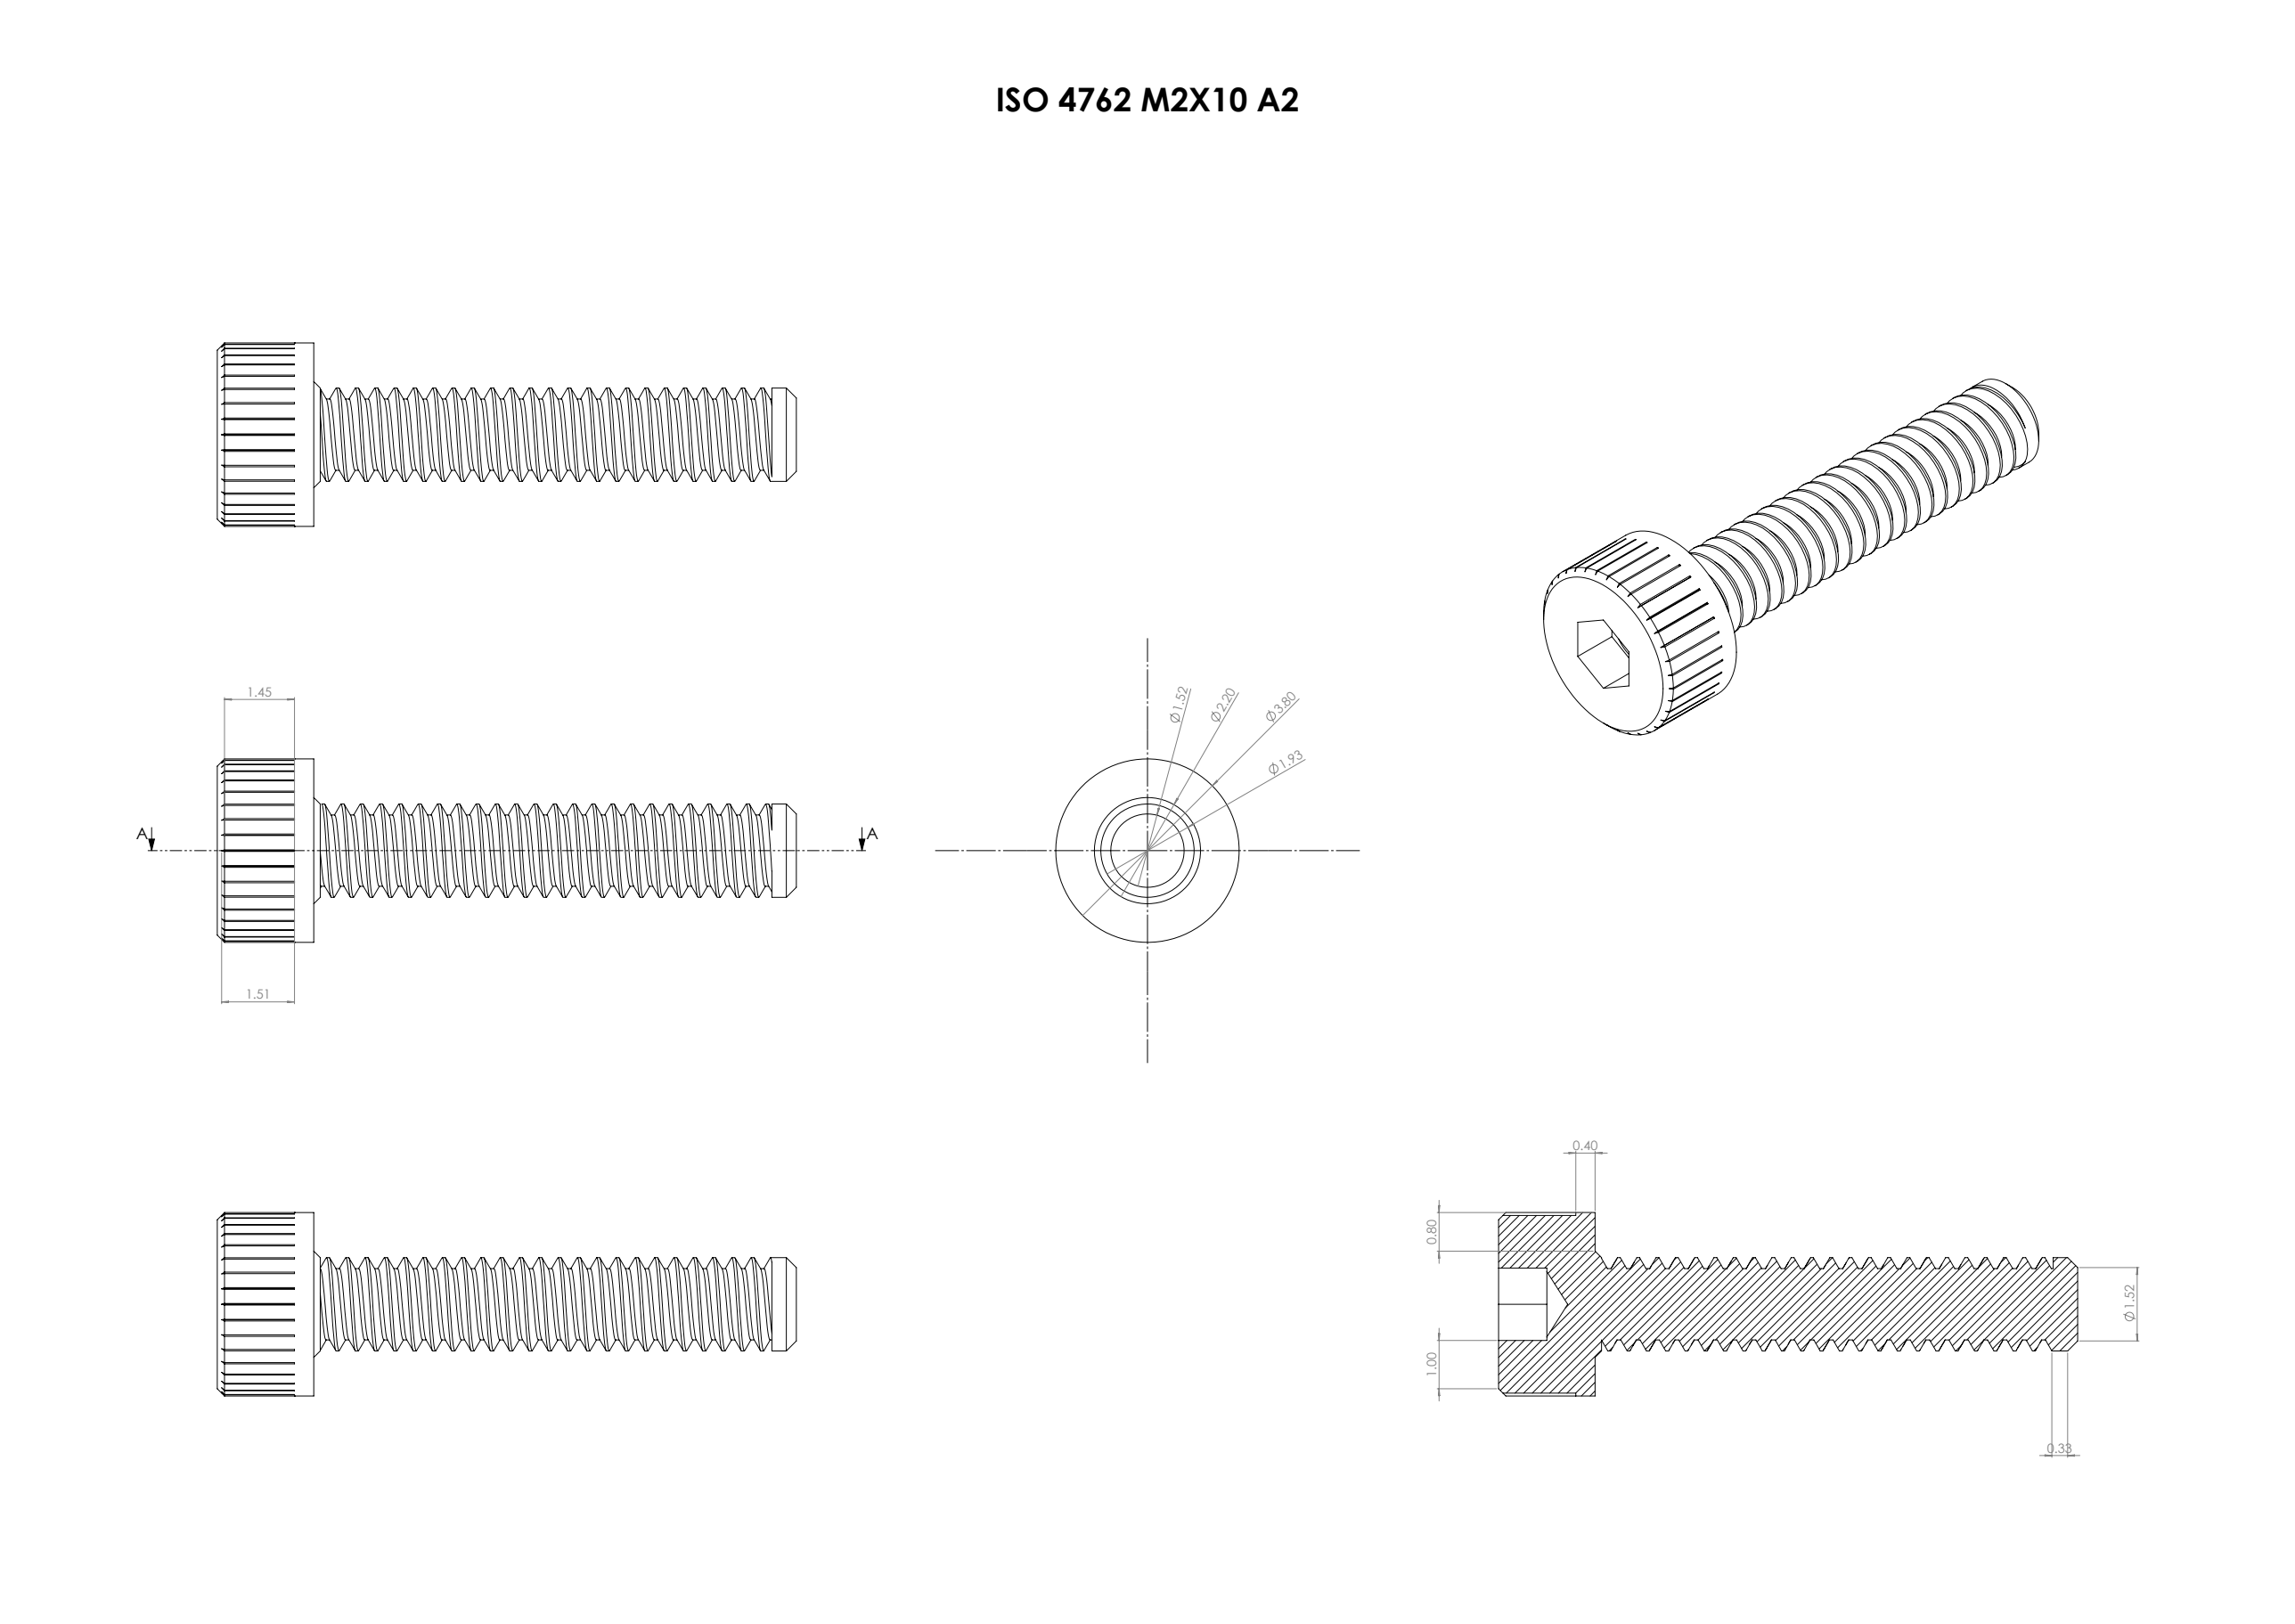
ISO-10303-21;
HEADER;
/* Generated by software containing ST-Developer
 * from STEP Tools, Inc. (www.steptools.com) 
 */

FILE_DESCRIPTION(
/* description */ (''),
/* implementation_level */ '2;1');

FILE_NAME(
/* name */ '16_ISO_4762_M2x10_A2.step',
/* time_stamp */ '2026-10-19T23:00:43-07:00',
/* author */ (''),
/* organization */ (''),
/* preprocessor_version */ 'ST-DEVELOPER v20.2',
/* originating_system */ 'Autodesk Translation Framework v15.15.0.0',
/* authorisation */ '');

FILE_SCHEMA (('AUTOMOTIVE_DESIGN { 1 0 10303 214 3 1 1 }'));
ENDSEC;

DATA;
#10=MECHANICAL_DESIGN_GEOMETRIC_PRESENTATION_REPRESENTATION('',(#1012),#55002);
#323=(
BOUNDED_CURVE()
B_SPLINE_CURVE(2,(#47824,#47825,#47826),.UNSPECIFIED.,.F.,.F.)
B_SPLINE_CURVE_WITH_KNOTS((3,3),(0.,0.00841282944278042),.UNSPECIFIED.)
CURVE()
GEOMETRIC_REPRESENTATION_ITEM()
RATIONAL_B_SPLINE_CURVE((1.,1.00035365746955,1.00043184882983))
REPRESENTATION_ITEM('')
);
#324=(
BOUNDED_CURVE()
B_SPLINE_CURVE(2,(#47830,#47831,#47832),.UNSPECIFIED.,.F.,.F.)
B_SPLINE_CURVE_WITH_KNOTS((3,3),(0.0131888113576721,0.0216016408002996),
 .UNSPECIFIED.)
CURVE()
GEOMETRIC_REPRESENTATION_ITEM()
RATIONAL_B_SPLINE_CURVE((1.00043184882948,1.00035365746926,1.))
REPRESENTATION_ITEM('')
);
#325=(
BOUNDED_CURVE()
B_SPLINE_CURVE(2,(#47845,#47846,#47847),.UNSPECIFIED.,.F.,.F.)
B_SPLINE_CURVE_WITH_KNOTS((3,3),(0.,0.0084128294426201),.UNSPECIFIED.)
CURVE()
GEOMETRIC_REPRESENTATION_ITEM()
RATIONAL_B_SPLINE_CURVE((1.,1.00035365746986,1.00043184883023))
REPRESENTATION_ITEM('')
);
#326=(
BOUNDED_CURVE()
B_SPLINE_CURVE(2,(#47851,#47852,#47853),.UNSPECIFIED.,.F.,.F.)
B_SPLINE_CURVE_WITH_KNOTS((3,3),(0.0131888113575809,0.0216016408002996),
 .UNSPECIFIED.)
CURVE()
GEOMETRIC_REPRESENTATION_ITEM()
RATIONAL_B_SPLINE_CURVE((1.00043184883059,1.00035365747017,1.))
REPRESENTATION_ITEM('')
);
#327=(
BOUNDED_CURVE()
B_SPLINE_CURVE(2,(#47866,#47867,#47868),.UNSPECIFIED.,.F.,.F.)
B_SPLINE_CURVE_WITH_KNOTS((3,3),(0.,0.00841282944278058),.UNSPECIFIED.)
CURVE()
GEOMETRIC_REPRESENTATION_ITEM()
RATIONAL_B_SPLINE_CURVE((1.,1.00035365746906,1.00043184882924))
REPRESENTATION_ITEM('')
);
#328=(
BOUNDED_CURVE()
B_SPLINE_CURVE(2,(#47872,#47873,#47874),.UNSPECIFIED.,.F.,.F.)
B_SPLINE_CURVE_WITH_KNOTS((3,3),(0.0131888113576548,0.0216016408002996),
 .UNSPECIFIED.)
CURVE()
GEOMETRIC_REPRESENTATION_ITEM()
RATIONAL_B_SPLINE_CURVE((1.00043184882846,1.00035365746842,1.))
REPRESENTATION_ITEM('')
);
#329=(
BOUNDED_CURVE()
B_SPLINE_CURVE(2,(#47887,#47888,#47889),.UNSPECIFIED.,.F.,.F.)
B_SPLINE_CURVE_WITH_KNOTS((3,3),(0.,0.00841282944280584),.UNSPECIFIED.)
CURVE()
GEOMETRIC_REPRESENTATION_ITEM()
RATIONAL_B_SPLINE_CURVE((1.,1.00035365746775,1.00043184882763))
REPRESENTATION_ITEM('')
);
#330=(
BOUNDED_CURVE()
B_SPLINE_CURVE(2,(#47893,#47894,#47895),.UNSPECIFIED.,.F.,.F.)
B_SPLINE_CURVE_WITH_KNOTS((3,3),(0.0131888113576015,0.0216016408002996),
 .UNSPECIFIED.)
CURVE()
GEOMETRIC_REPRESENTATION_ITEM()
RATIONAL_B_SPLINE_CURVE((1.00043184882681,1.00035365746707,1.))
REPRESENTATION_ITEM('')
);
#331=(
BOUNDED_CURVE()
B_SPLINE_CURVE(2,(#47908,#47909,#47910),.UNSPECIFIED.,.F.,.F.)
B_SPLINE_CURVE_WITH_KNOTS((3,3),(0.,0.00841282944278488),.UNSPECIFIED.)
CURVE()
GEOMETRIC_REPRESENTATION_ITEM()
RATIONAL_B_SPLINE_CURVE((1.,1.0003536574676,1.00043184882745))
REPRESENTATION_ITEM('')
);
#332=(
BOUNDED_CURVE()
B_SPLINE_CURVE(2,(#47914,#47915,#47916),.UNSPECIFIED.,.F.,.F.)
B_SPLINE_CURVE_WITH_KNOTS((3,3),(0.0131888113575949,0.0216016408002996),
 .UNSPECIFIED.)
CURVE()
GEOMETRIC_REPRESENTATION_ITEM()
RATIONAL_B_SPLINE_CURVE((1.000431848828,1.00035365746804,1.))
REPRESENTATION_ITEM('')
);
#333=(
BOUNDED_CURVE()
B_SPLINE_CURVE(2,(#47929,#47930,#47931),.UNSPECIFIED.,.F.,.F.)
B_SPLINE_CURVE_WITH_KNOTS((3,3),(0.,0.00841282944265237),.UNSPECIFIED.)
CURVE()
GEOMETRIC_REPRESENTATION_ITEM()
RATIONAL_B_SPLINE_CURVE((1.,1.00035365746874,1.00043184882885))
REPRESENTATION_ITEM('')
);
#334=(
BOUNDED_CURVE()
B_SPLINE_CURVE(2,(#47935,#47936,#47937),.UNSPECIFIED.,.F.,.F.)
B_SPLINE_CURVE_WITH_KNOTS((3,3),(0.0131888113575151,0.0216016408002996),
 .UNSPECIFIED.)
CURVE()
GEOMETRIC_REPRESENTATION_ITEM()
RATIONAL_B_SPLINE_CURVE((1.00043184882745,1.0003536574676,1.))
REPRESENTATION_ITEM('')
);
#335=(
BOUNDED_CURVE()
B_SPLINE_CURVE(2,(#47950,#47951,#47952),.UNSPECIFIED.,.F.,.F.)
B_SPLINE_CURVE_WITH_KNOTS((3,3),(0.,0.00841282944265245),.UNSPECIFIED.)
CURVE()
GEOMETRIC_REPRESENTATION_ITEM()
RATIONAL_B_SPLINE_CURVE((1.,1.00035365746621,1.00043184882576))
REPRESENTATION_ITEM('')
);
#336=(
BOUNDED_CURVE()
B_SPLINE_CURVE(2,(#47956,#47957,#47958),.UNSPECIFIED.,.F.,.F.)
B_SPLINE_CURVE_WITH_KNOTS((3,3),(0.013188811357676,0.0216016408002996),
 .UNSPECIFIED.)
CURVE()
GEOMETRIC_REPRESENTATION_ITEM()
RATIONAL_B_SPLINE_CURVE((1.00043184882966,1.0003536574694,1.))
REPRESENTATION_ITEM('')
);
#337=(
BOUNDED_CURVE()
B_SPLINE_CURVE(2,(#47971,#47972,#47973),.UNSPECIFIED.,.F.,.F.)
B_SPLINE_CURVE_WITH_KNOTS((3,3),(0.,0.00841282944263587),.UNSPECIFIED.)
CURVE()
GEOMETRIC_REPRESENTATION_ITEM()
RATIONAL_B_SPLINE_CURVE((1.,1.00035365746699,1.00043184882672))
REPRESENTATION_ITEM('')
);
#338=(
BOUNDED_CURVE()
B_SPLINE_CURVE(2,(#47977,#47978,#47979),.UNSPECIFIED.,.F.,.F.)
B_SPLINE_CURVE_WITH_KNOTS((3,3),(0.0131888113575321,0.0216016408002996),
 .UNSPECIFIED.)
CURVE()
GEOMETRIC_REPRESENTATION_ITEM()
RATIONAL_B_SPLINE_CURVE((1.00043184883015,1.00035365746981,1.))
REPRESENTATION_ITEM('')
);
#339=(
BOUNDED_CURVE()
B_SPLINE_CURVE(2,(#47992,#47993,#47994),.UNSPECIFIED.,.F.,.F.)
B_SPLINE_CURVE_WITH_KNOTS((3,3),(0.,0.00841282944268715),.UNSPECIFIED.)
CURVE()
GEOMETRIC_REPRESENTATION_ITEM()
RATIONAL_B_SPLINE_CURVE((1.,1.00035365746714,1.0004318488269))
REPRESENTATION_ITEM('')
);
#340=(
BOUNDED_CURVE()
B_SPLINE_CURVE(2,(#47998,#47999,#48000),.UNSPECIFIED.,.F.,.F.)
B_SPLINE_CURVE_WITH_KNOTS((3,3),(0.0131888113576173,0.0216016408002996),
 .UNSPECIFIED.)
CURVE()
GEOMETRIC_REPRESENTATION_ITEM()
RATIONAL_B_SPLINE_CURVE((1.00043184882651,1.00035365746683,1.))
REPRESENTATION_ITEM('')
);
#341=(
BOUNDED_CURVE()
B_SPLINE_CURVE(2,(#48013,#48014,#48015),.UNSPECIFIED.,.F.,.F.)
B_SPLINE_CURVE_WITH_KNOTS((3,3),(0.,0.00841282944268232),.UNSPECIFIED.)
CURVE()
GEOMETRIC_REPRESENTATION_ITEM()
RATIONAL_B_SPLINE_CURVE((1.,1.00035365746714,1.0004318488269))
REPRESENTATION_ITEM('')
);
#342=(
BOUNDED_CURVE()
B_SPLINE_CURVE(2,(#48019,#48020,#48021),.UNSPECIFIED.,.F.,.F.)
B_SPLINE_CURVE_WITH_KNOTS((3,3),(0.0131888113576523,0.0216016408002997),
 .UNSPECIFIED.)
CURVE()
GEOMETRIC_REPRESENTATION_ITEM()
RATIONAL_B_SPLINE_CURVE((1.00043184882641,1.00035365746674,1.))
REPRESENTATION_ITEM('')
);
#343=(
BOUNDED_CURVE()
B_SPLINE_CURVE(2,(#48034,#48035,#48036),.UNSPECIFIED.,.F.,.F.)
B_SPLINE_CURVE_WITH_KNOTS((3,3),(0.,0.00841282944262782),.UNSPECIFIED.)
CURVE()
GEOMETRIC_REPRESENTATION_ITEM()
RATIONAL_B_SPLINE_CURVE((1.,1.00035365747069,1.00043184883123))
REPRESENTATION_ITEM('')
);
#344=(
BOUNDED_CURVE()
B_SPLINE_CURVE(2,(#48040,#48041,#48042),.UNSPECIFIED.,.F.,.F.)
B_SPLINE_CURVE_WITH_KNOTS((3,3),(0.0131888113575803,0.0216016408002996),
 .UNSPECIFIED.)
CURVE()
GEOMETRIC_REPRESENTATION_ITEM()
RATIONAL_B_SPLINE_CURVE((1.00043184883154,1.00035365747094,1.))
REPRESENTATION_ITEM('')
);
#345=(
BOUNDED_CURVE()
B_SPLINE_CURVE(2,(#48055,#48056,#48057),.UNSPECIFIED.,.F.,.F.)
B_SPLINE_CURVE_WITH_KNOTS((3,3),(0.,0.00841282944278058),.UNSPECIFIED.)
CURVE()
GEOMETRIC_REPRESENTATION_ITEM()
RATIONAL_B_SPLINE_CURVE((1.,1.00035365746906,1.00043184882924))
REPRESENTATION_ITEM('')
);
#346=(
BOUNDED_CURVE()
B_SPLINE_CURVE(2,(#48061,#48062,#48063),.UNSPECIFIED.,.F.,.F.)
B_SPLINE_CURVE_WITH_KNOTS((3,3),(0.0131888113576548,0.0216016408002996),
 .UNSPECIFIED.)
CURVE()
GEOMETRIC_REPRESENTATION_ITEM()
RATIONAL_B_SPLINE_CURVE((1.00043184882846,1.00035365746842,1.))
REPRESENTATION_ITEM('')
);
#347=(
BOUNDED_CURVE()
B_SPLINE_CURVE(2,(#48076,#48077,#48078),.UNSPECIFIED.,.F.,.F.)
B_SPLINE_CURVE_WITH_KNOTS((3,3),(0.,0.00841282944280138),.UNSPECIFIED.)
CURVE()
GEOMETRIC_REPRESENTATION_ITEM()
RATIONAL_B_SPLINE_CURVE((1.,1.00035365746471,1.00043184882392))
REPRESENTATION_ITEM('')
);
#348=(
BOUNDED_CURVE()
B_SPLINE_CURVE(2,(#48082,#48083,#48084),.UNSPECIFIED.,.F.,.F.)
B_SPLINE_CURVE_WITH_KNOTS((3,3),(0.0131888113575931,0.0216016408002996),
 .UNSPECIFIED.)
CURVE()
GEOMETRIC_REPRESENTATION_ITEM()
RATIONAL_B_SPLINE_CURVE((1.00043184882494,1.00035365746554,1.))
REPRESENTATION_ITEM('')
);
#349=(
BOUNDED_CURVE()
B_SPLINE_CURVE(2,(#48097,#48098,#48099),.UNSPECIFIED.,.F.,.F.)
B_SPLINE_CURVE_WITH_KNOTS((3,3),(0.,0.00841282944261464),.UNSPECIFIED.)
CURVE()
GEOMETRIC_REPRESENTATION_ITEM()
RATIONAL_B_SPLINE_CURVE((1.,1.00035365746679,1.00043184882648))
REPRESENTATION_ITEM('')
);
#350=(
BOUNDED_CURVE()
B_SPLINE_CURVE(2,(#48103,#48104,#48105),.UNSPECIFIED.,.F.,.F.)
B_SPLINE_CURVE_WITH_KNOTS((3,3),(0.0131888113575887,0.0216016408002996),
 .UNSPECIFIED.)
CURVE()
GEOMETRIC_REPRESENTATION_ITEM()
RATIONAL_B_SPLINE_CURVE((1.00043184882758,1.0003536574677,1.))
REPRESENTATION_ITEM('')
);
#351=(
BOUNDED_CURVE()
B_SPLINE_CURVE(2,(#48118,#48119,#48120),.UNSPECIFIED.,.F.,.F.)
B_SPLINE_CURVE_WITH_KNOTS((3,3),(0.,0.00841282944265251),.UNSPECIFIED.)
CURVE()
GEOMETRIC_REPRESENTATION_ITEM()
RATIONAL_B_SPLINE_CURVE((1.,1.00035365746762,1.00043184882748))
REPRESENTATION_ITEM('')
);
#352=(
BOUNDED_CURVE()
B_SPLINE_CURVE(2,(#48124,#48125,#48126),.UNSPECIFIED.,.F.,.F.)
B_SPLINE_CURVE_WITH_KNOTS((3,3),(0.0131888113576473,0.0216016408002996),
 .UNSPECIFIED.)
CURVE()
GEOMETRIC_REPRESENTATION_ITEM()
RATIONAL_B_SPLINE_CURVE((1.00043184883165,1.00035365747103,1.))
REPRESENTATION_ITEM('')
);
#353=(
BOUNDED_CURVE()
B_SPLINE_CURVE(2,(#48139,#48140,#48141),.UNSPECIFIED.,.F.,.F.)
B_SPLINE_CURVE_WITH_KNOTS((3,3),(0.,0.00841282944262983),.UNSPECIFIED.)
CURVE()
GEOMETRIC_REPRESENTATION_ITEM()
RATIONAL_B_SPLINE_CURVE((1.,1.00035365747139,1.00043184883209))
REPRESENTATION_ITEM('')
);
#354=(
BOUNDED_CURVE()
B_SPLINE_CURVE(2,(#48145,#48146,#48147),.UNSPECIFIED.,.F.,.F.)
B_SPLINE_CURVE_WITH_KNOTS((3,3),(0.0131888113576388,0.0216016408002996),
 .UNSPECIFIED.)
CURVE()
GEOMETRIC_REPRESENTATION_ITEM()
RATIONAL_B_SPLINE_CURVE((1.00043184882737,1.00035365746753,1.))
REPRESENTATION_ITEM('')
);
#355=(
BOUNDED_CURVE()
B_SPLINE_CURVE(2,(#48160,#48161,#48162),.UNSPECIFIED.,.F.,.F.)
B_SPLINE_CURVE_WITH_KNOTS((3,3),(0.,0.00841282944261306),.UNSPECIFIED.)
CURVE()
GEOMETRIC_REPRESENTATION_ITEM()
RATIONAL_B_SPLINE_CURVE((1.,1.00035365747318,1.00043184883428))
REPRESENTATION_ITEM('')
);
#356=(
BOUNDED_CURVE()
B_SPLINE_CURVE(2,(#48166,#48167,#48168),.UNSPECIFIED.,.F.,.F.)
B_SPLINE_CURVE_WITH_KNOTS((3,3),(0.0131888113575341,0.0216016408002996),
 .UNSPECIFIED.)
CURVE()
GEOMETRIC_REPRESENTATION_ITEM()
RATIONAL_B_SPLINE_CURVE((1.00043184882813,1.00035365746816,1.))
REPRESENTATION_ITEM('')
);
#357=(
BOUNDED_CURVE()
B_SPLINE_CURVE(2,(#48183,#48184,#48185),.UNSPECIFIED.,.F.,.F.)
B_SPLINE_CURVE_WITH_KNOTS((3,3),(0.,0.00841282944268199),.UNSPECIFIED.)
CURVE()
GEOMETRIC_REPRESENTATION_ITEM()
RATIONAL_B_SPLINE_CURVE((1.,1.00035365746877,1.00043184882888))
REPRESENTATION_ITEM('')
);
#358=(
BOUNDED_CURVE()
B_SPLINE_CURVE(2,(#48189,#48190,#48191),.UNSPECIFIED.,.F.,.F.)
B_SPLINE_CURVE_WITH_KNOTS((3,3),(0.0131888113576103,0.0216016408002996),
 .UNSPECIFIED.)
CURVE()
GEOMETRIC_REPRESENTATION_ITEM()
RATIONAL_B_SPLINE_CURVE((1.00043184882915,1.00035365746898,1.))
REPRESENTATION_ITEM('')
);
#359=(
BOUNDED_CURVE()
B_SPLINE_CURVE(2,(#48204,#48205,#48206),.UNSPECIFIED.,.F.,.F.)
B_SPLINE_CURVE_WITH_KNOTS((3,3),(0.,0.00841282944276111),.UNSPECIFIED.)
CURVE()
GEOMETRIC_REPRESENTATION_ITEM()
RATIONAL_B_SPLINE_CURVE((1.,1.00035365746789,1.00043184882782))
REPRESENTATION_ITEM('')
);
#360=(
BOUNDED_CURVE()
B_SPLINE_CURVE(2,(#48210,#48211,#48212),.UNSPECIFIED.,.F.,.F.)
B_SPLINE_CURVE_WITH_KNOTS((3,3),(0.013188811357663,0.0216016408002997),
 .UNSPECIFIED.)
CURVE()
GEOMETRIC_REPRESENTATION_ITEM()
RATIONAL_B_SPLINE_CURVE((1.00043184882852,1.00035365746847,1.))
REPRESENTATION_ITEM('')
);
#361=(
BOUNDED_CURVE()
B_SPLINE_CURVE(2,(#48225,#48226,#48227),.UNSPECIFIED.,.F.,.F.)
B_SPLINE_CURVE_WITH_KNOTS((3,3),(0.,0.00841282944263208),.UNSPECIFIED.)
CURVE()
GEOMETRIC_REPRESENTATION_ITEM()
RATIONAL_B_SPLINE_CURVE((1.,1.00035365746816,1.00043184882815))
REPRESENTATION_ITEM('')
);
#362=(
BOUNDED_CURVE()
B_SPLINE_CURVE(2,(#48231,#48232,#48233),.UNSPECIFIED.,.F.,.F.)
B_SPLINE_CURVE_WITH_KNOTS((3,3),(0.013188811357748,0.0216016408002996),
 .UNSPECIFIED.)
CURVE()
GEOMETRIC_REPRESENTATION_ITEM()
RATIONAL_B_SPLINE_CURVE((1.00043184883132,1.00035365747076,1.))
REPRESENTATION_ITEM('')
);
#363=(
BOUNDED_CURVE()
B_SPLINE_CURVE(2,(#48246,#48247,#48248),.UNSPECIFIED.,.F.,.F.)
B_SPLINE_CURVE_WITH_KNOTS((3,3),(0.,0.00841282944264326),.UNSPECIFIED.)
CURVE()
GEOMETRIC_REPRESENTATION_ITEM()
RATIONAL_B_SPLINE_CURVE((1.,1.00035365746759,1.00043184882744))
REPRESENTATION_ITEM('')
);
#364=(
BOUNDED_CURVE()
B_SPLINE_CURVE(2,(#48252,#48253,#48254),.UNSPECIFIED.,.F.,.F.)
B_SPLINE_CURVE_WITH_KNOTS((3,3),(0.0131888113575487,0.0216016408002996),
 .UNSPECIFIED.)
CURVE()
GEOMETRIC_REPRESENTATION_ITEM()
RATIONAL_B_SPLINE_CURVE((1.0004318488259,1.00035365746632,1.))
REPRESENTATION_ITEM('')
);
#365=(
BOUNDED_CURVE()
B_SPLINE_CURVE(2,(#48267,#48268,#48269),.UNSPECIFIED.,.F.,.F.)
B_SPLINE_CURVE_WITH_KNOTS((3,3),(0.,0.00841282944280138),.UNSPECIFIED.)
CURVE()
GEOMETRIC_REPRESENTATION_ITEM()
RATIONAL_B_SPLINE_CURVE((1.,1.00035365746471,1.00043184882392))
REPRESENTATION_ITEM('')
);
#366=(
BOUNDED_CURVE()
B_SPLINE_CURVE(2,(#48273,#48274,#48275),.UNSPECIFIED.,.F.,.F.)
B_SPLINE_CURVE_WITH_KNOTS((3,3),(0.0131888113575931,0.0216016408002996),
 .UNSPECIFIED.)
CURVE()
GEOMETRIC_REPRESENTATION_ITEM()
RATIONAL_B_SPLINE_CURVE((1.00043184882494,1.00035365746554,1.))
REPRESENTATION_ITEM('')
);
#367=(
BOUNDED_CURVE()
B_SPLINE_CURVE(2,(#48288,#48289,#48290),.UNSPECIFIED.,.F.,.F.)
B_SPLINE_CURVE_WITH_KNOTS((3,3),(0.,0.00841282944270105),.UNSPECIFIED.)
CURVE()
GEOMETRIC_REPRESENTATION_ITEM()
RATIONAL_B_SPLINE_CURVE((1.,1.000353657467,1.00043184882673))
REPRESENTATION_ITEM('')
);
#368=(
BOUNDED_CURVE()
B_SPLINE_CURVE(2,(#48294,#48295,#48296),.UNSPECIFIED.,.F.,.F.)
B_SPLINE_CURVE_WITH_KNOTS((3,3),(0.0131888113574971,0.0216016408002996),
 .UNSPECIFIED.)
CURVE()
GEOMETRIC_REPRESENTATION_ITEM()
RATIONAL_B_SPLINE_CURVE((1.00043184882773,1.00035365746783,1.))
REPRESENTATION_ITEM('')
);
#369=(
BOUNDED_CURVE()
B_SPLINE_CURVE(2,(#48309,#48310,#48311),.UNSPECIFIED.,.F.,.F.)
B_SPLINE_CURVE_WITH_KNOTS((3,3),(0.,0.00841282944264652),.UNSPECIFIED.)
CURVE()
GEOMETRIC_REPRESENTATION_ITEM()
RATIONAL_B_SPLINE_CURVE((1.,1.00035365746972,1.00043184883004))
REPRESENTATION_ITEM('')
);
#370=(
BOUNDED_CURVE()
B_SPLINE_CURVE(2,(#48315,#48316,#48317),.UNSPECIFIED.,.F.,.F.)
B_SPLINE_CURVE_WITH_KNOTS((3,3),(0.0131888113576371,0.0216016408002996),
 .UNSPECIFIED.)
CURVE()
GEOMETRIC_REPRESENTATION_ITEM()
RATIONAL_B_SPLINE_CURVE((1.00043184882659,1.00035365746689,1.))
REPRESENTATION_ITEM('')
);
#371=(
BOUNDED_CURVE()
B_SPLINE_CURVE(2,(#48330,#48331,#48332),.UNSPECIFIED.,.F.,.F.)
B_SPLINE_CURVE_WITH_KNOTS((3,3),(0.,0.00841282944262983),.UNSPECIFIED.)
CURVE()
GEOMETRIC_REPRESENTATION_ITEM()
RATIONAL_B_SPLINE_CURVE((1.,1.00035365747139,1.00043184883209))
REPRESENTATION_ITEM('')
);
#372=(
BOUNDED_CURVE()
B_SPLINE_CURVE(2,(#48336,#48337,#48338),.UNSPECIFIED.,.F.,.F.)
B_SPLINE_CURVE_WITH_KNOTS((3,3),(0.0131888113576388,0.0216016408002996),
 .UNSPECIFIED.)
CURVE()
GEOMETRIC_REPRESENTATION_ITEM()
RATIONAL_B_SPLINE_CURVE((1.00043184882737,1.00035365746753,1.))
REPRESENTATION_ITEM('')
);
#373=(
BOUNDED_CURVE()
B_SPLINE_CURVE(2,(#48351,#48352,#48353),.UNSPECIFIED.,.F.,.F.)
B_SPLINE_CURVE_WITH_KNOTS((3,3),(0.,0.00841282944264003),.UNSPECIFIED.)
CURVE()
GEOMETRIC_REPRESENTATION_ITEM()
RATIONAL_B_SPLINE_CURVE((1.,1.0003536574673,1.00043184882709))
REPRESENTATION_ITEM('')
);
#374=(
BOUNDED_CURVE()
B_SPLINE_CURVE(2,(#48357,#48358,#48359),.UNSPECIFIED.,.F.,.F.)
B_SPLINE_CURVE_WITH_KNOTS((3,3),(0.0131888113576155,0.0216016408002996),
 .UNSPECIFIED.)
CURVE()
GEOMETRIC_REPRESENTATION_ITEM()
RATIONAL_B_SPLINE_CURVE((1.00043184882608,1.00035365746647,1.))
REPRESENTATION_ITEM('')
);
#375=(
BOUNDED_CURVE()
B_SPLINE_CURVE(2,(#48372,#48373,#48374),.UNSPECIFIED.,.F.,.F.)
B_SPLINE_CURVE_WITH_KNOTS((3,3),(0.,0.00841282944269557),.UNSPECIFIED.)
CURVE()
GEOMETRIC_REPRESENTATION_ITEM()
RATIONAL_B_SPLINE_CURVE((1.,1.00035365746722,1.000431848827))
REPRESENTATION_ITEM('')
);
#376=(
BOUNDED_CURVE()
B_SPLINE_CURVE(2,(#48378,#48379,#48380),.UNSPECIFIED.,.F.,.F.)
B_SPLINE_CURVE_WITH_KNOTS((3,3),(0.0131888113576143,0.0216016408002996),
 .UNSPECIFIED.)
CURVE()
GEOMETRIC_REPRESENTATION_ITEM()
RATIONAL_B_SPLINE_CURVE((1.00043184882947,1.00035365746925,1.))
REPRESENTATION_ITEM('')
);
#377=(
BOUNDED_CURVE()
B_SPLINE_CURVE(2,(#48393,#48394,#48395),.UNSPECIFIED.,.F.,.F.)
B_SPLINE_CURVE_WITH_KNOTS((3,3),(0.,0.00841282944278065),.UNSPECIFIED.)
CURVE()
GEOMETRIC_REPRESENTATION_ITEM()
RATIONAL_B_SPLINE_CURVE((1.,1.00035365746947,1.00043184882974))
REPRESENTATION_ITEM('')
);
#378=(
BOUNDED_CURVE()
B_SPLINE_CURVE(2,(#48399,#48400,#48401),.UNSPECIFIED.,.F.,.F.)
B_SPLINE_CURVE_WITH_KNOTS((3,3),(0.0131888113576697,0.0216016408002996),
 .UNSPECIFIED.)
CURVE()
GEOMETRIC_REPRESENTATION_ITEM()
RATIONAL_B_SPLINE_CURVE((1.00043184882899,1.00035365746886,1.))
REPRESENTATION_ITEM('')
);
#379=(
BOUNDED_CURVE()
B_SPLINE_CURVE(2,(#48414,#48415,#48416),.UNSPECIFIED.,.F.,.F.)
B_SPLINE_CURVE_WITH_KNOTS((3,3),(0.,0.00841282944263208),.UNSPECIFIED.)
CURVE()
GEOMETRIC_REPRESENTATION_ITEM()
RATIONAL_B_SPLINE_CURVE((1.,1.00035365746816,1.00043184882815))
REPRESENTATION_ITEM('')
);
#380=(
BOUNDED_CURVE()
B_SPLINE_CURVE(2,(#48420,#48421,#48422),.UNSPECIFIED.,.F.,.F.)
B_SPLINE_CURVE_WITH_KNOTS((3,3),(0.013188811357748,0.0216016408002996),
 .UNSPECIFIED.)
CURVE()
GEOMETRIC_REPRESENTATION_ITEM()
RATIONAL_B_SPLINE_CURVE((1.00043184883132,1.00035365747076,1.))
REPRESENTATION_ITEM('')
);
#381=(
BOUNDED_CURVE()
B_SPLINE_CURVE(2,(#48435,#48436,#48437),.UNSPECIFIED.,.F.,.F.)
B_SPLINE_CURVE_WITH_KNOTS((3,3),(0.,0.00841282944273455),.UNSPECIFIED.)
CURVE()
GEOMETRIC_REPRESENTATION_ITEM()
RATIONAL_B_SPLINE_CURVE((1.,1.00035365746539,1.00043184882476))
REPRESENTATION_ITEM('')
);
#382=(
BOUNDED_CURVE()
B_SPLINE_CURVE(2,(#48441,#48442,#48443),.UNSPECIFIED.,.F.,.F.)
B_SPLINE_CURVE_WITH_KNOTS((3,3),(0.0131888113576539,0.0216016408002996),
 .UNSPECIFIED.)
CURVE()
GEOMETRIC_REPRESENTATION_ITEM()
RATIONAL_B_SPLINE_CURVE((1.00043184882929,1.0003536574691,1.))
REPRESENTATION_ITEM('')
);
#383=(
BOUNDED_CURVE()
B_SPLINE_CURVE(2,(#48456,#48457,#48458),.UNSPECIFIED.,.F.,.F.)
B_SPLINE_CURVE_WITH_KNOTS((3,3),(0.,0.00841282944270133),.UNSPECIFIED.)
CURVE()
GEOMETRIC_REPRESENTATION_ITEM()
RATIONAL_B_SPLINE_CURVE((1.,1.00035365747008,1.00043184883048))
REPRESENTATION_ITEM('')
);
#384=(
BOUNDED_CURVE()
B_SPLINE_CURVE(2,(#48462,#48463,#48464),.UNSPECIFIED.,.F.,.F.)
B_SPLINE_CURVE_WITH_KNOTS((3,3),(0.0131888113576197,0.0216016408002996),
 .UNSPECIFIED.)
CURVE()
GEOMETRIC_REPRESENTATION_ITEM()
RATIONAL_B_SPLINE_CURVE((1.00043184882798,1.00035365746803,1.))
REPRESENTATION_ITEM('')
);
#385=(
BOUNDED_CURVE()
B_SPLINE_CURVE(2,(#48477,#48478,#48479),.UNSPECIFIED.,.F.,.F.)
B_SPLINE_CURVE_WITH_KNOTS((3,3),(0.,0.00841282944261464),.UNSPECIFIED.)
CURVE()
GEOMETRIC_REPRESENTATION_ITEM()
RATIONAL_B_SPLINE_CURVE((1.,1.00035365746679,1.00043184882648))
REPRESENTATION_ITEM('')
);
#386=(
BOUNDED_CURVE()
B_SPLINE_CURVE(2,(#48483,#48484,#48485),.UNSPECIFIED.,.F.,.F.)
B_SPLINE_CURVE_WITH_KNOTS((3,3),(0.0131888113575887,0.0216016408002996),
 .UNSPECIFIED.)
CURVE()
GEOMETRIC_REPRESENTATION_ITEM()
RATIONAL_B_SPLINE_CURVE((1.00043184882758,1.0003536574677,1.))
REPRESENTATION_ITEM('')
);
#387=(
BOUNDED_CURVE()
B_SPLINE_CURVE(2,(#48498,#48499,#48500),.UNSPECIFIED.,.F.,.F.)
B_SPLINE_CURVE_WITH_KNOTS((3,3),(0.,0.00841282944264924),.UNSPECIFIED.)
CURVE()
GEOMETRIC_REPRESENTATION_ITEM()
RATIONAL_B_SPLINE_CURVE((1.,1.00035365746952,1.00043184882981))
REPRESENTATION_ITEM('')
);
#388=(
BOUNDED_CURVE()
B_SPLINE_CURVE(2,(#48504,#48505,#48506),.UNSPECIFIED.,.F.,.F.)
B_SPLINE_CURVE_WITH_KNOTS((3,3),(0.0131888113576407,0.0216016408002996),
 .UNSPECIFIED.)
CURVE()
GEOMETRIC_REPRESENTATION_ITEM()
RATIONAL_B_SPLINE_CURVE((1.00043184882821,1.00035365746821,1.))
REPRESENTATION_ITEM('')
);
#389=(
BOUNDED_CURVE()
B_SPLINE_CURVE(2,(#48519,#48520,#48521),.UNSPECIFIED.,.F.,.F.)
B_SPLINE_CURVE_WITH_KNOTS((3,3),(0.,0.00841282944262983),.UNSPECIFIED.)
CURVE()
GEOMETRIC_REPRESENTATION_ITEM()
RATIONAL_B_SPLINE_CURVE((1.,1.00035365747139,1.00043184883209))
REPRESENTATION_ITEM('')
);
#390=(
BOUNDED_CURVE()
B_SPLINE_CURVE(2,(#48525,#48526,#48527),.UNSPECIFIED.,.F.,.F.)
B_SPLINE_CURVE_WITH_KNOTS((3,3),(0.0131888113576388,0.0216016408002996),
 .UNSPECIFIED.)
CURVE()
GEOMETRIC_REPRESENTATION_ITEM()
RATIONAL_B_SPLINE_CURVE((1.00043184882737,1.00035365746753,1.))
REPRESENTATION_ITEM('')
);
#391=(
BOUNDED_CURVE()
B_SPLINE_CURVE(2,(#48540,#48541,#48542),.UNSPECIFIED.,.F.,.F.)
B_SPLINE_CURVE_WITH_KNOTS((3,3),(0.,0.0084128294426321),.UNSPECIFIED.)
CURVE()
GEOMETRIC_REPRESENTATION_ITEM()
RATIONAL_B_SPLINE_CURVE((1.,1.00035365746883,1.00043184882896))
REPRESENTATION_ITEM('')
);
#392=(
BOUNDED_CURVE()
B_SPLINE_CURVE(2,(#48546,#48547,#48548),.UNSPECIFIED.,.F.,.F.)
B_SPLINE_CURVE_WITH_KNOTS((3,3),(0.0131888113575073,0.0216016408002996),
 .UNSPECIFIED.)
CURVE()
GEOMETRIC_REPRESENTATION_ITEM()
RATIONAL_B_SPLINE_CURVE((1.00043184882395,1.00035365746473,1.))
REPRESENTATION_ITEM('')
);
#393=(
BOUNDED_CURVE()
B_SPLINE_CURVE(2,(#48601,#48602,#48603),.UNSPECIFIED.,.F.,.F.)
B_SPLINE_CURVE_WITH_KNOTS((3,3),(0.,0.00841282944285724),.UNSPECIFIED.)
CURVE()
GEOMETRIC_REPRESENTATION_ITEM()
RATIONAL_B_SPLINE_CURVE((1.,1.00035365746964,1.00043184882994))
REPRESENTATION_ITEM('')
);
#394=(
BOUNDED_CURVE()
B_SPLINE_CURVE(2,(#48605,#48606,#48607),.UNSPECIFIED.,.F.,.F.)
B_SPLINE_CURVE_WITH_KNOTS((3,3),(0.0131888113574265,0.0216016408002996),
 .UNSPECIFIED.)
CURVE()
GEOMETRIC_REPRESENTATION_ITEM()
RATIONAL_B_SPLINE_CURVE((1.00043184882266,1.00035365746368,1.))
REPRESENTATION_ITEM('')
);
#476=B_SPLINE_SURFACE_WITH_KNOTS('',3,3,((#46447,#46448,#46449,#46450,#46451,
#46452,#46453,#46454,#46455,#46456,#46457,#46458,#46459,#46460,#46461,#46462,
#46463,#46464,#46465,#46466,#46467,#46468,#46469,#46470,#46471,#46472,#46473,
#46474,#46475,#46476,#46477,#46478,#46479,#46480,#46481,#46482,#46483,#46484,
#46485,#46486,#46487,#46488,#46489,#46490,#46491,#46492,#46493,#46494,#46495,
#46496,#46497,#46498,#46499,#46500,#46501,#46502,#46503,#46504,#46505,#46506,
#46507,#46508,#46509,#46510,#46511,#46512,#46513,#46514,#46515,#46516,#46517,
#46518,#46519,#46520,#46521,#46522,#46523,#46524,#46525,#46526,#46527,#46528,
#46529,#46530,#46531,#46532,#46533,#46534,#46535,#46536,#46537,#46538,#46539,
#46540,#46541,#46542,#46543,#46544,#46545,#46546,#46547,#46548,#46549,#46550,
#46551,#46552,#46553,#46554,#46555,#46556,#46557,#46558,#46559,#46560,#46561,
#46562,#46563,#46564,#46565,#46566,#46567,#46568,#46569,#46570,#46571,#46572,
#46573,#46574,#46575,#46576,#46577,#46578,#46579,#46580,#46581,#46582,#46583,
#46584,#46585,#46586,#46587,#46588,#46589,#46590,#46591,#46592,#46593,#46594,
#46595,#46596,#46597,#46598,#46599),(#46600,#46601,#46602,#46603,#46604,
#46605,#46606,#46607,#46608,#46609,#46610,#46611,#46612,#46613,#46614,#46615,
#46616,#46617,#46618,#46619,#46620,#46621,#46622,#46623,#46624,#46625,#46626,
#46627,#46628,#46629,#46630,#46631,#46632,#46633,#46634,#46635,#46636,#46637,
#46638,#46639,#46640,#46641,#46642,#46643,#46644,#46645,#46646,#46647,#46648,
#46649,#46650,#46651,#46652,#46653,#46654,#46655,#46656,#46657,#46658,#46659,
#46660,#46661,#46662,#46663,#46664,#46665,#46666,#46667,#46668,#46669,#46670,
#46671,#46672,#46673,#46674,#46675,#46676,#46677,#46678,#46679,#46680,#46681,
#46682,#46683,#46684,#46685,#46686,#46687,#46688,#46689,#46690,#46691,#46692,
#46693,#46694,#46695,#46696,#46697,#46698,#46699,#46700,#46701,#46702,#46703,
#46704,#46705,#46706,#46707,#46708,#46709,#46710,#46711,#46712,#46713,#46714,
#46715,#46716,#46717,#46718,#46719,#46720,#46721,#46722,#46723,#46724,#46725,
#46726,#46727,#46728,#46729,#46730,#46731,#46732,#46733,#46734,#46735,#46736,
#46737,#46738,#46739,#46740,#46741,#46742,#46743,#46744,#46745,#46746,#46747,
#46748,#46749,#46750,#46751,#46752),(#46753,#46754,#46755,#46756,#46757,
#46758,#46759,#46760,#46761,#46762,#46763,#46764,#46765,#46766,#46767,#46768,
#46769,#46770,#46771,#46772,#46773,#46774,#46775,#46776,#46777,#46778,#46779,
#46780,#46781,#46782,#46783,#46784,#46785,#46786,#46787,#46788,#46789,#46790,
#46791,#46792,#46793,#46794,#46795,#46796,#46797,#46798,#46799,#46800,#46801,
#46802,#46803,#46804,#46805,#46806,#46807,#46808,#46809,#46810,#46811,#46812,
#46813,#46814,#46815,#46816,#46817,#46818,#46819,#46820,#46821,#46822,#46823,
#46824,#46825,#46826,#46827,#46828,#46829,#46830,#46831,#46832,#46833,#46834,
#46835,#46836,#46837,#46838,#46839,#46840,#46841,#46842,#46843,#46844,#46845,
#46846,#46847,#46848,#46849,#46850,#46851,#46852,#46853,#46854,#46855,#46856,
#46857,#46858,#46859,#46860,#46861,#46862,#46863,#46864,#46865,#46866,#46867,
#46868,#46869,#46870,#46871,#46872,#46873,#46874,#46875,#46876,#46877,#46878,
#46879,#46880,#46881,#46882,#46883,#46884,#46885,#46886,#46887,#46888,#46889,
#46890,#46891,#46892,#46893,#46894,#46895,#46896,#46897,#46898,#46899,#46900,
#46901,#46902,#46903,#46904,#46905),(#46906,#46907,#46908,#46909,#46910,
#46911,#46912,#46913,#46914,#46915,#46916,#46917,#46918,#46919,#46920,#46921,
#46922,#46923,#46924,#46925,#46926,#46927,#46928,#46929,#46930,#46931,#46932,
#46933,#46934,#46935,#46936,#46937,#46938,#46939,#46940,#46941,#46942,#46943,
#46944,#46945,#46946,#46947,#46948,#46949,#46950,#46951,#46952,#46953,#46954,
#46955,#46956,#46957,#46958,#46959,#46960,#46961,#46962,#46963,#46964,#46965,
#46966,#46967,#46968,#46969,#46970,#46971,#46972,#46973,#46974,#46975,#46976,
#46977,#46978,#46979,#46980,#46981,#46982,#46983,#46984,#46985,#46986,#46987,
#46988,#46989,#46990,#46991,#46992,#46993,#46994,#46995,#46996,#46997,#46998,
#46999,#47000,#47001,#47002,#47003,#47004,#47005,#47006,#47007,#47008,#47009,
#47010,#47011,#47012,#47013,#47014,#47015,#47016,#47017,#47018,#47019,#47020,
#47021,#47022,#47023,#47024,#47025,#47026,#47027,#47028,#47029,#47030,#47031,
#47032,#47033,#47034,#47035,#47036,#47037,#47038,#47039,#47040,#47041,#47042,
#47043,#47044,#47045,#47046,#47047,#47048,#47049,#47050,#47051,#47052,#47053,
#47054,#47055,#47056,#47057,#47058)),.UNSPECIFIED.,.F.,.F.,.F.,(4,4),(4,
1,1,1,1,1,1,1,1,1,1,1,1,1,1,1,1,1,1,1,1,1,1,1,1,1,1,1,1,1,1,1,1,1,1,1,1,
1,1,1,1,1,1,1,1,1,1,1,1,1,1,1,1,1,1,1,1,1,1,1,1,1,1,1,1,1,1,1,1,1,1,1,1,
1,1,1,1,1,1,1,1,1,1,1,1,1,1,1,1,1,1,1,1,1,1,1,1,1,1,1,1,1,1,1,1,1,1,1,1,
1,1,1,1,1,1,1,1,1,1,1,1,1,1,1,1,1,1,1,1,1,1,1,1,1,1,1,1,1,1,1,1,1,1,1,1,
1,1,1,1,1,4),(0.,0.0262983047615875),(13.02168033215,14.0156270002435,15.009573668337,
16.0035203364305,16.997467004524,17.9914136726175,18.9853603407109,19.9793070088044,
20.9732536768979,21.9672003449914,22.9611470130849,23.9550936811784,24.9490403492719,
25.9429870173654,26.9369336854589,27.9308803535524,28.9248270216459,29.9187736897394,
30.9127203578329,31.9066670259264,32.9006136940199,33.8945603621134,34.8885070302068,
35.8824536983003,36.8764003663938,37.8703470344873,38.8642937025808,39.8582403706743,
40.8521870387678,41.8461337068613,42.8400803749548,43.8340270430483,44.8279737111418,
45.8219203792353,46.8158670473288,47.8098137154223,48.8037603835158,49.7977070516092,
50.7916537197027,51.7856003877962,52.7795470558897,53.7734937239832,54.7674403920767,
55.7613870601702,56.7553337282637,57.7492803963572,58.7432270644507,59.7371737325442,
60.7311204006377,61.7250670687312,62.7190137368247,63.7129604049182,64.7069070730116,
65.7008537411051,66.6948004091986,67.6887470772921,68.6826937453856,69.6766404134791,
70.6705870815726,71.6645337496661,72.6584804177596,73.6524270858531,74.6463737539466,
75.6403204220401,76.6342670901336,77.6282137582271,78.6221604263205,79.616107094414,
80.6100537625075,81.604000430601,82.5979470986945,83.591893766788,84.5858404348815,
85.579787102975,86.5737337710685,87.567680439162,88.5616271072555,89.555573775349,
90.5495204434425,91.543467111536,92.5374137796295,93.5313604477229,94.5253071158164,
95.5192537839099,96.5132004520034,97.5071471200969,98.5010937881904,99.4950404562839,
100.488987124377,101.482933792471,102.476880460564,103.470827128658,104.464773796751,
105.458720464845,106.452667132938,107.446613801032,108.440560469125,109.434507137219,
110.428453805312,111.422400473406,112.416347141499,113.410293809593,114.404240477686,
115.39818714578,116.392133813873,117.386080481967,118.38002715006,119.373973818154,
120.367920486247,121.361867154341,122.355813822434,123.349760490528,124.343707158621,
125.337653826715,126.331600494808,127.325547162902,128.319493830995,129.313440499089,
130.307387167182,131.301333835276,132.295280503369,133.289227171463,134.283173839556,
135.27712050765,136.271067175743,137.265013843837,138.25896051193,139.252907180024,
140.246853848117,141.240800516211,142.234747184304,143.228693852398,144.222640520491,
145.216587188585,146.210533856678,147.204480524772,148.198427192865,149.192373860959,
150.186320529052,151.180267197146,152.174213865239,153.168160533333,154.162107201426,
155.15605386952,156.150000537613,157.143947205707,158.1378938738,159.131840541894,
160.125787209987,161.119733878081,162.113680546174),.UNSPECIFIED.);
#477=B_SPLINE_SURFACE_WITH_KNOTS('',3,3,((#47181,#47182,#47183,#47184,#47185,
#47186,#47187,#47188,#47189,#47190,#47191,#47192,#47193,#47194,#47195,#47196,
#47197,#47198,#47199,#47200,#47201,#47202,#47203,#47204,#47205,#47206,#47207,
#47208,#47209,#47210,#47211,#47212,#47213,#47214,#47215,#47216,#47217,#47218,
#47219,#47220,#47221,#47222,#47223,#47224,#47225,#47226,#47227,#47228,#47229,
#47230,#47231,#47232,#47233,#47234,#47235,#47236,#47237,#47238,#47239,#47240,
#47241,#47242,#47243,#47244,#47245,#47246,#47247,#47248,#47249,#47250,#47251,
#47252,#47253,#47254,#47255,#47256,#47257,#47258,#47259,#47260,#47261,#47262,
#47263,#47264,#47265,#47266,#47267,#47268,#47269,#47270,#47271,#47272,#47273,
#47274,#47275,#47276,#47277,#47278,#47279,#47280,#47281,#47282,#47283,#47284,
#47285,#47286,#47287,#47288,#47289,#47290,#47291,#47292,#47293,#47294,#47295,
#47296,#47297,#47298,#47299,#47300,#47301,#47302,#47303,#47304,#47305,#47306,
#47307,#47308,#47309,#47310,#47311,#47312,#47313,#47314,#47315,#47316,#47317,
#47318,#47319,#47320,#47321,#47322,#47323,#47324,#47325,#47326,#47327,#47328,
#47329,#47330,#47331,#47332,#47333),(#47334,#47335,#47336,#47337,#47338,
#47339,#47340,#47341,#47342,#47343,#47344,#47345,#47346,#47347,#47348,#47349,
#47350,#47351,#47352,#47353,#47354,#47355,#47356,#47357,#47358,#47359,#47360,
#47361,#47362,#47363,#47364,#47365,#47366,#47367,#47368,#47369,#47370,#47371,
#47372,#47373,#47374,#47375,#47376,#47377,#47378,#47379,#47380,#47381,#47382,
#47383,#47384,#47385,#47386,#47387,#47388,#47389,#47390,#47391,#47392,#47393,
#47394,#47395,#47396,#47397,#47398,#47399,#47400,#47401,#47402,#47403,#47404,
#47405,#47406,#47407,#47408,#47409,#47410,#47411,#47412,#47413,#47414,#47415,
#47416,#47417,#47418,#47419,#47420,#47421,#47422,#47423,#47424,#47425,#47426,
#47427,#47428,#47429,#47430,#47431,#47432,#47433,#47434,#47435,#47436,#47437,
#47438,#47439,#47440,#47441,#47442,#47443,#47444,#47445,#47446,#47447,#47448,
#47449,#47450,#47451,#47452,#47453,#47454,#47455,#47456,#47457,#47458,#47459,
#47460,#47461,#47462,#47463,#47464,#47465,#47466,#47467,#47468,#47469,#47470,
#47471,#47472,#47473,#47474,#47475,#47476,#47477,#47478,#47479,#47480,#47481,
#47482,#47483,#47484,#47485,#47486),(#47487,#47488,#47489,#47490,#47491,
#47492,#47493,#47494,#47495,#47496,#47497,#47498,#47499,#47500,#47501,#47502,
#47503,#47504,#47505,#47506,#47507,#47508,#47509,#47510,#47511,#47512,#47513,
#47514,#47515,#47516,#47517,#47518,#47519,#47520,#47521,#47522,#47523,#47524,
#47525,#47526,#47527,#47528,#47529,#47530,#47531,#47532,#47533,#47534,#47535,
#47536,#47537,#47538,#47539,#47540,#47541,#47542,#47543,#47544,#47545,#47546,
#47547,#47548,#47549,#47550,#47551,#47552,#47553,#47554,#47555,#47556,#47557,
#47558,#47559,#47560,#47561,#47562,#47563,#47564,#47565,#47566,#47567,#47568,
#47569,#47570,#47571,#47572,#47573,#47574,#47575,#47576,#47577,#47578,#47579,
#47580,#47581,#47582,#47583,#47584,#47585,#47586,#47587,#47588,#47589,#47590,
#47591,#47592,#47593,#47594,#47595,#47596,#47597,#47598,#47599,#47600,#47601,
#47602,#47603,#47604,#47605,#47606,#47607,#47608,#47609,#47610,#47611,#47612,
#47613,#47614,#47615,#47616,#47617,#47618,#47619,#47620,#47621,#47622,#47623,
#47624,#47625,#47626,#47627,#47628,#47629,#47630,#47631,#47632,#47633,#47634,
#47635,#47636,#47637,#47638,#47639),(#47640,#47641,#47642,#47643,#47644,
#47645,#47646,#47647,#47648,#47649,#47650,#47651,#47652,#47653,#47654,#47655,
#47656,#47657,#47658,#47659,#47660,#47661,#47662,#47663,#47664,#47665,#47666,
#47667,#47668,#47669,#47670,#47671,#47672,#47673,#47674,#47675,#47676,#47677,
#47678,#47679,#47680,#47681,#47682,#47683,#47684,#47685,#47686,#47687,#47688,
#47689,#47690,#47691,#47692,#47693,#47694,#47695,#47696,#47697,#47698,#47699,
#47700,#47701,#47702,#47703,#47704,#47705,#47706,#47707,#47708,#47709,#47710,
#47711,#47712,#47713,#47714,#47715,#47716,#47717,#47718,#47719,#47720,#47721,
#47722,#47723,#47724,#47725,#47726,#47727,#47728,#47729,#47730,#47731,#47732,
#47733,#47734,#47735,#47736,#47737,#47738,#47739,#47740,#47741,#47742,#47743,
#47744,#47745,#47746,#47747,#47748,#47749,#47750,#47751,#47752,#47753,#47754,
#47755,#47756,#47757,#47758,#47759,#47760,#47761,#47762,#47763,#47764,#47765,
#47766,#47767,#47768,#47769,#47770,#47771,#47772,#47773,#47774,#47775,#47776,
#47777,#47778,#47779,#47780,#47781,#47782,#47783,#47784,#47785,#47786,#47787,
#47788,#47789,#47790,#47791,#47792)),.UNSPECIFIED.,.F.,.F.,.F.,(4,4),(4,
1,1,1,1,1,1,1,1,1,1,1,1,1,1,1,1,1,1,1,1,1,1,1,1,1,1,1,1,1,1,1,1,1,1,1,1,
1,1,1,1,1,1,1,1,1,1,1,1,1,1,1,1,1,1,1,1,1,1,1,1,1,1,1,1,1,1,1,1,1,1,1,1,
1,1,1,1,1,1,1,1,1,1,1,1,1,1,1,1,1,1,1,1,1,1,1,1,1,1,1,1,1,1,1,1,1,1,1,1,
1,1,1,1,1,1,1,1,1,1,1,1,1,1,1,1,1,1,1,1,1,1,1,1,1,1,1,1,1,1,1,1,1,1,1,1,
1,1,1,1,1,4),(0.,0.0262983047615874),(16.3287821777262,17.3227288458197,
18.3166755139132,19.3106221820067,20.3045688501002,21.2985155181937,22.2924621862871,
23.2864088543806,24.2803555224741,25.2743021905676,26.2682488586611,27.2621955267546,
28.2561421948481,29.2500888629416,30.2440355310351,31.2379821991286,32.2319288672221,
33.2258755353156,34.2198222034091,35.2137688715026,36.2077155395961,37.2016622076895,
38.195608875783,39.1895555438765,40.18350221197,41.1774488800635,42.171395548157,
43.1653422162505,44.159288884344,45.1532355524375,46.147182220531,47.1411288886245,
48.135075556718,49.1290222248115,50.122968892905,51.1169155609985,52.1108622290919,
53.1048088971854,54.0987555652789,55.0927022333724,56.0866489014659,57.0805955695594,
58.0745422376529,59.0684889057464,60.0624355738399,61.0563822419334,62.0503289100269,
63.0442755781204,64.0382222462139,65.0321689143073,66.0261155824008,67.0200622504943,
68.0140089185878,69.0079555866813,70.0019022547748,70.9958489228683,71.9897955909618,
72.9837422590553,73.9776889271488,74.9716355952423,75.9655822633358,76.9595289314293,
77.9534755995228,78.9474222676163,79.9413689357097,80.9353156038032,81.9292622718967,
82.9232089399902,83.9171556080837,84.9111022761772,85.9050489442707,86.8989956123642,
87.8929422804577,88.8868889485512,89.8808356166447,90.8747822847382,91.8687289528317,
92.8626756209252,93.8566222890186,94.8505689571121,95.8445156252056,96.8384622932991,
97.8324089613926,98.8263556294861,99.8203022975796,100.814248965673,101.808195633767,
102.80214230186,103.796088969954,104.790035638047,105.783982306141,106.777928974234,
107.771875642328,108.765822310421,109.759768978515,110.753715646608,111.747662314702,
112.741608982795,113.735555650889,114.729502318982,115.723448987075,116.717395655169,
117.711342323262,118.705288991356,119.699235659449,120.693182327543,121.687128995636,
122.68107566373,123.675022331823,124.668968999917,125.66291566801,126.656862336104,
127.650809004197,128.644755672291,129.638702340384,130.632649008478,131.626595676571,
132.620542344665,133.614489012758,134.608435680852,135.602382348945,136.596329017039,
137.590275685132,138.584222353226,139.578169021319,140.572115689413,141.566062357506,
142.5600090256,143.553955693693,144.547902361787,145.54184902988,146.535795697974,
147.529742366067,148.523689034161,149.517635702254,150.511582370348,151.505529038441,
152.499475706535,153.493422374628,154.487369042722,155.481315710815,156.475262378909,
157.469209047002,158.463155715096,159.457102383189,160.451049051283,161.444995719376,
162.43894238747,163.432889055563,164.426835723657,165.42078239175),
 .UNSPECIFIED.);
#689=B_SPLINE_CURVE_WITH_KNOTS('',3,(#44634,#44635,#44636,#44637,#44638,
#44639,#44640,#44641,#44642,#44643,#44644,#44645,#44646),.UNSPECIFIED.,
 .F.,.F.,(4,3,3,3,4),(-5.66236639740237,-4.96973334046747,-3.97578667237397,
-2.98184000428048,-2.06546402602168),.UNSPECIFIED.);
#690=B_SPLINE_CURVE_WITH_KNOTS('',3,(#44654,#44655,#44656,#44657,#44658,
#44659,#44660,#44661,#44662,#44663),.UNSPECIFIED.,.F.,.F.,(4,3,3,4),(0.,
0.993946668093495,1.98789333618699,2.68628293579895),.UNSPECIFIED.);
#691=B_SPLINE_CURVE_WITH_KNOTS('',3,(#44668,#44669,#44670,#44671,#44672,
#44673,#44674,#44675,#44676,#44677,#44678,#44679,#44680,#44681,#44682,#44683,
#44684,#44685,#44686,#44687,#44688,#44689,#44690,#44691,#44692),
 .UNSPECIFIED.,.F.,.F.,(4,3,3,3,3,3,3,3,4),(-11.945551704582,-11.9273600171219,
-10.9334133490284,-9.93946668093493,-8.94552001284144,-7.95157334474795,
-6.95762667665445,-5.96368000856096,-5.66236639740237),.UNSPECIFIED.);
#692=B_SPLINE_CURVE_WITH_KNOTS('',3,(#44693,#44694,#44695,#44696,#44697,
#44698,#44699,#44700,#44701,#44702,#44703,#44704,#44705,#44706,#44707,#44708,
#44709,#44710,#44711,#44712,#44713,#44714,#44715,#44716,#44717),
 .UNSPECIFIED.,.F.,.F.,(4,3,3,3,3,3,3,3,4),(2.68628293579895,2.98184000428049,
3.97578667237398,4.96973334046747,5.96368000856096,6.95762667665446,7.95157334474795,
8.94552001284145,8.96946824297854),.UNSPECIFIED.);
#693=B_SPLINE_CURVE_WITH_KNOTS('',3,(#44722,#44723,#44724,#44725,#44726,
#44727,#44728,#44729,#44730,#44731,#44732,#44733,#44734,#44735,#44736,#44737,
#44738,#44739,#44740,#44741,#44742,#44743),.UNSPECIFIED.,.F.,.F.,(4,3,3,
3,3,3,3,4),(-18.2287370117615,-17.8910400256829,-16.8970933575894,-15.9031466894959,
-14.9092000214024,-13.9152533533089,-12.9213066852154,-11.945551704582),
 .UNSPECIFIED.);
#694=B_SPLINE_CURVE_WITH_KNOTS('',3,(#44744,#44745,#44746,#44747,#44748,
#44749,#44750,#44751,#44752,#44753,#44754,#44755,#44756,#44757,#44758,#44759,
#44760,#44761,#44762,#44763,#44764,#44765),.UNSPECIFIED.,.F.,.F.,(4,3,3,
3,3,3,3,4),(8.96946824297854,9.93946668093494,10.9334133490284,11.9273600171219,
12.9213066852154,13.9152533533089,14.9092000214024,15.2526535501581),
 .UNSPECIFIED.);
#695=B_SPLINE_CURVE_WITH_KNOTS('',3,(#44770,#44771,#44772,#44773,#44774,
#44775,#44776,#44777,#44778,#44779,#44780,#44781,#44782,#44783,#44784,#44785,
#44786,#44787,#44788,#44789,#44790,#44791),.UNSPECIFIED.,.F.,.F.,(4,3,3,
3,3,3,3,4),(-24.5119223189411,-23.8547200342438,-22.8607733661503,-21.8668266980569,
-20.8728800299634,-19.8789333618699,-18.8849866937764,-18.2287370117615),
 .UNSPECIFIED.);
#696=B_SPLINE_CURVE_WITH_KNOTS('',3,(#44792,#44793,#44794,#44795,#44796,
#44797,#44798,#44799,#44800,#44801,#44802,#44803,#44804,#44805,#44806,#44807,
#44808,#44809,#44810,#44811,#44812,#44813),.UNSPECIFIED.,.F.,.F.,(4,3,3,
3,3,3,3,4),(15.2526535501581,15.9031466894959,16.8970933575894,17.8910400256829,
18.8849866937764,19.8789333618699,20.8728800299634,21.5358388573377),
 .UNSPECIFIED.);
#697=B_SPLINE_CURVE_WITH_KNOTS('',3,(#44818,#44819,#44820,#44821,#44822,
#44823,#44824,#44825,#44826,#44827,#44828,#44829,#44830,#44831,#44832,#44833,
#44834,#44835,#44836,#44837,#44838,#44839),.UNSPECIFIED.,.F.,.F.,(4,3,3,
3,3,3,3,4),(-30.7951076261207,-29.8184000428048,-28.8244533747113,-27.8305067066178,
-26.8365600385243,-25.8426133704308,-24.8486667023373,-24.5119223189411),
 .UNSPECIFIED.);
#698=B_SPLINE_CURVE_WITH_KNOTS('',3,(#44840,#44841,#44842,#44843,#44844,
#44845,#44846,#44847,#44848,#44849,#44850,#44851,#44852,#44853,#44854,#44855,
#44856,#44857,#44858,#44859,#44860,#44861),.UNSPECIFIED.,.F.,.F.,(4,3,3,
3,3,3,3,4),(21.5358388573377,21.8668266980569,22.8607733661503,23.8547200342438,
24.8486667023373,25.8426133704308,26.8365600385243,27.8190241645173),
 .UNSPECIFIED.);
#699=B_SPLINE_CURVE_WITH_KNOTS('',3,(#44866,#44867,#44868,#44869,#44870,
#44871,#44872,#44873,#44874,#44875,#44876,#44877,#44878,#44879,#44880,#44881,
#44882,#44883,#44884,#44885,#44886,#44887,#44888,#44889,#44890),
 .UNSPECIFIED.,.F.,.F.,(4,3,3,3,3,3,3,3,4),(-37.0782929333003,-36.7760267194593,
-35.7820800513658,-34.7881333832723,-33.7941867151788,-32.8002400470853,
-31.8062933789918,-30.8123467108983,-30.7951076261207),.UNSPECIFIED.);
#700=B_SPLINE_CURVE_WITH_KNOTS('',3,(#44891,#44892,#44893,#44894,#44895,
#44896,#44897,#44898,#44899,#44900,#44901,#44902,#44903,#44904,#44905,#44906,
#44907,#44908,#44909,#44910,#44911,#44912,#44913,#44914,#44915),
 .UNSPECIFIED.,.F.,.F.,(4,3,3,3,3,3,3,3,4),(27.8190241645173,27.8305067066178,
28.8244533747113,29.8184000428048,30.8123467108983,31.8062933789918,32.8002400470853,
33.7941867151788,34.1022094716969),.UNSPECIFIED.);
#701=B_SPLINE_CURVE_WITH_KNOTS('',3,(#44920,#44921,#44922,#44923,#44924,
#44925,#44926,#44927,#44928,#44929,#44930,#44931,#44932,#44933,#44934,#44935,
#44936,#44937,#44938,#44939,#44940,#44941),.UNSPECIFIED.,.F.,.F.,(4,3,3,
3,3,3,3,4),(-43.3614782404799,-42.7397067280202,-41.7457600599267,-40.7518133918332,
-39.7578667237397,-38.7639200556462,-37.7699733875527,-37.0782929333003),
 .UNSPECIFIED.);
#702=B_SPLINE_CURVE_WITH_KNOTS('',3,(#44942,#44943,#44944,#44945,#44946,
#44947,#44948,#44949,#44950,#44951,#44952,#44953,#44954,#44955,#44956,#44957,
#44958,#44959,#44960,#44961,#44962,#44963),.UNSPECIFIED.,.F.,.F.,(4,3,3,
3,3,3,3,4),(34.1022094716969,34.7881333832723,35.7820800513658,36.7760267194593,
37.7699733875528,38.7639200556462,39.7578667237397,40.3853947788765),
 .UNSPECIFIED.);
#703=B_SPLINE_CURVE_WITH_KNOTS('',3,(#44968,#44969,#44970,#44971,#44972,
#44973,#44974,#44975,#44976,#44977,#44978,#44979,#44980,#44981,#44982,#44983,
#44984,#44985,#44986,#44987,#44988,#44989),.UNSPECIFIED.,.F.,.F.,(4,3,3,
3,3,3,3,4),(-49.6446635476595,-48.7033867365812,-47.7094400684877,-46.7154934003942,
-45.7215467323007,-44.7276000642072,-43.7336533961137,-43.3614782404799),
 .UNSPECIFIED.);
#704=B_SPLINE_CURVE_WITH_KNOTS('',3,(#44990,#44991,#44992,#44993,#44994,
#44995,#44996,#44997,#44998,#44999,#45000,#45001,#45002,#45003,#45004,#45005,
#45006,#45007,#45008,#45009,#45010,#45011),.UNSPECIFIED.,.F.,.F.,(4,3,3,
3,3,3,3,4),(40.3853947788765,40.7518133918332,41.7457600599267,42.7397067280202,
43.7336533961137,44.7276000642072,45.7215467323007,46.6685800860561),
 .UNSPECIFIED.);
#705=B_SPLINE_CURVE_WITH_KNOTS('',3,(#45016,#45017,#45018,#45019,#45020,
#45021,#45022,#45023,#45024,#45025,#45026,#45027,#45028,#45029,#45030,#45031,
#45032,#45033,#45034,#45035,#45036,#45037,#45038,#45039,#45040),
 .UNSPECIFIED.,.F.,.F.,(4,3,3,3,3,3,3,3,4),(-55.9278488548391,-55.6610134132356,
-54.6670667451421,-53.6731200770486,-52.6791734089552,-51.6852267408617,
-50.6912800727682,-49.6973334046747,-49.6446635476595),.UNSPECIFIED.);
#706=B_SPLINE_CURVE_WITH_KNOTS('',3,(#45041,#45042,#45043,#45044,#45045,
#45046,#45047,#45048,#45049,#45050,#45051,#45052,#45053,#45054,#45055,#45056,
#45057,#45058,#45059,#45060,#45061,#45062,#45063,#45064,#45065),
 .UNSPECIFIED.,.F.,.F.,(4,3,3,3,3,3,3,3,4),(46.6685800860561,46.7154934003942,
47.7094400684877,48.7033867365812,49.6973334046747,50.6912800727682,51.6852267408617,
52.6791734089551,52.9517653932357),.UNSPECIFIED.);
#707=B_SPLINE_CURVE_WITH_KNOTS('',3,(#45070,#45071,#45072,#45073,#45074,
#45075,#45076,#45077,#45078,#45079,#45080,#45081,#45082,#45083,#45084,#45085,
#45086,#45087,#45088,#45089,#45090,#45091),.UNSPECIFIED.,.F.,.F.,(4,3,3,
3,3,3,3,4),(-62.2110341620187,-61.6246934217966,-60.6307467537031,-59.6368000856096,
-58.6428534175161,-57.6489067494226,-56.6549600813291,-55.9278488548391),
 .UNSPECIFIED.);
#708=B_SPLINE_CURVE_WITH_KNOTS('',3,(#45092,#45093,#45094,#45095,#45096,
#45097,#45098,#45099,#45100,#45101,#45102,#45103,#45104,#45105,#45106,#45107,
#45108,#45109,#45110,#45111,#45112,#45113),.UNSPECIFIED.,.F.,.F.,(4,3,3,
3,3,3,3,4),(52.9517653932357,53.6731200770486,54.6670667451421,55.6610134132356,
56.6549600813291,57.6489067494226,58.6428534175161,59.2349507004152),
 .UNSPECIFIED.);
#709=B_SPLINE_CURVE_WITH_KNOTS('',3,(#45118,#45119,#45120,#45121,#45122,
#45123,#45124,#45125,#45126,#45127,#45128,#45129,#45130,#45131,#45132,#45133,
#45134,#45135,#45136,#45137,#45138,#45139),.UNSPECIFIED.,.F.,.F.,(4,3,3,
3,3,3,3,4),(-68.4942194691983,-67.5883734303575,-66.5944267622641,-65.6004800941705,
-64.6065334260771,-63.6125867579836,-62.6186400898901,-62.2110341620187),
 .UNSPECIFIED.);
#710=B_SPLINE_CURVE_WITH_KNOTS('',3,(#45140,#45141,#45142,#45143,#45144,
#45145,#45146,#45147,#45148,#45149,#45150,#45151,#45152,#45153,#45154,#45155,
#45156,#45157,#45158,#45159,#45160,#45161),.UNSPECIFIED.,.F.,.F.,(4,3,3,
3,3,3,3,4),(59.2349507004152,59.6368000856096,60.6307467537031,61.6246934217966,
62.6186400898901,63.6125867579836,64.6065334260771,65.5181360075948),
 .UNSPECIFIED.);
#711=B_SPLINE_CURVE_WITH_KNOTS('',3,(#45166,#45167,#45168,#45169,#45170,
#45171,#45172,#45173,#45174,#45175,#45176,#45177,#45178,#45179,#45180,#45181,
#45182,#45183,#45184,#45185,#45186,#45187,#45188,#45189,#45190),
 .UNSPECIFIED.,.F.,.F.,(4,3,3,3,3,3,3,3,4),(-74.7774047763779,-74.546000107012,
-73.5520534389185,-72.558106770825,-71.5641601027315,-70.570213434638,-69.5762667665445,
-68.582320098451,-68.4942194691983),.UNSPECIFIED.);
#712=B_SPLINE_CURVE_WITH_KNOTS('',3,(#45191,#45192,#45193,#45194,#45195,
#45196,#45197,#45198,#45199,#45200,#45201,#45202,#45203,#45204,#45205,#45206,
#45207,#45208,#45209,#45210,#45211,#45212,#45213,#45214,#45215),
 .UNSPECIFIED.,.F.,.F.,(4,3,3,3,3,3,3,3,4),(65.5181360075948,65.6004800941706,
66.5944267622641,67.5883734303575,68.582320098451,69.5762667665445,70.570213434638,
71.5641601027315,71.8013213147744),.UNSPECIFIED.);
#713=B_SPLINE_CURVE_WITH_KNOTS('',3,(#45220,#45221,#45222,#45223,#45224,
#45225,#45226,#45227,#45228,#45229,#45230,#45231,#45232,#45233,#45234,#45235,
#45236,#45237,#45238,#45239,#45240,#45241),.UNSPECIFIED.,.F.,.F.,(4,3,3,
3,3,3,3,4),(-81.0605900835575,-80.5096801155729,-79.5157334474794,-78.521786779386,
-77.5278401112925,-76.533893443199,-75.5399467751055,-74.7774047763779),
 .UNSPECIFIED.);
#714=B_SPLINE_CURVE_WITH_KNOTS('',3,(#45242,#45243,#45244,#45245,#45246,
#45247,#45248,#45249,#45250,#45251,#45252,#45253,#45254,#45255,#45256,#45257,
#45258,#45259,#45260,#45261,#45262,#45263),.UNSPECIFIED.,.F.,.F.,(4,3,3,
3,3,3,3,4),(71.8013213147744,72.558106770825,73.5520534389185,74.546000107012,
75.5399467751055,76.533893443199,77.5278401112925,78.084506621954),
 .UNSPECIFIED.);
#715=B_SPLINE_CURVE_WITH_KNOTS('',3,(#45268,#45269,#45270,#45271,#45272,
#45273,#45274,#45275,#45276,#45277,#45278,#45279,#45280,#45281,#45282,#45283,
#45284,#45285,#45286,#45287,#45288,#45289),.UNSPECIFIED.,.F.,.F.,(4,3,3,
3,3,3,3,4),(-87.343775390737,-86.4733601241339,-85.4794134560404,-84.4854667879469,
-83.4915201198534,-82.4975734517599,-81.5036267836664,-81.0605900835575),
 .UNSPECIFIED.);
#716=B_SPLINE_CURVE_WITH_KNOTS('',3,(#45290,#45291,#45292,#45293,#45294,
#45295,#45296,#45297,#45298,#45299,#45300,#45301,#45302,#45303,#45304,#45305,
#45306,#45307,#45308,#45309,#45310,#45311),.UNSPECIFIED.,.F.,.F.,(4,3,3,
3,3,3,3,4),(78.084506621954,78.521786779386,79.5157334474795,80.509680115573,
81.5036267836665,82.4975734517599,83.4915201198534,84.3676919291336),
 .UNSPECIFIED.);
#717=B_SPLINE_CURVE_WITH_KNOTS('',3,(#45316,#45317,#45318,#45319,#45320,
#45321,#45322,#45323,#45324,#45325,#45326,#45327,#45328,#45329,#45330,#45331,
#45332,#45333,#45334,#45335,#45336,#45337,#45338,#45339,#45340),
 .UNSPECIFIED.,.F.,.F.,(4,3,3,3,3,3,3,3,4),(-93.6269606979166,-93.4309868007884,
-92.4370401326949,-91.4430934646014,-90.4491467965079,-89.4552001284144,
-88.4612534603209,-87.4673067922274,-87.343775390737),.UNSPECIFIED.);
#718=B_SPLINE_CURVE_WITH_KNOTS('',3,(#45341,#45342,#45343,#45344,#45345,
#45346,#45347,#45348,#45349,#45350,#45351,#45352,#45353,#45354,#45355,#45356,
#45357,#45358,#45359,#45360,#45361,#45362,#45363,#45364,#45365),
 .UNSPECIFIED.,.F.,.F.,(4,3,3,3,3,3,3,3,4),(84.3676919291336,84.4854667879469,
85.4794134560404,86.4733601241339,87.4673067922274,88.4612534603209,89.4552001284144,
90.4491467965079,90.6508772363132),.UNSPECIFIED.);
#719=B_SPLINE_CURVE_WITH_KNOTS('',3,(#45370,#45371,#45372,#45373,#45374,
#45375,#45376,#45377,#45378,#45379,#45380,#45381,#45382,#45383,#45384,#45385,
#45386,#45387,#45388,#45389,#45390,#45391),.UNSPECIFIED.,.F.,.F.,(4,3,3,
3,3,3,3,4),(-99.9101460050962,-99.3946668093493,-98.4007201412558,-97.4067734731623,
-96.4128268050689,-95.4188801369753,-94.4249334688819,-93.6269606979166),
 .UNSPECIFIED.);
#720=B_SPLINE_CURVE_WITH_KNOTS('',3,(#45392,#45393,#45394,#45395,#45396,
#45397,#45398,#45399,#45400,#45401,#45402,#45403,#45404,#45405,#45406,#45407,
#45408,#45409,#45410,#45411,#45412,#45413),.UNSPECIFIED.,.F.,.F.,(4,3,3,
3,3,3,3,4),(90.6508772363132,91.4430934646014,92.4370401326949,93.4309868007884,
94.4249334688819,95.4188801369754,96.4128268050689,96.9340625434928),
 .UNSPECIFIED.);
#721=B_SPLINE_CURVE_WITH_KNOTS('',3,(#45418,#45419,#45420,#45421,#45422,
#45423,#45424,#45425,#45426,#45427,#45428,#45429,#45430,#45431,#45432,#45433,
#45434,#45435,#45436,#45437,#45438,#45439),.UNSPECIFIED.,.F.,.F.,(4,3,3,
3,3,3,3,4),(-106.193331312276,-105.35834681791,-104.364400149817,-103.370453481723,
-102.37650681363,-101.382560145536,-100.388613477443,-99.9101460050962),
 .UNSPECIFIED.);
#722=B_SPLINE_CURVE_WITH_KNOTS('',3,(#45440,#45441,#45442,#45443,#45444,
#45445,#45446,#45447,#45448,#45449,#45450,#45451,#45452,#45453,#45454,#45455,
#45456,#45457,#45458,#45459,#45460,#45461),.UNSPECIFIED.,.F.,.F.,(4,3,3,
3,3,3,3,4),(96.9340625434928,97.4067734731624,98.4007201412558,99.3946668093493,
100.388613477443,101.382560145536,102.37650681363,103.217247850672),
 .UNSPECIFIED.);
#723=B_SPLINE_CURVE_WITH_KNOTS('',3,(#45466,#45467,#45468,#45469,#45470,
#45471,#45472,#45473,#45474,#45475,#45476,#45477,#45478,#45479,#45480,#45481,
#45482,#45483,#45484,#45485,#45486,#45487,#45488,#45489,#45490),
 .UNSPECIFIED.,.F.,.F.,(4,3,3,3,3,3,3,3,4),(-112.476516619455,-112.315973494565,
-111.322026826471,-110.328080158378,-109.334133490284,-108.340186822191,
-107.346240154097,-106.352293486004,-106.193331312276),.UNSPECIFIED.);
#724=B_SPLINE_CURVE_WITH_KNOTS('',3,(#45491,#45492,#45493,#45494,#45495,
#45496,#45497,#45498,#45499,#45500,#45501,#45502,#45503,#45504,#45505,#45506,
#45507,#45508,#45509,#45510,#45511,#45512,#45513,#45514,#45515),
 .UNSPECIFIED.,.F.,.F.,(4,3,3,3,3,3,3,3,4),(103.217247850672,103.370453481723,
104.364400149817,105.35834681791,106.352293486004,107.346240154097,108.340186822191,
109.334133490284,109.500433157852),.UNSPECIFIED.);
#725=B_SPLINE_CURVE_WITH_KNOTS('',3,(#45520,#45521,#45522,#45523,#45524,
#45525,#45526,#45527,#45528,#45529,#45530,#45531,#45532,#45533,#45534,#45535,
#45536,#45537,#45538,#45539,#45540,#45541),.UNSPECIFIED.,.F.,.F.,(4,3,3,
3,3,3,3,4),(-118.759701926635,-118.279653503126,-117.285706835032,-116.291760166939,
-115.297813498845,-114.303866830752,-113.309920162658,-112.476516619455),
 .UNSPECIFIED.);
#726=B_SPLINE_CURVE_WITH_KNOTS('',3,(#45542,#45543,#45544,#45545,#45546,
#45547,#45548,#45549,#45550,#45551,#45552,#45553,#45554,#45555,#45556,#45557,
#45558,#45559,#45560,#45561,#45562,#45563),.UNSPECIFIED.,.F.,.F.,(4,3,3,
3,3,3,3,4),(109.500433157852,110.328080158378,111.322026826471,112.315973494565,
113.309920162658,114.303866830752,115.297813498845,115.783618465032),
 .UNSPECIFIED.);
#727=B_SPLINE_CURVE_WITH_KNOTS('',3,(#45568,#45569,#45570,#45571,#45572,
#45573,#45574,#45575,#45576,#45577,#45578,#45579,#45580,#45581,#45582,#45583,
#45584,#45585,#45586,#45587,#45588,#45589),.UNSPECIFIED.,.F.,.F.,(4,3,3,
3,3,3,3,4),(-125.042887233815,-124.243333511687,-123.249386843593,-122.2554401755,
-121.261493507406,-120.267546839313,-119.273600171219,-118.759701926635),
 .UNSPECIFIED.);
#728=B_SPLINE_CURVE_WITH_KNOTS('',3,(#45590,#45591,#45592,#45593,#45594,
#45595,#45596,#45597,#45598,#45599,#45600,#45601,#45602,#45603,#45604,#45605,
#45606,#45607,#45608,#45609,#45610,#45611),.UNSPECIFIED.,.F.,.F.,(4,3,3,
3,3,3,3,4),(115.783618465032,116.291760166939,117.285706835032,118.279653503126,
119.273600171219,120.267546839313,121.261493507406,122.066803772211),
 .UNSPECIFIED.);
#729=B_SPLINE_CURVE_WITH_KNOTS('',3,(#45616,#45617,#45618,#45619,#45620,
#45621,#45622,#45623,#45624,#45625,#45626,#45627,#45628,#45629,#45630,#45631,
#45632,#45633,#45634,#45635,#45636,#45637,#45638,#45639,#45640),
 .UNSPECIFIED.,.F.,.F.,(4,3,3,3,3,3,3,3,4),(-131.326072540994,-131.200960188341,
-130.207013520248,-129.213066852154,-128.219120184061,-127.225173515967,
-126.231226847874,-125.23728017978,-125.042887233815),.UNSPECIFIED.);
#730=B_SPLINE_CURVE_WITH_KNOTS('',3,(#45641,#45642,#45643,#45644,#45645,
#45646,#45647,#45648,#45649,#45650,#45651,#45652,#45653,#45654,#45655,#45656,
#45657,#45658,#45659,#45660,#45661,#45662,#45663,#45664,#45665),
 .UNSPECIFIED.,.F.,.F.,(4,3,3,3,3,3,3,3,4),(122.066803772211,122.2554401755,
123.249386843593,124.243333511687,125.23728017978,126.231226847874,127.225173515967,
128.219120184061,128.349989079391),.UNSPECIFIED.);
#731=B_SPLINE_CURVE_WITH_KNOTS('',3,(#45670,#45671,#45672,#45673,#45674,
#45675,#45676,#45677,#45678,#45679,#45680,#45681,#45682,#45683,#45684,#45685,
#45686,#45687,#45688,#45689,#45690,#45691),.UNSPECIFIED.,.F.,.F.,(4,3,3,
3,3,3,3,4),(-137.609257848174,-137.164640196902,-136.170693528809,-135.176746860715,
-134.182800192622,-133.188853524528,-132.194906856435,-131.326072540994),
 .UNSPECIFIED.);
#732=B_SPLINE_CURVE_WITH_KNOTS('',3,(#45692,#45693,#45694,#45695,#45696,
#45697,#45698,#45699,#45700,#45701,#45702,#45703,#45704,#45705,#45706,#45707,
#45708,#45709,#45710,#45711,#45712,#45713),.UNSPECIFIED.,.F.,.F.,(4,3,3,
3,3,3,3,4),(128.349989079391,129.213066852154,130.207013520248,131.200960188341,
132.194906856435,133.188853524528,134.182800192622,134.63317438657),
 .UNSPECIFIED.);
#733=B_SPLINE_CURVE_WITH_KNOTS('',3,(#45718,#45719,#45720,#45721,#45722,
#45723,#45724,#45725,#45726,#45727,#45728,#45729,#45730,#45731,#45732,#45733,
#45734,#45735,#45736,#45737,#45738,#45739),.UNSPECIFIED.,.F.,.F.,(4,3,3,
3,3,3,3,4),(-143.892443155353,-143.128320205463,-142.13437353737,-141.140426869276,
-140.146480201183,-139.152533533089,-138.158586864996,-137.609257848174),
 .UNSPECIFIED.);
#734=B_SPLINE_CURVE_WITH_KNOTS('',3,(#45740,#45741,#45742,#45743,#45744,
#45745,#45746,#45747,#45748,#45749,#45750,#45751,#45752,#45753,#45754,#45755,
#45756,#45757,#45758,#45759,#45760,#45761),.UNSPECIFIED.,.F.,.F.,(4,3,3,
3,3,3,3,4),(134.63317438657,135.176746860715,136.170693528809,137.164640196902,
138.158586864996,139.152533533089,140.146480201183,140.91635969375),
 .UNSPECIFIED.);
#735=B_SPLINE_CURVE_WITH_KNOTS('',3,(#45767,#45768,#45769,#45770,#45771,
#45772,#45773),.UNSPECIFIED.,.F.,.F.,(4,1,1,1,4),(160.221225333079,160.451049051283,
161.444995719376,162.43894238747,163.355318365728),.UNSPECIFIED.);
#736=B_SPLINE_CURVE_WITH_KNOTS('',3,(#45776,#45777,#45778,#45779,#45780),
 .UNSPECIFIED.,.F.,.F.,(4,1,4),(160.221225333079,161.119733878081,162.113680546174),
 .UNSPECIFIED.);
#737=B_SPLINE_CURVE_WITH_KNOTS('',3,(#45785,#45786,#45787,#45788,#45789,
#45790,#45791,#45792,#45793,#45794),.UNSPECIFIED.,.F.,.F.,(4,1,1,1,1,1,
1,4),(153.9380400259,154.487369042722,155.481315710815,156.475262378909,
157.469209047002,158.463155715096,159.457102383189,160.221225333079),
 .UNSPECIFIED.);
#738=B_SPLINE_CURVE_WITH_KNOTS('',3,(#45795,#45796,#45797,#45798,#45799,
#45800,#45801,#45802,#45803,#45804,#45805),.UNSPECIFIED.,.F.,.F.,(4,1,1,
1,1,1,1,1,4),(153.9380400259,154.162107201426,155.15605386952,156.150000537613,
157.143947205707,158.1378938738,159.131840541894,160.125787209987,160.221225333079),
 .UNSPECIFIED.);
#739=B_SPLINE_CURVE_WITH_KNOTS('',3,(#45810,#45811,#45812,#45813,#45814,
#45815,#45816,#45817,#45818,#45819),.UNSPECIFIED.,.F.,.F.,(4,1,1,1,1,1,
1,4),(147.65485471872,148.523689034161,149.517635702254,150.511582370348,
151.505529038441,152.499475706535,153.493422374628,153.9380400259),
 .UNSPECIFIED.);
#740=B_SPLINE_CURVE_WITH_KNOTS('',3,(#45820,#45821,#45822,#45823,#45824,
#45825,#45826,#45827,#45828,#45829),.UNSPECIFIED.,.F.,.F.,(4,1,1,1,1,1,
1,4),(147.65485471872,148.198427192865,149.192373860959,150.186320529052,
151.180267197146,152.174213865239,153.168160533333,153.9380400259),
 .UNSPECIFIED.);
#741=B_SPLINE_CURVE_WITH_KNOTS('',3,(#45834,#45835,#45836,#45837,#45838,
#45839,#45840,#45841,#45842,#45843,#45844),.UNSPECIFIED.,.F.,.F.,(4,1,1,
1,1,1,1,1,4),(141.371669411541,141.566062357506,142.5600090256,143.553955693693,
144.547902361787,145.54184902988,146.535795697974,147.529742366067,147.65485471872),
 .UNSPECIFIED.);
#742=B_SPLINE_CURVE_WITH_KNOTS('',3,(#45845,#45846,#45847,#45848,#45849,
#45850,#45851,#45852,#45853,#45854),.UNSPECIFIED.,.F.,.F.,(4,1,1,1,1,1,
1,4),(141.371669411541,142.234747184304,143.228693852398,144.222640520491,
145.216587188585,146.210533856678,147.204480524772,147.65485471872),
 .UNSPECIFIED.);
#743=B_SPLINE_CURVE_WITH_KNOTS('',3,(#45859,#45860,#45861,#45862,#45863,
#45864,#45865,#45866,#45867,#45868),.UNSPECIFIED.,.F.,.F.,(4,1,1,1,1,1,
1,4),(135.088484104361,135.602382348945,136.596329017039,137.590275685132,
138.584222353226,139.578169021319,140.572115689413,141.371669411541),
 .UNSPECIFIED.);
#744=B_SPLINE_CURVE_WITH_KNOTS('',3,(#45869,#45870,#45871,#45872,#45873,
#45874,#45875,#45876,#45877,#45878,#45879),.UNSPECIFIED.,.F.,.F.,(4,1,1,
1,1,1,1,1,4),(135.088484104361,135.27712050765,136.271067175743,137.265013843837,
138.25896051193,139.252907180024,140.246853848117,141.240800516211,141.371669411541),
 .UNSPECIFIED.);
#745=B_SPLINE_CURVE_WITH_KNOTS('',3,(#45884,#45885,#45886,#45887,#45888,
#45889,#45890,#45891,#45892,#45893),.UNSPECIFIED.,.F.,.F.,(4,1,1,1,1,1,
1,4),(128.805298797182,129.638702340384,130.632649008478,131.626595676571,
132.620542344665,133.614489012758,134.608435680852,135.088484104361),
 .UNSPECIFIED.);
#746=B_SPLINE_CURVE_WITH_KNOTS('',3,(#45894,#45895,#45896,#45897,#45898,
#45899,#45900,#45901,#45902,#45903),.UNSPECIFIED.,.F.,.F.,(4,1,1,1,1,1,
1,4),(128.805298797182,129.313440499089,130.307387167182,131.301333835276,
132.295280503369,133.289227171463,134.283173839556,135.088484104361),
 .UNSPECIFIED.);
#747=B_SPLINE_CURVE_WITH_KNOTS('',3,(#45908,#45909,#45910,#45911,#45912,
#45913,#45914,#45915,#45916,#45917,#45918),.UNSPECIFIED.,.F.,.F.,(4,1,1,
1,1,1,1,1,4),(122.522113490002,122.68107566373,123.675022331823,124.668968999917,
125.66291566801,126.656862336104,127.650809004197,128.644755672291,128.805298797182),
 .UNSPECIFIED.);
#748=B_SPLINE_CURVE_WITH_KNOTS('',3,(#45919,#45920,#45921,#45922,#45923,
#45924,#45925,#45926,#45927,#45928),.UNSPECIFIED.,.F.,.F.,(4,1,1,1,1,1,
1,4),(122.522113490002,123.349760490528,124.343707158621,125.337653826715,
126.331600494808,127.325547162902,128.319493830995,128.805298797182),
 .UNSPECIFIED.);
#749=B_SPLINE_CURVE_WITH_KNOTS('',3,(#45933,#45934,#45935,#45936,#45937,
#45938,#45939,#45940,#45941,#45942),.UNSPECIFIED.,.F.,.F.,(4,1,1,1,1,1,
1,4),(116.238928182822,116.717395655169,117.711342323262,118.705288991356,
119.699235659449,120.693182327543,121.687128995636,122.522113490002),
 .UNSPECIFIED.);
#750=B_SPLINE_CURVE_WITH_KNOTS('',3,(#45943,#45944,#45945,#45946,#45947,
#45948,#45949,#45950,#45951,#45952,#45953),.UNSPECIFIED.,.F.,.F.,(4,1,1,
1,1,1,1,1,4),(116.238928182822,116.392133813873,117.386080481967,118.38002715006,
119.373973818154,120.367920486247,121.361867154341,122.355813822434,122.522113490002),
 .UNSPECIFIED.);
#751=B_SPLINE_CURVE_WITH_KNOTS('',3,(#45958,#45959,#45960,#45961,#45962,
#45963,#45964,#45965,#45966,#45967),.UNSPECIFIED.,.F.,.F.,(4,1,1,1,1,1,
1,4),(109.955742875643,110.753715646608,111.747662314702,112.741608982795,
113.735555650889,114.729502318982,115.723448987075,116.238928182822),
 .UNSPECIFIED.);
#752=B_SPLINE_CURVE_WITH_KNOTS('',3,(#45968,#45969,#45970,#45971,#45972,
#45973,#45974,#45975,#45976,#45977),.UNSPECIFIED.,.F.,.F.,(4,1,1,1,1,1,
1,4),(109.955742875643,110.428453805312,111.422400473406,112.416347141499,
113.410293809593,114.404240477686,115.39818714578,116.238928182822),
 .UNSPECIFIED.);
#753=B_SPLINE_CURVE_WITH_KNOTS('',3,(#45982,#45983,#45984,#45985,#45986,
#45987,#45988,#45989,#45990,#45991,#45992),.UNSPECIFIED.,.F.,.F.,(4,1,1,
1,1,1,1,1,4),(103.672557568463,103.796088969954,104.790035638047,105.783982306141,
106.777928974234,107.771875642328,108.765822310421,109.759768978515,109.955742875643),
 .UNSPECIFIED.);
#754=B_SPLINE_CURVE_WITH_KNOTS('',3,(#45993,#45994,#45995,#45996,#45997,
#45998,#45999,#46000,#46001,#46002),.UNSPECIFIED.,.F.,.F.,(4,1,1,1,1,1,
1,4),(103.672557568463,104.464773796751,105.458720464845,106.452667132938,
107.446613801032,108.440560469125,109.434507137219,109.955742875643),
 .UNSPECIFIED.);
#755=B_SPLINE_CURVE_WITH_KNOTS('',3,(#46007,#46008,#46009,#46010,#46011,
#46012,#46013,#46014,#46015,#46016),.UNSPECIFIED.,.F.,.F.,(4,1,1,1,1,1,
1,4),(97.3893722612836,97.8324089613926,98.8263556294861,99.8203022975796,
100.814248965673,101.808195633767,102.80214230186,103.672557568463),
 .UNSPECIFIED.);
#756=B_SPLINE_CURVE_WITH_KNOTS('',3,(#46017,#46018,#46019,#46020,#46021,
#46022,#46023,#46024,#46025,#46026,#46027),.UNSPECIFIED.,.F.,.F.,(4,1,1,
1,1,1,1,1,4),(97.3893722612836,97.5071471200969,98.5010937881904,99.4950404562839,
100.488987124377,101.482933792471,102.476880460564,103.470827128658,103.672557568463),
 .UNSPECIFIED.);
#757=B_SPLINE_CURVE_WITH_KNOTS('',3,(#46032,#46033,#46034,#46035,#46036,
#46037,#46038,#46039,#46040,#46041),.UNSPECIFIED.,.F.,.F.,(4,1,1,1,1,1,
1,4),(91.106186954104,91.8687289528317,92.8626756209252,93.8566222890186,
94.8505689571121,95.8445156252056,96.8384622932991,97.3893722612836),
 .UNSPECIFIED.);
#758=B_SPLINE_CURVE_WITH_KNOTS('',3,(#46042,#46043,#46044,#46045,#46046,
#46047,#46048,#46049,#46050,#46051),.UNSPECIFIED.,.F.,.F.,(4,1,1,1,1,1,
1,4),(91.106186954104,91.543467111536,92.5374137796295,93.5313604477229,
94.5253071158164,95.5192537839099,96.5132004520034,97.3893722612836),
 .UNSPECIFIED.);
#759=B_SPLINE_CURVE_WITH_KNOTS('',3,(#46056,#46057,#46058,#46059,#46060,
#46061,#46062,#46063,#46064,#46065,#46066),.UNSPECIFIED.,.F.,.F.,(4,1,1,
1,1,1,1,1,4),(84.8230016469245,84.9111022761772,85.9050489442707,86.8989956123642,
87.8929422804577,88.8868889485512,89.8808356166447,90.8747822847382,91.106186954104),
 .UNSPECIFIED.);
#760=B_SPLINE_CURVE_WITH_KNOTS('',3,(#46067,#46068,#46069,#46070,#46071,
#46072,#46073,#46074,#46075,#46076),.UNSPECIFIED.,.F.,.F.,(4,1,1,1,1,1,
1,4),(84.8230016469245,85.579787102975,86.5737337710685,87.567680439162,
88.5616271072555,89.555573775349,90.5495204434425,91.106186954104),
 .UNSPECIFIED.);
#761=B_SPLINE_CURVE_WITH_KNOTS('',3,(#46081,#46082,#46083,#46084,#46085,
#46086,#46087,#46088,#46089,#46090),.UNSPECIFIED.,.F.,.F.,(4,1,1,1,1,1,
1,4),(78.5398163397449,78.9474222676163,79.9413689357097,80.9353156038032,
81.9292622718967,82.9232089399902,83.9171556080837,84.8230016469245),
 .UNSPECIFIED.);
#762=B_SPLINE_CURVE_WITH_KNOTS('',3,(#46091,#46092,#46093,#46094,#46095,
#46096,#46097,#46098,#46099,#46100,#46101),.UNSPECIFIED.,.F.,.F.,(4,1,1,
1,1,1,1,1,4),(78.5398163397449,78.6221604263205,79.616107094414,80.6100537625075,
81.604000430601,82.5979470986945,83.591893766788,84.5858404348815,84.8230016469245),
 .UNSPECIFIED.);
#763=B_SPLINE_CURVE_WITH_KNOTS('',3,(#46106,#46107,#46108,#46109,#46110,
#46111,#46112,#46113,#46114,#46115),.UNSPECIFIED.,.F.,.F.,(4,1,1,1,1,1,
1,4),(72.2566310325653,72.9837422590553,73.9776889271488,74.9716355952423,
75.9655822633358,76.9595289314293,77.9534755995228,78.5398163397449),
 .UNSPECIFIED.);
#764=B_SPLINE_CURVE_WITH_KNOTS('',3,(#46116,#46117,#46118,#46119,#46120,
#46121,#46122,#46123,#46124,#46125),.UNSPECIFIED.,.F.,.F.,(4,1,1,1,1,1,
1,4),(72.2566310325653,72.6584804177596,73.6524270858531,74.6463737539466,
75.6403204220401,76.6342670901336,77.6282137582271,78.5398163397449),
 .UNSPECIFIED.);
#765=B_SPLINE_CURVE_WITH_KNOTS('',3,(#46130,#46131,#46132,#46133,#46134,
#46135,#46136,#46137,#46138,#46139,#46140),.UNSPECIFIED.,.F.,.F.,(4,1,1,
1,1,1,1,1,4),(65.9734457253857,66.0261155824008,67.0200622504943,68.0140089185878,
69.0079555866813,70.0019022547748,70.9958489228683,71.9897955909618,72.2566310325653),
 .UNSPECIFIED.);
#766=B_SPLINE_CURVE_WITH_KNOTS('',3,(#46141,#46142,#46143,#46144,#46145,
#46146,#46147,#46148,#46149,#46150),.UNSPECIFIED.,.F.,.F.,(4,1,1,1,1,1,
1,4),(65.9734457253857,66.6948004091986,67.6887470772921,68.6826937453856,
69.6766404134791,70.6705870815726,71.6645337496661,72.2566310325653),
 .UNSPECIFIED.);
#767=B_SPLINE_CURVE_WITH_KNOTS('',3,(#46155,#46156,#46157,#46158,#46159,
#46160,#46161,#46162,#46163,#46164),.UNSPECIFIED.,.F.,.F.,(4,1,1,1,1,1,
1,4),(59.6902604182061,60.0624355738399,61.0563822419334,62.0503289100269,
63.0442755781204,64.0382222462139,65.0321689143073,65.9734457253857),
 .UNSPECIFIED.);
#768=B_SPLINE_CURVE_WITH_KNOTS('',3,(#46165,#46166,#46167,#46168,#46169,
#46170,#46171,#46172,#46173,#46174,#46175),.UNSPECIFIED.,.F.,.F.,(4,1,1,
1,1,1,1,1,4),(59.6902604182061,59.7371737325442,60.7311204006377,61.7250670687312,
62.7190137368247,63.7129604049182,64.7069070730116,65.7008537411051,65.9734457253857),
 .UNSPECIFIED.);
#769=B_SPLINE_CURVE_WITH_KNOTS('',3,(#46180,#46181,#46182,#46183,#46184,
#46185,#46186,#46187,#46188,#46189),.UNSPECIFIED.,.F.,.F.,(4,1,1,1,1,1,
1,4),(53.4070751110265,54.0987555652789,55.0927022333724,56.0866489014659,
57.0805955695594,58.0745422376529,59.0684889057464,59.6902604182061),
 .UNSPECIFIED.);
#770=B_SPLINE_CURVE_WITH_KNOTS('',3,(#46190,#46191,#46192,#46193,#46194,
#46195,#46196,#46197,#46198,#46199),.UNSPECIFIED.,.F.,.F.,(4,1,1,1,1,1,
1,4),(53.4070751110265,53.7734937239832,54.7674403920767,55.7613870601702,
56.7553337282637,57.7492803963572,58.7432270644507,59.6902604182061),
 .UNSPECIFIED.);
#771=B_SPLINE_CURVE_WITH_KNOTS('',3,(#46204,#46205,#46206,#46207,#46208,
#46209,#46210,#46211,#46212,#46213,#46214),.UNSPECIFIED.,.F.,.F.,(4,1,1,
1,1,1,1,1,4),(47.1238898038469,47.1411288886245,48.135075556718,49.1290222248115,
50.122968892905,51.1169155609985,52.1108622290919,53.1048088971854,53.4070751110265),
 .UNSPECIFIED.);
#772=B_SPLINE_CURVE_WITH_KNOTS('',3,(#46215,#46216,#46217,#46218,#46219,
#46220,#46221,#46222,#46223,#46224),.UNSPECIFIED.,.F.,.F.,(4,1,1,1,1,1,
1,4),(47.1238898038469,47.8098137154223,48.8037603835158,49.7977070516092,
50.7916537197027,51.7856003877962,52.7795470558897,53.4070751110265),
 .UNSPECIFIED.);
#773=B_SPLINE_CURVE_WITH_KNOTS('',3,(#46229,#46230,#46231,#46232,#46233,
#46234,#46235,#46236,#46237,#46238),.UNSPECIFIED.,.F.,.F.,(4,1,1,1,1,1,
1,4),(40.8407044966673,41.1774488800635,42.171395548157,43.1653422162505,
44.159288884344,45.1532355524375,46.147182220531,47.1238898038469),
 .UNSPECIFIED.);
#774=B_SPLINE_CURVE_WITH_KNOTS('',3,(#46239,#46240,#46241,#46242,#46243,
#46244,#46245,#46246,#46247,#46248,#46249),.UNSPECIFIED.,.F.,.F.,(4,1,1,
1,1,1,1,1,4),(40.8407044966673,40.8521870387678,41.8461337068613,42.8400803749548,
43.8340270430483,44.8279737111418,45.8219203792353,46.8158670473288,47.1238898038469),
 .UNSPECIFIED.);
#775=B_SPLINE_CURVE_WITH_KNOTS('',3,(#46254,#46255,#46256,#46257,#46258,
#46259,#46260,#46261,#46262,#46263),.UNSPECIFIED.,.F.,.F.,(4,1,1,1,1,1,
1,4),(34.5575191894877,35.2137688715026,36.2077155395961,37.2016622076895,
38.195608875783,39.1895555438765,40.18350221197,40.8407044966673),
 .UNSPECIFIED.);
#776=B_SPLINE_CURVE_WITH_KNOTS('',3,(#46264,#46265,#46266,#46267,#46268,
#46269,#46270,#46271,#46272,#46273),.UNSPECIFIED.,.F.,.F.,(4,1,1,1,1,1,
1,4),(34.5575191894877,34.8885070302068,35.8824536983003,36.8764003663938,
37.8703470344873,38.8642937025808,39.8582403706743,40.8407044966673),
 .UNSPECIFIED.);
#777=B_SPLINE_CURVE_WITH_KNOTS('',3,(#46278,#46279,#46280,#46281,#46282,
#46283,#46284,#46285,#46286,#46287),.UNSPECIFIED.,.F.,.F.,(4,1,1,1,1,1,
1,4),(28.2743338823081,29.2500888629416,30.2440355310351,31.2379821991286,
32.2319288672221,33.2258755353156,34.2198222034091,34.5575191894877),
 .UNSPECIFIED.);
#778=B_SPLINE_CURVE_WITH_KNOTS('',3,(#46288,#46289,#46290,#46291,#46292,
#46293,#46294,#46295,#46296,#46297),.UNSPECIFIED.,.F.,.F.,(4,1,1,1,1,1,
1,4),(28.2743338823081,28.9248270216459,29.9187736897394,30.9127203578329,
31.9066670259264,32.9006136940199,33.8945603621134,34.5575191894877),
 .UNSPECIFIED.);
#779=B_SPLINE_CURVE_WITH_KNOTS('',3,(#46302,#46303,#46304,#46305,#46306,
#46307,#46308,#46309,#46310,#46311,#46312),.UNSPECIFIED.,.F.,.F.,(4,1,1,
1,1,1,1,1,4),(21.9911485751285,22.2924621862871,23.2864088543806,24.2803555224741,
25.2743021905676,26.2682488586611,27.2621955267546,28.2561421948481,28.2743338823081),
 .UNSPECIFIED.);
#780=B_SPLINE_CURVE_WITH_KNOTS('',3,(#46313,#46314,#46315,#46316,#46317,
#46318,#46319,#46320,#46321,#46322),.UNSPECIFIED.,.F.,.F.,(4,1,1,1,1,1,
1,4),(21.9911485751285,22.9611470130849,23.9550936811784,24.9490403492719,
25.9429870173654,26.9369336854589,27.9308803535524,28.2743338823081),
 .UNSPECIFIED.);
#781=B_SPLINE_CURVE_WITH_KNOTS('',3,(#46329,#46330,#46331,#46332,#46333,
#46334,#46335,#46336,#46337),.UNSPECIFIED.,.F.,.F.,(4,1,1,1,1,1,4),(16.3287821777262,
17.3227288458197,18.3166755139132,19.3106221820067,20.3045688501002,21.2985155181937,
21.9911485751285),.UNSPECIFIED.);
#782=B_SPLINE_CURVE_WITH_KNOTS('',3,(#46338,#46339,#46340,#46341,#46342,
#46343,#46344,#46345,#46346,#46347,#46348),.UNSPECIFIED.,.F.,.F.,(4,1,1,
1,1,1,1,1,4),(15.707963267949,16.0035203364305,16.997467004524,17.9914136726175,
18.9853603407109,19.9793070088044,20.9732536768979,21.9672003449914,21.9911485751285),
 .UNSPECIFIED.);
#783=B_SPLINE_CURVE_WITH_KNOTS('',3,(#46351,#46352,#46353,#46354,#46355,
#46356,#46357,#46358,#46359,#46360,#46361,#46362,#46363,#46364,#46365,#46366,
#46367,#46368,#46369,#46370,#46371,#46372,#46373,#46374,#46375,#46376,#46377,
#46378,#46379,#46380,#46381,#46382,#46383,#46384,#46385,#46386,#46387,#46388,
#46389,#46390,#46391,#46392,#46393,#46394,#46395,#46396),.UNSPECIFIED.,
 .F.,.F.,(4,3,3,3,3,3,3,3,3,3,3,3,3,3,3,4),(-0.178587760439502,-0.17272415791405,
-0.159234259496745,-0.149955987523703,-0.138284796292971,-0.130233106211232,
-0.109899246057786,-0.100105179624859,-0.091716036524901,-0.0758685250126272,
-0.0664651298683787,-0.049848847401284,-0.0374767593822167,-0.0290667458166763,
-0.00650275602542257,0.),.UNSPECIFIED.);
#784=B_SPLINE_CURVE_WITH_KNOTS('',3,(#46401,#46402,#46403,#46404,#46405,
#46406,#46407,#46408,#46409,#46410,#46411,#46412,#46413,#46414,#46415,#46416,
#46417,#46418,#46419,#46420,#46421,#46422,#46423,#46424,#46425,#46426,#46427,
#46428,#46429,#46430,#46431,#46432,#46433,#46434,#46435,#46436,#46437,#46438,
#46439,#46440,#46441,#46442,#46443,#46444,#46445,#46446),.UNSPECIFIED.,
 .F.,.F.,(4,3,3,3,3,3,3,3,3,3,3,3,3,3,3,4),(-0.177567088092129,-0.170082240150724,
-0.15457601521052,-0.145395130014627,-0.128168571237308,-0.119335659531165,
-0.0984679221196259,-0.0877800536301027,-0.0797891990001937,-0.0653423149591641,
-0.0553291551848597,-0.0414968663886448,-0.0315265905887463,-0.02445163365906,
-0.00608210383285545,0.),.UNSPECIFIED.);
#785=B_SPLINE_CURVE_WITH_KNOTS('',3,(#47059,#47060,#47061,#47062,#47063,
#47064,#47065,#47066,#47067,#47068,#47069,#47070,#47071,#47072,#47073,#47074,
#47075,#47076,#47077,#47078,#47079,#47080),.UNSPECIFIED.,.F.,.F.,(4,3,3,
3,3,3,3,4),(140.91635969375,141.140426869276,142.13437353737,143.128320205463,
144.122266873557,145.11621354165,146.110160209744,147.026536188002),
 .UNSPECIFIED.);
#786=B_SPLINE_CURVE_WITH_KNOTS('',3,(#47082,#47083,#47084,#47085,#47086,
#47087,#47088,#47089,#47090,#47091,#47092,#47093,#47094,#47095,#47096,#47097,
#47098,#47099,#47100,#47101,#47102,#47103,#47104,#47105,#47106,#47107,#47108,
#47109,#47110,#47111,#47112,#47113,#47114,#47115,#47116,#47117,#47118,#47119,
#47120,#47121,#47122,#47123,#47124,#47125,#47126,#47127),.UNSPECIFIED.,
 .F.,.F.,(4,3,3,3,3,3,3,3,3,3,3,3,3,3,3,4),(-0.178587760439499,-0.172724157914047,
-0.159234256607848,-0.149955988339685,-0.138284793408456,-0.13023310313133,
-0.109899242927986,-0.100105179984139,-0.0917160365248915,-0.0758685219321002,
-0.0664651290585325,-0.0498488467938994,-0.0374767514336811,-0.0290667438409786,
-0.00650275235697207,0.),.UNSPECIFIED.);
#787=B_SPLINE_CURVE_WITH_KNOTS('',3,(#47128,#47129,#47130,#47131),
 .UNSPECIFIED.,.F.,.F.,(4,4),(15.0871443581717,15.707963267949),
 .UNSPECIFIED.);
#788=B_SPLINE_CURVE_WITH_KNOTS('',3,(#47133,#47134,#47135,#47136,#47137,
#47138,#47139,#47140,#47141,#47142,#47143,#47144,#47145,#47146,#47147,#47148,
#47149,#47150,#47151,#47152,#47153,#47154,#47155,#47156,#47157,#47158,#47159,
#47160,#47161,#47162,#47163,#47164,#47165,#47166,#47167,#47168,#47169,#47170,
#47171,#47172,#47173,#47174,#47175,#47176,#47177,#47178),.UNSPECIFIED.,
 .F.,.F.,(4,3,3,3,3,3,3,3,3,3,3,3,3,3,3,4),(-0.177567088092154,-0.170082240150739,
-0.154576013989902,-0.14539512805807,-0.12816855715706,-0.119335657029697,
-0.0984679168567635,-0.0877800538914335,-0.079789199000203,-0.0653423499049758,
-0.0553291540771241,-0.0414968655578431,-0.0315265899871487,-0.0244516335344751,
-0.00608210876879094,0.),.UNSPECIFIED.);
#789=B_SPLINE_CURVE_WITH_KNOTS('',3,(#47793,#47794,#47795,#47796,#47797,
#47798,#47799,#47800,#47801,#47802,#47803,#47804,#47805,#47806,#47807,#47808,
#47809,#47810,#47811),.UNSPECIFIED.,.F.,.F.,(4,3,3,3,3,3,4),(-149.092000214024,
-148.098053545931,-147.104106877837,-146.110160209743,-145.11621354165,
-144.122266873557,-143.892443155353),.UNSPECIFIED.);
#972=SHAPE_REPRESENTATION_RELATIONSHIP('SRR','None',#55120,#992);
#992=ADVANCED_BREP_SHAPE_REPRESENTATION('',(#1032),#54998);
#1012=STYLED_ITEM('',(#55393),#1032);
#1032=MANIFOLD_SOLID_BREP('ISO_4762_M2x10_A2',#24545);
#1266=FACE_BOUND('',#5115,.T.);
#1267=FACE_BOUND('',#5121,.T.);
#1268=FACE_BOUND('',#5123,.T.);
#1678=PLANE('',#26577);
#1679=PLANE('',#26580);
#1680=PLANE('',#26583);
#1681=PLANE('',#26585);
#1682=PLANE('',#26586);
#1683=PLANE('',#26587);
#1684=PLANE('',#26589);
#1685=PLANE('',#26590);
#1686=PLANE('',#26591);
#1687=PLANE('',#26593);
#1688=PLANE('',#26594);
#1689=PLANE('',#26595);
#1690=PLANE('',#26597);
#1691=PLANE('',#26598);
#1692=PLANE('',#26599);
#1693=PLANE('',#26601);
#1694=PLANE('',#26602);
#1695=PLANE('',#26603);
#1696=PLANE('',#26605);
#1697=PLANE('',#26606);
#1698=PLANE('',#26607);
#1699=PLANE('',#26609);
#1700=PLANE('',#26610);
#1701=PLANE('',#26611);
#1702=PLANE('',#26613);
#1703=PLANE('',#26614);
#1704=PLANE('',#26615);
#1705=PLANE('',#26617);
#1706=PLANE('',#26618);
#1707=PLANE('',#26619);
#1708=PLANE('',#26621);
#1709=PLANE('',#26622);
#1710=PLANE('',#26623);
#1711=PLANE('',#26625);
#1712=PLANE('',#26626);
#1713=PLANE('',#26627);
#1714=PLANE('',#26629);
#1715=PLANE('',#26630);
#1716=PLANE('',#26631);
#1717=PLANE('',#26633);
#1718=PLANE('',#26634);
#1719=PLANE('',#26635);
#1720=PLANE('',#26637);
#1721=PLANE('',#26638);
#1722=PLANE('',#26639);
#1723=PLANE('',#26641);
#1724=PLANE('',#26642);
#1725=PLANE('',#26643);
#1726=PLANE('',#26645);
#1727=PLANE('',#26646);
#1728=PLANE('',#26647);
#1729=PLANE('',#26649);
#1730=PLANE('',#26650);
#1731=PLANE('',#26651);
#1732=PLANE('',#26654);
#1733=PLANE('',#26655);
#1734=PLANE('',#26656);
#1735=PLANE('',#26658);
#1736=PLANE('',#26659);
#1737=PLANE('',#26660);
#1738=PLANE('',#26662);
#1739=PLANE('',#26663);
#1740=PLANE('',#26664);
#1741=PLANE('',#26666);
#1742=PLANE('',#26667);
#1743=PLANE('',#26668);
#1744=PLANE('',#26670);
#1745=PLANE('',#26671);
#1746=PLANE('',#26672);
#1747=PLANE('',#26674);
#1748=PLANE('',#26675);
#1749=PLANE('',#26676);
#1750=PLANE('',#26678);
#1751=PLANE('',#26679);
#1752=PLANE('',#26680);
#1753=PLANE('',#26682);
#1754=PLANE('',#26683);
#1755=PLANE('',#26684);
#1756=PLANE('',#26686);
#1757=PLANE('',#26687);
#1758=PLANE('',#26688);
#1759=PLANE('',#26690);
#1760=PLANE('',#26691);
#1761=PLANE('',#26692);
#1762=PLANE('',#26694);
#1763=PLANE('',#26695);
#1764=PLANE('',#26696);
#1765=PLANE('',#26698);
#1766=PLANE('',#26699);
#1767=PLANE('',#26700);
#1768=PLANE('',#26702);
#1769=PLANE('',#26703);
#1770=PLANE('',#26704);
#1771=PLANE('',#26706);
#1772=PLANE('',#26707);
#1773=PLANE('',#26708);
#1774=PLANE('',#26710);
#1775=PLANE('',#26711);
#1776=PLANE('',#26712);
#1777=PLANE('',#26714);
#1778=PLANE('',#26715);
#1779=PLANE('',#26716);
#1780=PLANE('',#26718);
#1781=PLANE('',#26719);
#1782=PLANE('',#26720);
#1783=PLANE('',#26722);
#1784=PLANE('',#26723);
#1785=PLANE('',#26763);
#1786=PLANE('',#26764);
#1787=PLANE('',#26765);
#1788=PLANE('',#26770);
#1789=PLANE('',#26771);
#1790=PLANE('',#26772);
#1791=PLANE('',#26773);
#1792=PLANE('',#26774);
#1793=PLANE('',#26775);
#1794=PLANE('',#26776);
#1795=PLANE('',#26777);
#1796=PLANE('',#26784);
#1797=PLANE('',#26785);
#2281=CYLINDRICAL_SURFACE('',#26525,0.096675);
#2282=CYLINDRICAL_SURFACE('',#26529,0.096675);
#2283=CYLINDRICAL_SURFACE('',#26530,0.096675);
#2284=CYLINDRICAL_SURFACE('',#26531,0.096675);
#2285=CYLINDRICAL_SURFACE('',#26532,0.096675);
#2286=CYLINDRICAL_SURFACE('',#26533,0.096675);
#2287=CYLINDRICAL_SURFACE('',#26534,0.096675);
#2288=CYLINDRICAL_SURFACE('',#26535,0.096675);
#2289=CYLINDRICAL_SURFACE('',#26536,0.096675);
#2290=CYLINDRICAL_SURFACE('',#26537,0.096675);
#2291=CYLINDRICAL_SURFACE('',#26538,0.096675);
#2292=CYLINDRICAL_SURFACE('',#26539,0.096675);
#2293=CYLINDRICAL_SURFACE('',#26540,0.096675);
#2294=CYLINDRICAL_SURFACE('',#26541,0.096675);
#2295=CYLINDRICAL_SURFACE('',#26542,0.096675);
#2296=CYLINDRICAL_SURFACE('',#26543,0.096675);
#2297=CYLINDRICAL_SURFACE('',#26544,0.096675);
#2298=CYLINDRICAL_SURFACE('',#26545,0.096675);
#2299=CYLINDRICAL_SURFACE('',#26546,0.096675);
#2300=CYLINDRICAL_SURFACE('',#26547,0.096675);
#2301=CYLINDRICAL_SURFACE('',#26548,0.096675);
#2302=CYLINDRICAL_SURFACE('',#26549,0.096675);
#2303=CYLINDRICAL_SURFACE('',#26550,0.096675);
#2304=CYLINDRICAL_SURFACE('',#26551,0.0739);
#2305=CYLINDRICAL_SURFACE('',#26553,0.0739);
#2306=CYLINDRICAL_SURFACE('',#26554,0.0739);
#2307=CYLINDRICAL_SURFACE('',#26555,0.0739);
#2308=CYLINDRICAL_SURFACE('',#26556,0.0739);
#2309=CYLINDRICAL_SURFACE('',#26557,0.0739);
#2310=CYLINDRICAL_SURFACE('',#26558,0.0739);
#2311=CYLINDRICAL_SURFACE('',#26559,0.0739);
#2312=CYLINDRICAL_SURFACE('',#26560,0.0739);
#2313=CYLINDRICAL_SURFACE('',#26561,0.0739);
#2314=CYLINDRICAL_SURFACE('',#26562,0.0739);
#2315=CYLINDRICAL_SURFACE('',#26563,0.0739);
#2316=CYLINDRICAL_SURFACE('',#26564,0.0739);
#2317=CYLINDRICAL_SURFACE('',#26565,0.0739);
#2318=CYLINDRICAL_SURFACE('',#26566,0.0739);
#2319=CYLINDRICAL_SURFACE('',#26567,0.0739);
#2320=CYLINDRICAL_SURFACE('',#26568,0.0739);
#2321=CYLINDRICAL_SURFACE('',#26569,0.0739);
#2322=CYLINDRICAL_SURFACE('',#26570,0.0739);
#2323=CYLINDRICAL_SURFACE('',#26571,0.0739);
#2324=CYLINDRICAL_SURFACE('',#26572,0.0739);
#2325=CYLINDRICAL_SURFACE('',#26573,0.0739);
#2326=CYLINDRICAL_SURFACE('',#26574,0.0739);
#2327=CYLINDRICAL_SURFACE('',#26575,0.0739);
#2328=CYLINDRICAL_SURFACE('',#26582,0.0739);
#2329=CYLINDRICAL_SURFACE('',#26724,0.19);
#2330=CYLINDRICAL_SURFACE('',#26780,0.096675);
#3351=FACE_OUTER_BOUND('',#4945,.T.);
#3352=FACE_OUTER_BOUND('',#4946,.T.);
#3353=FACE_OUTER_BOUND('',#4947,.T.);
#3354=FACE_OUTER_BOUND('',#4948,.T.);
#3355=FACE_OUTER_BOUND('',#4949,.T.);
#3356=FACE_OUTER_BOUND('',#4950,.T.);
#3357=FACE_OUTER_BOUND('',#4951,.T.);
#3358=FACE_OUTER_BOUND('',#4952,.T.);
#3359=FACE_OUTER_BOUND('',#4953,.T.);
#3360=FACE_OUTER_BOUND('',#4954,.T.);
#3361=FACE_OUTER_BOUND('',#4955,.T.);
#3362=FACE_OUTER_BOUND('',#4956,.T.);
#3363=FACE_OUTER_BOUND('',#4957,.T.);
#3364=FACE_OUTER_BOUND('',#4958,.T.);
#3365=FACE_OUTER_BOUND('',#4959,.T.);
#3366=FACE_OUTER_BOUND('',#4960,.T.);
#3367=FACE_OUTER_BOUND('',#4961,.T.);
#3368=FACE_OUTER_BOUND('',#4962,.T.);
#3369=FACE_OUTER_BOUND('',#4963,.T.);
#3370=FACE_OUTER_BOUND('',#4964,.T.);
#3371=FACE_OUTER_BOUND('',#4965,.T.);
#3372=FACE_OUTER_BOUND('',#4966,.T.);
#3373=FACE_OUTER_BOUND('',#4967,.T.);
#3374=FACE_OUTER_BOUND('',#4968,.T.);
#3375=FACE_OUTER_BOUND('',#4969,.T.);
#3376=FACE_OUTER_BOUND('',#4970,.T.);
#3377=FACE_OUTER_BOUND('',#4971,.T.);
#3378=FACE_OUTER_BOUND('',#4972,.T.);
#3379=FACE_OUTER_BOUND('',#4973,.T.);
#3380=FACE_OUTER_BOUND('',#4974,.T.);
#3381=FACE_OUTER_BOUND('',#4975,.T.);
#3382=FACE_OUTER_BOUND('',#4976,.T.);
#3383=FACE_OUTER_BOUND('',#4977,.T.);
#3384=FACE_OUTER_BOUND('',#4978,.T.);
#3385=FACE_OUTER_BOUND('',#4979,.T.);
#3386=FACE_OUTER_BOUND('',#4980,.T.);
#3387=FACE_OUTER_BOUND('',#4981,.T.);
#3388=FACE_OUTER_BOUND('',#4982,.T.);
#3389=FACE_OUTER_BOUND('',#4983,.T.);
#3390=FACE_OUTER_BOUND('',#4984,.T.);
#3391=FACE_OUTER_BOUND('',#4985,.T.);
#3392=FACE_OUTER_BOUND('',#4986,.T.);
#3393=FACE_OUTER_BOUND('',#4987,.T.);
#3394=FACE_OUTER_BOUND('',#4988,.T.);
#3395=FACE_OUTER_BOUND('',#4989,.T.);
#3396=FACE_OUTER_BOUND('',#4990,.T.);
#3397=FACE_OUTER_BOUND('',#4991,.T.);
#3398=FACE_OUTER_BOUND('',#4992,.T.);
#3399=FACE_OUTER_BOUND('',#4993,.T.);
#3400=FACE_OUTER_BOUND('',#4994,.T.);
#3401=FACE_OUTER_BOUND('',#4995,.T.);
#3402=FACE_OUTER_BOUND('',#4996,.T.);
#3403=FACE_OUTER_BOUND('',#4997,.T.);
#3404=FACE_OUTER_BOUND('',#4998,.T.);
#3405=FACE_OUTER_BOUND('',#4999,.T.);
#3406=FACE_OUTER_BOUND('',#5000,.T.);
#3407=FACE_OUTER_BOUND('',#5001,.T.);
#3408=FACE_OUTER_BOUND('',#5002,.T.);
#3409=FACE_OUTER_BOUND('',#5003,.T.);
#3410=FACE_OUTER_BOUND('',#5004,.T.);
#3411=FACE_OUTER_BOUND('',#5005,.T.);
#3412=FACE_OUTER_BOUND('',#5006,.T.);
#3413=FACE_OUTER_BOUND('',#5007,.T.);
#3414=FACE_OUTER_BOUND('',#5008,.T.);
#3415=FACE_OUTER_BOUND('',#5009,.T.);
#3416=FACE_OUTER_BOUND('',#5010,.T.);
#3417=FACE_OUTER_BOUND('',#5011,.T.);
#3418=FACE_OUTER_BOUND('',#5012,.T.);
#3419=FACE_OUTER_BOUND('',#5013,.T.);
#3420=FACE_OUTER_BOUND('',#5014,.T.);
#3421=FACE_OUTER_BOUND('',#5015,.T.);
#3422=FACE_OUTER_BOUND('',#5016,.T.);
#3423=FACE_OUTER_BOUND('',#5017,.T.);
#3424=FACE_OUTER_BOUND('',#5018,.T.);
#3425=FACE_OUTER_BOUND('',#5019,.T.);
#3426=FACE_OUTER_BOUND('',#5020,.T.);
#3427=FACE_OUTER_BOUND('',#5021,.T.);
#3428=FACE_OUTER_BOUND('',#5022,.T.);
#3429=FACE_OUTER_BOUND('',#5023,.T.);
#3430=FACE_OUTER_BOUND('',#5024,.T.);
#3431=FACE_OUTER_BOUND('',#5025,.T.);
#3432=FACE_OUTER_BOUND('',#5026,.T.);
#3433=FACE_OUTER_BOUND('',#5027,.T.);
#3434=FACE_OUTER_BOUND('',#5028,.T.);
#3435=FACE_OUTER_BOUND('',#5029,.T.);
#3436=FACE_OUTER_BOUND('',#5030,.T.);
#3437=FACE_OUTER_BOUND('',#5031,.T.);
#3438=FACE_OUTER_BOUND('',#5032,.T.);
#3439=FACE_OUTER_BOUND('',#5033,.T.);
#3440=FACE_OUTER_BOUND('',#5034,.T.);
#3441=FACE_OUTER_BOUND('',#5035,.T.);
#3442=FACE_OUTER_BOUND('',#5036,.T.);
#3443=FACE_OUTER_BOUND('',#5037,.T.);
#3444=FACE_OUTER_BOUND('',#5038,.T.);
#3445=FACE_OUTER_BOUND('',#5039,.T.);
#3446=FACE_OUTER_BOUND('',#5040,.T.);
#3447=FACE_OUTER_BOUND('',#5041,.T.);
#3448=FACE_OUTER_BOUND('',#5042,.T.);
#3449=FACE_OUTER_BOUND('',#5043,.T.);
#3450=FACE_OUTER_BOUND('',#5044,.T.);
#3451=FACE_OUTER_BOUND('',#5045,.T.);
#3452=FACE_OUTER_BOUND('',#5046,.T.);
#3453=FACE_OUTER_BOUND('',#5047,.T.);
#3454=FACE_OUTER_BOUND('',#5048,.T.);
#3455=FACE_OUTER_BOUND('',#5049,.T.);
#3456=FACE_OUTER_BOUND('',#5050,.T.);
#3457=FACE_OUTER_BOUND('',#5051,.T.);
#3458=FACE_OUTER_BOUND('',#5052,.T.);
#3459=FACE_OUTER_BOUND('',#5053,.T.);
#3460=FACE_OUTER_BOUND('',#5054,.T.);
#3461=FACE_OUTER_BOUND('',#5055,.T.);
#3462=FACE_OUTER_BOUND('',#5056,.T.);
#3463=FACE_OUTER_BOUND('',#5057,.T.);
#3464=FACE_OUTER_BOUND('',#5058,.T.);
#3465=FACE_OUTER_BOUND('',#5059,.T.);
#3466=FACE_OUTER_BOUND('',#5060,.T.);
#3467=FACE_OUTER_BOUND('',#5061,.T.);
#3468=FACE_OUTER_BOUND('',#5062,.T.);
#3469=FACE_OUTER_BOUND('',#5063,.T.);
#3470=FACE_OUTER_BOUND('',#5064,.T.);
#3471=FACE_OUTER_BOUND('',#5065,.T.);
#3472=FACE_OUTER_BOUND('',#5066,.T.);
#3473=FACE_OUTER_BOUND('',#5067,.T.);
#3474=FACE_OUTER_BOUND('',#5068,.T.);
#3475=FACE_OUTER_BOUND('',#5069,.T.);
#3476=FACE_OUTER_BOUND('',#5070,.T.);
#3477=FACE_OUTER_BOUND('',#5071,.T.);
#3478=FACE_OUTER_BOUND('',#5072,.T.);
#3479=FACE_OUTER_BOUND('',#5073,.T.);
#3480=FACE_OUTER_BOUND('',#5074,.T.);
#3481=FACE_OUTER_BOUND('',#5075,.T.);
#3482=FACE_OUTER_BOUND('',#5076,.T.);
#3483=FACE_OUTER_BOUND('',#5077,.T.);
#3484=FACE_OUTER_BOUND('',#5078,.T.);
#3485=FACE_OUTER_BOUND('',#5079,.T.);
#3486=FACE_OUTER_BOUND('',#5080,.T.);
#3487=FACE_OUTER_BOUND('',#5081,.T.);
#3488=FACE_OUTER_BOUND('',#5082,.T.);
#3489=FACE_OUTER_BOUND('',#5083,.T.);
#3490=FACE_OUTER_BOUND('',#5084,.T.);
#3491=FACE_OUTER_BOUND('',#5085,.T.);
#3492=FACE_OUTER_BOUND('',#5086,.T.);
#3493=FACE_OUTER_BOUND('',#5087,.T.);
#3494=FACE_OUTER_BOUND('',#5088,.T.);
#3495=FACE_OUTER_BOUND('',#5089,.T.);
#3496=FACE_OUTER_BOUND('',#5090,.T.);
#3497=FACE_OUTER_BOUND('',#5091,.T.);
#3498=FACE_OUTER_BOUND('',#5092,.T.);
#3499=FACE_OUTER_BOUND('',#5093,.T.);
#3500=FACE_OUTER_BOUND('',#5094,.T.);
#3501=FACE_OUTER_BOUND('',#5095,.T.);
#3502=FACE_OUTER_BOUND('',#5096,.T.);
#3503=FACE_OUTER_BOUND('',#5097,.T.);
#3504=FACE_OUTER_BOUND('',#5098,.T.);
#3505=FACE_OUTER_BOUND('',#5099,.T.);
#3506=FACE_OUTER_BOUND('',#5100,.T.);
#3507=FACE_OUTER_BOUND('',#5101,.T.);
#3508=FACE_OUTER_BOUND('',#5102,.T.);
#3509=FACE_OUTER_BOUND('',#5103,.T.);
#3510=FACE_OUTER_BOUND('',#5104,.T.);
#3511=FACE_OUTER_BOUND('',#5105,.T.);
#3512=FACE_OUTER_BOUND('',#5106,.T.);
#3513=FACE_OUTER_BOUND('',#5107,.T.);
#3514=FACE_OUTER_BOUND('',#5108,.T.);
#3515=FACE_OUTER_BOUND('',#5109,.T.);
#3516=FACE_OUTER_BOUND('',#5110,.T.);
#3517=FACE_OUTER_BOUND('',#5111,.T.);
#3518=FACE_OUTER_BOUND('',#5112,.T.);
#3519=FACE_OUTER_BOUND('',#5113,.T.);
#3520=FACE_OUTER_BOUND('',#5114,.T.);
#3521=FACE_OUTER_BOUND('',#5116,.T.);
#3522=FACE_OUTER_BOUND('',#5117,.T.);
#3523=FACE_OUTER_BOUND('',#5118,.T.);
#3524=FACE_OUTER_BOUND('',#5119,.T.);
#3525=FACE_OUTER_BOUND('',#5120,.T.);
#3526=FACE_OUTER_BOUND('',#5122,.T.);
#4945=EDGE_LOOP('',(#20530,#20531,#20532,#20533,#20534,#20535,#20536,#20537));
#4946=EDGE_LOOP('',(#20538,#20539,#20540,#20541));
#4947=EDGE_LOOP('',(#20542,#20543,#20544,#20545));
#4948=EDGE_LOOP('',(#20546,#20547,#20548,#20549));
#4949=EDGE_LOOP('',(#20550,#20551,#20552,#20553));
#4950=EDGE_LOOP('',(#20554,#20555,#20556,#20557));
#4951=EDGE_LOOP('',(#20558,#20559,#20560,#20561));
#4952=EDGE_LOOP('',(#20562,#20563,#20564,#20565));
#4953=EDGE_LOOP('',(#20566,#20567,#20568,#20569));
#4954=EDGE_LOOP('',(#20570,#20571,#20572,#20573));
#4955=EDGE_LOOP('',(#20574,#20575,#20576,#20577));
#4956=EDGE_LOOP('',(#20578,#20579,#20580,#20581));
#4957=EDGE_LOOP('',(#20582,#20583,#20584,#20585));
#4958=EDGE_LOOP('',(#20586,#20587,#20588,#20589));
#4959=EDGE_LOOP('',(#20590,#20591,#20592,#20593));
#4960=EDGE_LOOP('',(#20594,#20595,#20596,#20597));
#4961=EDGE_LOOP('',(#20598,#20599,#20600,#20601));
#4962=EDGE_LOOP('',(#20602,#20603,#20604,#20605));
#4963=EDGE_LOOP('',(#20606,#20607,#20608,#20609));
#4964=EDGE_LOOP('',(#20610,#20611,#20612,#20613));
#4965=EDGE_LOOP('',(#20614,#20615,#20616,#20617));
#4966=EDGE_LOOP('',(#20618,#20619,#20620,#20621));
#4967=EDGE_LOOP('',(#20622,#20623,#20624,#20625));
#4968=EDGE_LOOP('',(#20626,#20627,#20628,#20629));
#4969=EDGE_LOOP('',(#20630,#20631,#20632,#20633));
#4970=EDGE_LOOP('',(#20634,#20635,#20636,#20637));
#4971=EDGE_LOOP('',(#20638,#20639,#20640,#20641));
#4972=EDGE_LOOP('',(#20642,#20643,#20644,#20645));
#4973=EDGE_LOOP('',(#20646,#20647,#20648,#20649));
#4974=EDGE_LOOP('',(#20650,#20651,#20652,#20653));
#4975=EDGE_LOOP('',(#20654,#20655,#20656,#20657));
#4976=EDGE_LOOP('',(#20658,#20659,#20660,#20661));
#4977=EDGE_LOOP('',(#20662,#20663,#20664,#20665));
#4978=EDGE_LOOP('',(#20666,#20667,#20668,#20669));
#4979=EDGE_LOOP('',(#20670,#20671,#20672,#20673));
#4980=EDGE_LOOP('',(#20674,#20675,#20676,#20677));
#4981=EDGE_LOOP('',(#20678,#20679,#20680,#20681));
#4982=EDGE_LOOP('',(#20682,#20683,#20684,#20685));
#4983=EDGE_LOOP('',(#20686,#20687,#20688,#20689));
#4984=EDGE_LOOP('',(#20690,#20691,#20692,#20693));
#4985=EDGE_LOOP('',(#20694,#20695,#20696,#20697));
#4986=EDGE_LOOP('',(#20698,#20699,#20700,#20701));
#4987=EDGE_LOOP('',(#20702,#20703,#20704,#20705));
#4988=EDGE_LOOP('',(#20706,#20707,#20708,#20709));
#4989=EDGE_LOOP('',(#20710,#20711,#20712,#20713));
#4990=EDGE_LOOP('',(#20714,#20715,#20716,#20717));
#4991=EDGE_LOOP('',(#20718,#20719,#20720,#20721,#20722));
#4992=EDGE_LOOP('',(#20723,#20724,#20725,#20726,#20727));
#4993=EDGE_LOOP('',(#20728,#20729,#20730,#20731,#20732,#20733,#20734,#20735,
#20736,#20737,#20738,#20739,#20740,#20741,#20742,#20743,#20744,#20745,#20746,
#20747,#20748,#20749,#20750,#20751,#20752,#20753,#20754,#20755,#20756,#20757,
#20758,#20759,#20760,#20761,#20762,#20763,#20764,#20765,#20766,#20767,#20768,
#20769,#20770,#20771,#20772,#20773,#20774,#20775,#20776,#20777,#20778));
#4994=EDGE_LOOP('',(#20779,#20780,#20781,#20782,#20783,#20784));
#4995=EDGE_LOOP('',(#20785,#20786,#20787));
#4996=EDGE_LOOP('',(#20788,#20789,#20790,#20791,#20792,#20793,#20794,#20795,
#20796,#20797,#20798,#20799,#20800,#20801,#20802,#20803,#20804,#20805,#20806,
#20807,#20808,#20809,#20810,#20811,#20812,#20813,#20814,#20815,#20816,#20817,
#20818,#20819,#20820,#20821,#20822,#20823,#20824,#20825,#20826,#20827,#20828,
#20829,#20830,#20831,#20832,#20833,#20834,#20835,#20836,#20837));
#4997=EDGE_LOOP('',(#20838,#20839,#20840));
#4998=EDGE_LOOP('',(#20841,#20842,#20843,#20844));
#4999=EDGE_LOOP('',(#20845,#20846,#20847,#20848));
#5000=EDGE_LOOP('',(#20849,#20850,#20851));
#5001=EDGE_LOOP('',(#20852,#20853,#20854,#20855));
#5002=EDGE_LOOP('',(#20856,#20857,#20858,#20859));
#5003=EDGE_LOOP('',(#20860,#20861,#20862));
#5004=EDGE_LOOP('',(#20863,#20864,#20865,#20866));
#5005=EDGE_LOOP('',(#20867,#20868,#20869,#20870));
#5006=EDGE_LOOP('',(#20871,#20872,#20873));
#5007=EDGE_LOOP('',(#20874,#20875,#20876,#20877));
#5008=EDGE_LOOP('',(#20878,#20879,#20880,#20881));
#5009=EDGE_LOOP('',(#20882,#20883,#20884));
#5010=EDGE_LOOP('',(#20885,#20886,#20887,#20888));
#5011=EDGE_LOOP('',(#20889,#20890,#20891,#20892));
#5012=EDGE_LOOP('',(#20893,#20894,#20895));
#5013=EDGE_LOOP('',(#20896,#20897,#20898,#20899));
#5014=EDGE_LOOP('',(#20900,#20901,#20902,#20903));
#5015=EDGE_LOOP('',(#20904,#20905,#20906));
#5016=EDGE_LOOP('',(#20907,#20908,#20909,#20910));
#5017=EDGE_LOOP('',(#20911,#20912,#20913,#20914));
#5018=EDGE_LOOP('',(#20915,#20916,#20917));
#5019=EDGE_LOOP('',(#20918,#20919,#20920,#20921));
#5020=EDGE_LOOP('',(#20922,#20923,#20924,#20925));
#5021=EDGE_LOOP('',(#20926,#20927,#20928));
#5022=EDGE_LOOP('',(#20929,#20930,#20931,#20932));
#5023=EDGE_LOOP('',(#20933,#20934,#20935,#20936));
#5024=EDGE_LOOP('',(#20937,#20938,#20939));
#5025=EDGE_LOOP('',(#20940,#20941,#20942,#20943));
#5026=EDGE_LOOP('',(#20944,#20945,#20946,#20947));
#5027=EDGE_LOOP('',(#20948,#20949,#20950));
#5028=EDGE_LOOP('',(#20951,#20952,#20953,#20954));
#5029=EDGE_LOOP('',(#20955,#20956,#20957,#20958));
#5030=EDGE_LOOP('',(#20959,#20960,#20961));
#5031=EDGE_LOOP('',(#20962,#20963,#20964,#20965));
#5032=EDGE_LOOP('',(#20966,#20967,#20968,#20969));
#5033=EDGE_LOOP('',(#20970,#20971,#20972));
#5034=EDGE_LOOP('',(#20973,#20974,#20975,#20976));
#5035=EDGE_LOOP('',(#20977,#20978,#20979,#20980));
#5036=EDGE_LOOP('',(#20981,#20982,#20983));
#5037=EDGE_LOOP('',(#20984,#20985,#20986,#20987));
#5038=EDGE_LOOP('',(#20988,#20989,#20990,#20991));
#5039=EDGE_LOOP('',(#20992,#20993,#20994));
#5040=EDGE_LOOP('',(#20995,#20996,#20997,#20998));
#5041=EDGE_LOOP('',(#20999,#21000,#21001,#21002));
#5042=EDGE_LOOP('',(#21003,#21004,#21005));
#5043=EDGE_LOOP('',(#21006,#21007,#21008,#21009));
#5044=EDGE_LOOP('',(#21010,#21011,#21012,#21013));
#5045=EDGE_LOOP('',(#21014,#21015,#21016));
#5046=EDGE_LOOP('',(#21017,#21018,#21019,#21020));
#5047=EDGE_LOOP('',(#21021,#21022,#21023,#21024));
#5048=EDGE_LOOP('',(#21025,#21026,#21027,#21028));
#5049=EDGE_LOOP('',(#21029,#21030,#21031,#21032));
#5050=EDGE_LOOP('',(#21033,#21034,#21035,#21036));
#5051=EDGE_LOOP('',(#21037,#21038,#21039));
#5052=EDGE_LOOP('',(#21040,#21041,#21042,#21043));
#5053=EDGE_LOOP('',(#21044,#21045,#21046,#21047));
#5054=EDGE_LOOP('',(#21048,#21049,#21050));
#5055=EDGE_LOOP('',(#21051,#21052,#21053,#21054));
#5056=EDGE_LOOP('',(#21055,#21056,#21057,#21058));
#5057=EDGE_LOOP('',(#21059,#21060,#21061));
#5058=EDGE_LOOP('',(#21062,#21063,#21064,#21065));
#5059=EDGE_LOOP('',(#21066,#21067,#21068,#21069));
#5060=EDGE_LOOP('',(#21070,#21071,#21072));
#5061=EDGE_LOOP('',(#21073,#21074,#21075,#21076));
#5062=EDGE_LOOP('',(#21077,#21078,#21079,#21080));
#5063=EDGE_LOOP('',(#21081,#21082,#21083));
#5064=EDGE_LOOP('',(#21084,#21085,#21086,#21087));
#5065=EDGE_LOOP('',(#21088,#21089,#21090,#21091));
#5066=EDGE_LOOP('',(#21092,#21093,#21094));
#5067=EDGE_LOOP('',(#21095,#21096,#21097,#21098));
#5068=EDGE_LOOP('',(#21099,#21100,#21101,#21102));
#5069=EDGE_LOOP('',(#21103,#21104,#21105));
#5070=EDGE_LOOP('',(#21106,#21107,#21108,#21109));
#5071=EDGE_LOOP('',(#21110,#21111,#21112,#21113));
#5072=EDGE_LOOP('',(#21114,#21115,#21116));
#5073=EDGE_LOOP('',(#21117,#21118,#21119,#21120));
#5074=EDGE_LOOP('',(#21121,#21122,#21123,#21124));
#5075=EDGE_LOOP('',(#21125,#21126,#21127));
#5076=EDGE_LOOP('',(#21128,#21129,#21130,#21131));
#5077=EDGE_LOOP('',(#21132,#21133,#21134,#21135));
#5078=EDGE_LOOP('',(#21136,#21137,#21138));
#5079=EDGE_LOOP('',(#21139,#21140,#21141,#21142));
#5080=EDGE_LOOP('',(#21143,#21144,#21145,#21146));
#5081=EDGE_LOOP('',(#21147,#21148,#21149));
#5082=EDGE_LOOP('',(#21150,#21151,#21152,#21153));
#5083=EDGE_LOOP('',(#21154,#21155,#21156,#21157));
#5084=EDGE_LOOP('',(#21158,#21159,#21160));
#5085=EDGE_LOOP('',(#21161,#21162,#21163,#21164));
#5086=EDGE_LOOP('',(#21165,#21166,#21167,#21168));
#5087=EDGE_LOOP('',(#21169,#21170,#21171));
#5088=EDGE_LOOP('',(#21172,#21173,#21174,#21175));
#5089=EDGE_LOOP('',(#21176,#21177,#21178,#21179));
#5090=EDGE_LOOP('',(#21180,#21181,#21182));
#5091=EDGE_LOOP('',(#21183,#21184,#21185,#21186));
#5092=EDGE_LOOP('',(#21187,#21188,#21189,#21190));
#5093=EDGE_LOOP('',(#21191,#21192,#21193));
#5094=EDGE_LOOP('',(#21194,#21195,#21196,#21197));
#5095=EDGE_LOOP('',(#21198,#21199,#21200,#21201));
#5096=EDGE_LOOP('',(#21202,#21203,#21204));
#5097=EDGE_LOOP('',(#21205,#21206,#21207,#21208));
#5098=EDGE_LOOP('',(#21209,#21210,#21211,#21212));
#5099=EDGE_LOOP('',(#21213,#21214,#21215));
#5100=EDGE_LOOP('',(#21216,#21217,#21218,#21219));
#5101=EDGE_LOOP('',(#21220,#21221,#21222,#21223));
#5102=EDGE_LOOP('',(#21224,#21225,#21226,#21227,#21228,#21229,#21230,#21231,
#21232,#21233,#21234,#21235,#21236,#21237,#21238,#21239,#21240,#21241,#21242,
#21243,#21244,#21245,#21246,#21247,#21248,#21249,#21250,#21251,#21252,#21253,
#21254,#21255,#21256,#21257,#21258,#21259,#21260,#21261,#21262,#21263,#21264,
#21265,#21266,#21267,#21268,#21269,#21270,#21271,#21272,#21273,#21274,#21275,
#21276,#21277,#21278,#21279,#21280,#21281,#21282,#21283,#21284,#21285,#21286,
#21287,#21288,#21289,#21290,#21291,#21292,#21293,#21294,#21295,#21296,#21297,
#21298,#21299,#21300,#21301,#21302,#21303,#21304,#21305,#21306,#21307,#21308,
#21309,#21310,#21311,#21312,#21313,#21314,#21315,#21316,#21317,#21318,#21319,
#21320,#21321,#21322,#21323,#21324,#21325,#21326,#21327,#21328,#21329,#21330,
#21331,#21332,#21333,#21334,#21335,#21336,#21337,#21338,#21339,#21340,#21341,
#21342,#21343,#21344,#21345,#21346,#21347,#21348,#21349,#21350,#21351,#21352,
#21353,#21354,#21355,#21356,#21357,#21358,#21359,#21360,#21361,#21362,#21363,
#21364,#21365,#21366,#21367,#21368,#21369,#21370,#21371));
#5103=EDGE_LOOP('',(#21372,#21373,#21374,#21375));
#5104=EDGE_LOOP('',(#21376,#21377,#21378,#21379));
#5105=EDGE_LOOP('',(#21380,#21381,#21382));
#5106=EDGE_LOOP('',(#21383,#21384,#21385,#21386,#21387,#21388,#21389,#21390,
#21391,#21392,#21393,#21394,#21395,#21396,#21397,#21398,#21399,#21400,#21401,
#21402,#21403,#21404,#21405,#21406,#21407,#21408,#21409,#21410,#21411,#21412,
#21413,#21414,#21415,#21416,#21417,#21418,#21419,#21420,#21421,#21422,#21423,
#21424,#21425,#21426,#21427,#21428,#21429,#21430,#21431,#21432,#21433,#21434,
#21435,#21436,#21437,#21438,#21439,#21440,#21441,#21442,#21443,#21444,#21445,
#21446,#21447,#21448,#21449,#21450,#21451,#21452,#21453,#21454,#21455,#21456,
#21457,#21458,#21459,#21460,#21461,#21462,#21463,#21464,#21465,#21466,#21467,
#21468,#21469,#21470,#21471,#21472,#21473,#21474,#21475,#21476,#21477,#21478,
#21479,#21480,#21481,#21482,#21483,#21484,#21485,#21486,#21487,#21488,#21489,
#21490,#21491,#21492,#21493));
#5107=EDGE_LOOP('',(#21494,#21495,#21496));
#5108=EDGE_LOOP('',(#21497,#21498,#21499,#21500));
#5109=EDGE_LOOP('',(#21501,#21502,#21503,#21504));
#5110=EDGE_LOOP('',(#21505,#21506,#21507,#21508));
#5111=EDGE_LOOP('',(#21509,#21510,#21511,#21512));
#5112=EDGE_LOOP('',(#21513,#21514,#21515,#21516));
#5113=EDGE_LOOP('',(#21517,#21518,#21519,#21520));
#5114=EDGE_LOOP('',(#21521,#21522,#21523,#21524,#21525,#21526));
#5115=EDGE_LOOP('',(#21527));
#5116=EDGE_LOOP('',(#21528));
#5117=EDGE_LOOP('',(#21529,#21530,#21531,#21532));
#5118=EDGE_LOOP('',(#21533,#21534,#21535,#21536));
#5119=EDGE_LOOP('',(#21537,#21538,#21539,#21540,#21541,#21542));
#5120=EDGE_LOOP('',(#21543));
#5121=EDGE_LOOP('',(#21544));
#5122=EDGE_LOOP('',(#21545));
#5123=EDGE_LOOP('',(#21546,#21547,#21548,#21549,#21550,#21551));
#6594=LINE('',#44632,#8415);
#6595=LINE('',#44650,#8416);
#6596=LINE('',#44667,#8417);
#6597=LINE('',#44721,#8418);
#6598=LINE('',#44769,#8419);
#6599=LINE('',#44817,#8420);
#6600=LINE('',#44865,#8421);
#6601=LINE('',#44919,#8422);
#6602=LINE('',#44967,#8423);
#6603=LINE('',#45015,#8424);
#6604=LINE('',#45069,#8425);
#6605=LINE('',#45117,#8426);
#6606=LINE('',#45165,#8427);
#6607=LINE('',#45219,#8428);
#6608=LINE('',#45267,#8429);
#6609=LINE('',#45315,#8430);
#6610=LINE('',#45369,#8431);
#6611=LINE('',#45417,#8432);
#6612=LINE('',#45465,#8433);
#6613=LINE('',#45519,#8434);
#6614=LINE('',#45567,#8435);
#6615=LINE('',#45615,#8436);
#6616=LINE('',#45669,#8437);
#6617=LINE('',#45717,#8438);
#6618=LINE('',#45765,#8439);
#6619=LINE('',#45784,#8440);
#6620=LINE('',#45809,#8441);
#6621=LINE('',#45833,#8442);
#6622=LINE('',#45858,#8443);
#6623=LINE('',#45883,#8444);
#6624=LINE('',#45907,#8445);
#6625=LINE('',#45932,#8446);
#6626=LINE('',#45957,#8447);
#6627=LINE('',#45981,#8448);
#6628=LINE('',#46006,#8449);
#6629=LINE('',#46031,#8450);
#6630=LINE('',#46055,#8451);
#6631=LINE('',#46080,#8452);
#6632=LINE('',#46105,#8453);
#6633=LINE('',#46129,#8454);
#6634=LINE('',#46154,#8455);
#6635=LINE('',#46179,#8456);
#6636=LINE('',#46203,#8457);
#6637=LINE('',#46228,#8458);
#6638=LINE('',#46253,#8459);
#6639=LINE('',#46277,#8460);
#6640=LINE('',#46301,#8461);
#6641=LINE('',#46326,#8462);
#6642=LINE('',#47817,#8463);
#6643=LINE('',#47818,#8464);
#6644=LINE('',#47821,#8465);
#6645=LINE('',#47823,#8466);
#6646=LINE('',#47829,#8467);
#6647=LINE('',#47838,#8468);
#6648=LINE('',#47839,#8469);
#6649=LINE('',#47842,#8470);
#6650=LINE('',#47844,#8471);
#6651=LINE('',#47850,#8472);
#6652=LINE('',#47859,#8473);
#6653=LINE('',#47860,#8474);
#6654=LINE('',#47863,#8475);
#6655=LINE('',#47865,#8476);
#6656=LINE('',#47871,#8477);
#6657=LINE('',#47880,#8478);
#6658=LINE('',#47881,#8479);
#6659=LINE('',#47884,#8480);
#6660=LINE('',#47886,#8481);
#6661=LINE('',#47892,#8482);
#6662=LINE('',#47901,#8483);
#6663=LINE('',#47902,#8484);
#6664=LINE('',#47905,#8485);
#6665=LINE('',#47907,#8486);
#6666=LINE('',#47913,#8487);
#6667=LINE('',#47922,#8488);
#6668=LINE('',#47923,#8489);
#6669=LINE('',#47926,#8490);
#6670=LINE('',#47928,#8491);
#6671=LINE('',#47934,#8492);
#6672=LINE('',#47943,#8493);
#6673=LINE('',#47944,#8494);
#6674=LINE('',#47947,#8495);
#6675=LINE('',#47949,#8496);
#6676=LINE('',#47955,#8497);
#6677=LINE('',#47964,#8498);
#6678=LINE('',#47965,#8499);
#6679=LINE('',#47968,#8500);
#6680=LINE('',#47970,#8501);
#6681=LINE('',#47976,#8502);
#6682=LINE('',#47985,#8503);
#6683=LINE('',#47986,#8504);
#6684=LINE('',#47989,#8505);
#6685=LINE('',#47991,#8506);
#6686=LINE('',#47997,#8507);
#6687=LINE('',#48006,#8508);
#6688=LINE('',#48007,#8509);
#6689=LINE('',#48010,#8510);
#6690=LINE('',#48012,#8511);
#6691=LINE('',#48018,#8512);
#6692=LINE('',#48027,#8513);
#6693=LINE('',#48028,#8514);
#6694=LINE('',#48031,#8515);
#6695=LINE('',#48033,#8516);
#6696=LINE('',#48039,#8517);
#6697=LINE('',#48048,#8518);
#6698=LINE('',#48049,#8519);
#6699=LINE('',#48052,#8520);
#6700=LINE('',#48054,#8521);
#6701=LINE('',#48060,#8522);
#6702=LINE('',#48069,#8523);
#6703=LINE('',#48070,#8524);
#6704=LINE('',#48073,#8525);
#6705=LINE('',#48075,#8526);
#6706=LINE('',#48081,#8527);
#6707=LINE('',#48090,#8528);
#6708=LINE('',#48091,#8529);
#6709=LINE('',#48094,#8530);
#6710=LINE('',#48096,#8531);
#6711=LINE('',#48102,#8532);
#6712=LINE('',#48111,#8533);
#6713=LINE('',#48112,#8534);
#6714=LINE('',#48115,#8535);
#6715=LINE('',#48117,#8536);
#6716=LINE('',#48123,#8537);
#6717=LINE('',#48132,#8538);
#6718=LINE('',#48133,#8539);
#6719=LINE('',#48136,#8540);
#6720=LINE('',#48138,#8541);
#6721=LINE('',#48144,#8542);
#6722=LINE('',#48153,#8543);
#6723=LINE('',#48154,#8544);
#6724=LINE('',#48157,#8545);
#6725=LINE('',#48159,#8546);
#6726=LINE('',#48165,#8547);
#6727=LINE('',#48174,#8548);
#6728=LINE('',#48176,#8549);
#6729=LINE('',#48180,#8550);
#6730=LINE('',#48182,#8551);
#6731=LINE('',#48188,#8552);
#6732=LINE('',#48197,#8553);
#6733=LINE('',#48198,#8554);
#6734=LINE('',#48201,#8555);
#6735=LINE('',#48203,#8556);
#6736=LINE('',#48209,#8557);
#6737=LINE('',#48218,#8558);
#6738=LINE('',#48219,#8559);
#6739=LINE('',#48222,#8560);
#6740=LINE('',#48224,#8561);
#6741=LINE('',#48230,#8562);
#6742=LINE('',#48239,#8563);
#6743=LINE('',#48240,#8564);
#6744=LINE('',#48243,#8565);
#6745=LINE('',#48245,#8566);
#6746=LINE('',#48251,#8567);
#6747=LINE('',#48260,#8568);
#6748=LINE('',#48261,#8569);
#6749=LINE('',#48264,#8570);
#6750=LINE('',#48266,#8571);
#6751=LINE('',#48272,#8572);
#6752=LINE('',#48281,#8573);
#6753=LINE('',#48282,#8574);
#6754=LINE('',#48285,#8575);
#6755=LINE('',#48287,#8576);
#6756=LINE('',#48293,#8577);
#6757=LINE('',#48302,#8578);
#6758=LINE('',#48303,#8579);
#6759=LINE('',#48306,#8580);
#6760=LINE('',#48308,#8581);
#6761=LINE('',#48314,#8582);
#6762=LINE('',#48323,#8583);
#6763=LINE('',#48324,#8584);
#6764=LINE('',#48327,#8585);
#6765=LINE('',#48329,#8586);
#6766=LINE('',#48335,#8587);
#6767=LINE('',#48344,#8588);
#6768=LINE('',#48345,#8589);
#6769=LINE('',#48348,#8590);
#6770=LINE('',#48350,#8591);
#6771=LINE('',#48356,#8592);
#6772=LINE('',#48365,#8593);
#6773=LINE('',#48366,#8594);
#6774=LINE('',#48369,#8595);
#6775=LINE('',#48371,#8596);
#6776=LINE('',#48377,#8597);
#6777=LINE('',#48386,#8598);
#6778=LINE('',#48387,#8599);
#6779=LINE('',#48390,#8600);
#6780=LINE('',#48392,#8601);
#6781=LINE('',#48398,#8602);
#6782=LINE('',#48407,#8603);
#6783=LINE('',#48408,#8604);
#6784=LINE('',#48411,#8605);
#6785=LINE('',#48413,#8606);
#6786=LINE('',#48419,#8607);
#6787=LINE('',#48428,#8608);
#6788=LINE('',#48429,#8609);
#6789=LINE('',#48432,#8610);
#6790=LINE('',#48434,#8611);
#6791=LINE('',#48440,#8612);
#6792=LINE('',#48449,#8613);
#6793=LINE('',#48450,#8614);
#6794=LINE('',#48453,#8615);
#6795=LINE('',#48455,#8616);
#6796=LINE('',#48461,#8617);
#6797=LINE('',#48470,#8618);
#6798=LINE('',#48471,#8619);
#6799=LINE('',#48474,#8620);
#6800=LINE('',#48476,#8621);
#6801=LINE('',#48482,#8622);
#6802=LINE('',#48491,#8623);
#6803=LINE('',#48492,#8624);
#6804=LINE('',#48495,#8625);
#6805=LINE('',#48497,#8626);
#6806=LINE('',#48503,#8627);
#6807=LINE('',#48512,#8628);
#6808=LINE('',#48513,#8629);
#6809=LINE('',#48516,#8630);
#6810=LINE('',#48518,#8631);
#6811=LINE('',#48524,#8632);
#6812=LINE('',#48533,#8633);
#6813=LINE('',#48534,#8634);
#6814=LINE('',#48537,#8635);
#6815=LINE('',#48539,#8636);
#6816=LINE('',#48545,#8637);
#6817=LINE('',#48568,#8638);
#6818=LINE('',#48590,#8639);
#6819=LINE('',#48594,#8640);
#6820=LINE('',#48598,#8641);
#6821=LINE('',#48600,#8642);
#6822=LINE('',#48608,#8643);
#6823=LINE('',#48613,#8644);
#6824=LINE('',#48617,#8645);
#6825=LINE('',#48622,#8646);
#6826=LINE('',#48624,#8647);
#6827=LINE('',#48626,#8648);
#6828=LINE('',#48627,#8649);
#6829=LINE('',#48630,#8650);
#6830=LINE('',#48632,#8651);
#6831=LINE('',#48633,#8652);
#6832=LINE('',#48636,#8653);
#6833=LINE('',#48638,#8654);
#6834=LINE('',#48639,#8655);
#6835=LINE('',#48642,#8656);
#6836=LINE('',#48644,#8657);
#6837=LINE('',#48645,#8658);
#6838=LINE('',#48648,#8659);
#6839=LINE('',#48650,#8660);
#6840=LINE('',#48651,#8661);
#6841=LINE('',#48653,#8662);
#6842=LINE('',#48654,#8663);
#6843=LINE('',#48660,#8664);
#6844=LINE('',#48666,#8665);
#8415=VECTOR('',#31922,0.1);
#8416=VECTOR('',#31925,0.1);
#8417=VECTOR('',#31932,0.1);
#8418=VECTOR('',#31935,0.1);
#8419=VECTOR('',#31938,0.1);
#8420=VECTOR('',#31941,0.1);
#8421=VECTOR('',#31944,0.1);
#8422=VECTOR('',#31947,0.1);
#8423=VECTOR('',#31950,0.1);
#8424=VECTOR('',#31953,0.1);
#8425=VECTOR('',#31956,0.1);
#8426=VECTOR('',#31959,0.1);
#8427=VECTOR('',#31962,0.1);
#8428=VECTOR('',#31965,0.1);
#8429=VECTOR('',#31968,0.1);
#8430=VECTOR('',#31971,0.1);
#8431=VECTOR('',#31974,0.1);
#8432=VECTOR('',#31977,0.1);
#8433=VECTOR('',#31980,0.1);
#8434=VECTOR('',#31983,0.1);
#8435=VECTOR('',#31986,0.1);
#8436=VECTOR('',#31989,0.1);
#8437=VECTOR('',#31992,0.1);
#8438=VECTOR('',#31995,0.1);
#8439=VECTOR('',#31998,0.0739);
#8440=VECTOR('',#32003,0.0739);
#8441=VECTOR('',#32006,0.0739);
#8442=VECTOR('',#32009,0.0739);
#8443=VECTOR('',#32012,0.0739);
#8444=VECTOR('',#32015,0.0739);
#8445=VECTOR('',#32018,0.0739);
#8446=VECTOR('',#32021,0.0739);
#8447=VECTOR('',#32024,0.0739);
#8448=VECTOR('',#32027,0.0739);
#8449=VECTOR('',#32030,0.0739);
#8450=VECTOR('',#32033,0.0739);
#8451=VECTOR('',#32036,0.0739);
#8452=VECTOR('',#32039,0.0739);
#8453=VECTOR('',#32042,0.0739);
#8454=VECTOR('',#32045,0.0739);
#8455=VECTOR('',#32048,0.0739);
#8456=VECTOR('',#32051,0.0739);
#8457=VECTOR('',#32054,0.0739);
#8458=VECTOR('',#32057,0.0739);
#8459=VECTOR('',#32060,0.0739);
#8460=VECTOR('',#32063,0.0739);
#8461=VECTOR('',#32066,0.0739);
#8462=VECTOR('',#32069,0.0739);
#8463=VECTOR('',#32088,1.);
#8464=VECTOR('',#32089,1.);
#8465=VECTOR('',#32092,1.);
#8466=VECTOR('',#32093,1.);
#8467=VECTOR('',#32096,1.);
#8468=VECTOR('',#32101,1.);
#8469=VECTOR('',#32102,1.);
#8470=VECTOR('',#32105,1.);
#8471=VECTOR('',#32106,1.);
#8472=VECTOR('',#32109,1.);
#8473=VECTOR('',#32114,1.);
#8474=VECTOR('',#32115,1.);
#8475=VECTOR('',#32118,1.);
#8476=VECTOR('',#32119,1.);
#8477=VECTOR('',#32122,1.);
#8478=VECTOR('',#32127,1.);
#8479=VECTOR('',#32128,1.);
#8480=VECTOR('',#32131,1.);
#8481=VECTOR('',#32132,1.);
#8482=VECTOR('',#32135,1.);
#8483=VECTOR('',#32140,1.);
#8484=VECTOR('',#32141,1.);
#8485=VECTOR('',#32144,1.);
#8486=VECTOR('',#32145,1.);
#8487=VECTOR('',#32148,1.);
#8488=VECTOR('',#32153,1.);
#8489=VECTOR('',#32154,1.);
#8490=VECTOR('',#32157,1.);
#8491=VECTOR('',#32158,1.);
#8492=VECTOR('',#32161,1.);
#8493=VECTOR('',#32166,1.);
#8494=VECTOR('',#32167,1.);
#8495=VECTOR('',#32170,1.);
#8496=VECTOR('',#32171,1.);
#8497=VECTOR('',#32174,1.);
#8498=VECTOR('',#32179,1.);
#8499=VECTOR('',#32180,1.);
#8500=VECTOR('',#32183,1.);
#8501=VECTOR('',#32184,1.);
#8502=VECTOR('',#32187,1.);
#8503=VECTOR('',#32192,1.);
#8504=VECTOR('',#32193,1.);
#8505=VECTOR('',#32196,1.);
#8506=VECTOR('',#32197,1.);
#8507=VECTOR('',#32200,1.);
#8508=VECTOR('',#32205,1.);
#8509=VECTOR('',#32206,1.);
#8510=VECTOR('',#32209,1.);
#8511=VECTOR('',#32210,1.);
#8512=VECTOR('',#32213,1.);
#8513=VECTOR('',#32218,1.);
#8514=VECTOR('',#32219,1.);
#8515=VECTOR('',#32222,1.);
#8516=VECTOR('',#32223,1.);
#8517=VECTOR('',#32226,1.);
#8518=VECTOR('',#32231,1.);
#8519=VECTOR('',#32232,1.);
#8520=VECTOR('',#32235,1.);
#8521=VECTOR('',#32236,1.);
#8522=VECTOR('',#32239,1.);
#8523=VECTOR('',#32244,1.);
#8524=VECTOR('',#32245,1.);
#8525=VECTOR('',#32248,1.);
#8526=VECTOR('',#32249,1.);
#8527=VECTOR('',#32252,1.);
#8528=VECTOR('',#32257,1.);
#8529=VECTOR('',#32258,1.);
#8530=VECTOR('',#32261,1.);
#8531=VECTOR('',#32262,1.);
#8532=VECTOR('',#32265,1.);
#8533=VECTOR('',#32270,1.);
#8534=VECTOR('',#32271,1.);
#8535=VECTOR('',#32274,1.);
#8536=VECTOR('',#32275,1.);
#8537=VECTOR('',#32278,1.);
#8538=VECTOR('',#32283,1.);
#8539=VECTOR('',#32284,1.);
#8540=VECTOR('',#32287,1.);
#8541=VECTOR('',#32288,1.);
#8542=VECTOR('',#32291,1.);
#8543=VECTOR('',#32296,1.);
#8544=VECTOR('',#32297,1.);
#8545=VECTOR('',#32300,1.);
#8546=VECTOR('',#32301,1.);
#8547=VECTOR('',#32304,1.);
#8548=VECTOR('',#32309,1.);
#8549=VECTOR('',#32310,1.);
#8550=VECTOR('',#32315,1.);
#8551=VECTOR('',#32316,1.);
#8552=VECTOR('',#32319,1.);
#8553=VECTOR('',#32324,1.);
#8554=VECTOR('',#32325,1.);
#8555=VECTOR('',#32328,1.);
#8556=VECTOR('',#32329,1.);
#8557=VECTOR('',#32332,1.);
#8558=VECTOR('',#32337,1.);
#8559=VECTOR('',#32338,1.);
#8560=VECTOR('',#32341,1.);
#8561=VECTOR('',#32342,1.);
#8562=VECTOR('',#32345,1.);
#8563=VECTOR('',#32350,1.);
#8564=VECTOR('',#32351,1.);
#8565=VECTOR('',#32354,1.);
#8566=VECTOR('',#32355,1.);
#8567=VECTOR('',#32358,1.);
#8568=VECTOR('',#32363,1.);
#8569=VECTOR('',#32364,1.);
#8570=VECTOR('',#32367,1.);
#8571=VECTOR('',#32368,1.);
#8572=VECTOR('',#32371,1.);
#8573=VECTOR('',#32376,1.);
#8574=VECTOR('',#32377,1.);
#8575=VECTOR('',#32380,1.);
#8576=VECTOR('',#32381,1.);
#8577=VECTOR('',#32384,1.);
#8578=VECTOR('',#32389,1.);
#8579=VECTOR('',#32390,1.);
#8580=VECTOR('',#32393,1.);
#8581=VECTOR('',#32394,1.);
#8582=VECTOR('',#32397,1.);
#8583=VECTOR('',#32402,1.);
#8584=VECTOR('',#32403,1.);
#8585=VECTOR('',#32406,1.);
#8586=VECTOR('',#32407,1.);
#8587=VECTOR('',#32410,1.);
#8588=VECTOR('',#32415,1.);
#8589=VECTOR('',#32416,1.);
#8590=VECTOR('',#32419,1.);
#8591=VECTOR('',#32420,1.);
#8592=VECTOR('',#32423,1.);
#8593=VECTOR('',#32428,1.);
#8594=VECTOR('',#32429,1.);
#8595=VECTOR('',#32432,1.);
#8596=VECTOR('',#32433,1.);
#8597=VECTOR('',#32436,1.);
#8598=VECTOR('',#32441,1.);
#8599=VECTOR('',#32442,1.);
#8600=VECTOR('',#32445,1.);
#8601=VECTOR('',#32446,1.);
#8602=VECTOR('',#32449,1.);
#8603=VECTOR('',#32454,1.);
#8604=VECTOR('',#32455,1.);
#8605=VECTOR('',#32458,1.);
#8606=VECTOR('',#32459,1.);
#8607=VECTOR('',#32462,1.);
#8608=VECTOR('',#32467,1.);
#8609=VECTOR('',#32468,1.);
#8610=VECTOR('',#32471,1.);
#8611=VECTOR('',#32472,1.);
#8612=VECTOR('',#32475,1.);
#8613=VECTOR('',#32480,1.);
#8614=VECTOR('',#32481,1.);
#8615=VECTOR('',#32484,1.);
#8616=VECTOR('',#32485,1.);
#8617=VECTOR('',#32488,1.);
#8618=VECTOR('',#32493,1.);
#8619=VECTOR('',#32494,1.);
#8620=VECTOR('',#32497,1.);
#8621=VECTOR('',#32498,1.);
#8622=VECTOR('',#32501,1.);
#8623=VECTOR('',#32506,1.);
#8624=VECTOR('',#32507,1.);
#8625=VECTOR('',#32510,1.);
#8626=VECTOR('',#32511,1.);
#8627=VECTOR('',#32514,1.);
#8628=VECTOR('',#32519,1.);
#8629=VECTOR('',#32520,1.);
#8630=VECTOR('',#32523,1.);
#8631=VECTOR('',#32524,1.);
#8632=VECTOR('',#32527,1.);
#8633=VECTOR('',#32532,1.);
#8634=VECTOR('',#32533,1.);
#8635=VECTOR('',#32536,1.);
#8636=VECTOR('',#32537,1.);
#8637=VECTOR('',#32540,1.);
#8638=VECTOR('',#32577,0.19);
#8639=VECTOR('',#32616,1.);
#8640=VECTOR('',#32619,1.);
#8641=VECTOR('',#32624,1.);
#8642=VECTOR('',#32625,1.);
#8643=VECTOR('',#32628,1.);
#8644=VECTOR('',#32635,0.1825);
#8645=VECTOR('',#32638,0.0346410161513776);
#8646=VECTOR('',#32643,1.);
#8647=VECTOR('',#32644,1.);
#8648=VECTOR('',#32645,1.);
#8649=VECTOR('',#32646,1.);
#8650=VECTOR('',#32649,1.);
#8651=VECTOR('',#32650,1.);
#8652=VECTOR('',#32651,1.);
#8653=VECTOR('',#32654,1.);
#8654=VECTOR('',#32655,1.);
#8655=VECTOR('',#32656,1.);
#8656=VECTOR('',#32659,1.);
#8657=VECTOR('',#32660,1.);
#8658=VECTOR('',#32661,1.);
#8659=VECTOR('',#32664,1.);
#8660=VECTOR('',#32665,1.);
#8661=VECTOR('',#32666,1.);
#8662=VECTOR('',#32669,1.);
#8663=VECTOR('',#32670,1.);
#8664=VECTOR('',#32679,0.088);
#8665=VECTOR('',#32688,0.105);
#9829=CIRCLE('',#26526,0.096675);
#9830=CIRCLE('',#26527,0.096675);
#9831=CIRCLE('',#26528,0.096675);
#9832=CIRCLE('',#26552,0.0739);
#9833=CIRCLE('',#26576,0.0739);
#9834=CIRCLE('',#26578,0.096675);
#9835=CIRCLE('',#26579,0.096675);
#9836=CIRCLE('',#26581,0.0739);
#9837=CIRCLE('',#26584,0.19);
#9838=CIRCLE('',#26588,0.19);
#9839=CIRCLE('',#26592,0.19);
#9840=CIRCLE('',#26596,0.19);
#9841=CIRCLE('',#26600,0.19);
#9842=CIRCLE('',#26604,0.19);
#9843=CIRCLE('',#26608,0.19);
#9844=CIRCLE('',#26612,0.19);
#9845=CIRCLE('',#26616,0.19);
#9846=CIRCLE('',#26620,0.19);
#9847=CIRCLE('',#26624,0.19);
#9848=CIRCLE('',#26628,0.19);
#9849=CIRCLE('',#26632,0.19);
#9850=CIRCLE('',#26636,0.19);
#9851=CIRCLE('',#26640,0.19);
#9852=CIRCLE('',#26644,0.19);
#9853=CIRCLE('',#26648,0.19);
#9854=CIRCLE('',#26652,0.19);
#9855=CIRCLE('',#26653,0.19);
#9856=CIRCLE('',#26657,0.19);
#9857=CIRCLE('',#26661,0.19);
#9858=CIRCLE('',#26665,0.19);
#9859=CIRCLE('',#26669,0.19);
#9860=CIRCLE('',#26673,0.19);
#9861=CIRCLE('',#26677,0.19);
#9862=CIRCLE('',#26681,0.19);
#9863=CIRCLE('',#26685,0.19);
#9864=CIRCLE('',#26689,0.19);
#9865=CIRCLE('',#26693,0.19);
#9866=CIRCLE('',#26697,0.19);
#9867=CIRCLE('',#26701,0.19);
#9868=CIRCLE('',#26705,0.19);
#9869=CIRCLE('',#26709,0.19);
#9870=CIRCLE('',#26713,0.19);
#9871=CIRCLE('',#26717,0.19);
#9872=CIRCLE('',#26721,0.19);
#9873=CIRCLE('',#26725,0.19);
#9874=CIRCLE('',#26726,0.19);
#9875=CIRCLE('',#26727,0.19);
#9876=CIRCLE('',#26728,0.19);
#9877=CIRCLE('',#26729,0.19);
#9878=CIRCLE('',#26730,0.19);
#9879=CIRCLE('',#26731,0.19);
#9880=CIRCLE('',#26732,0.19);
#9881=CIRCLE('',#26733,0.19);
#9882=CIRCLE('',#26734,0.19);
#9883=CIRCLE('',#26735,0.19);
#9884=CIRCLE('',#26736,0.19);
#9885=CIRCLE('',#26737,0.19);
#9886=CIRCLE('',#26738,0.19);
#9887=CIRCLE('',#26739,0.19);
#9888=CIRCLE('',#26740,0.19);
#9889=CIRCLE('',#26741,0.19);
#9890=CIRCLE('',#26742,0.19);
#9891=CIRCLE('',#26743,0.19);
#9892=CIRCLE('',#26744,0.19);
#9893=CIRCLE('',#26745,0.19);
#9894=CIRCLE('',#26746,0.19);
#9895=CIRCLE('',#26747,0.19);
#9896=CIRCLE('',#26748,0.19);
#9897=CIRCLE('',#26749,0.19);
#9898=CIRCLE('',#26750,0.19);
#9899=CIRCLE('',#26751,0.19);
#9900=CIRCLE('',#26752,0.19);
#9901=CIRCLE('',#26753,0.19);
#9902=CIRCLE('',#26754,0.19);
#9903=CIRCLE('',#26755,0.19);
#9904=CIRCLE('',#26756,0.19);
#9905=CIRCLE('',#26757,0.19);
#9906=CIRCLE('',#26758,0.19);
#9907=CIRCLE('',#26759,0.19);
#9908=CIRCLE('',#26760,0.19);
#9909=CIRCLE('',#26761,0.19);
#9910=CIRCLE('',#26762,0.19);
#9911=CIRCLE('',#26767,0.175);
#9912=CIRCLE('',#26769,0.0677181486487011);
#9913=CIRCLE('',#26778,0.076);
#9914=CIRCLE('',#26781,0.096675);
#9915=CIRCLE('',#26783,0.11);
#11545=VERTEX_POINT('',#44630);
#11546=VERTEX_POINT('',#44631);
#11547=VERTEX_POINT('',#44633);
#11548=VERTEX_POINT('',#44647);
#11549=VERTEX_POINT('',#44649);
#11550=VERTEX_POINT('',#44652);
#11551=VERTEX_POINT('',#44665);
#11552=VERTEX_POINT('',#44666);
#11553=VERTEX_POINT('',#44719);
#11554=VERTEX_POINT('',#44720);
#11555=VERTEX_POINT('',#44767);
#11556=VERTEX_POINT('',#44768);
#11557=VERTEX_POINT('',#44815);
#11558=VERTEX_POINT('',#44816);
#11559=VERTEX_POINT('',#44863);
#11560=VERTEX_POINT('',#44864);
#11561=VERTEX_POINT('',#44917);
#11562=VERTEX_POINT('',#44918);
#11563=VERTEX_POINT('',#44965);
#11564=VERTEX_POINT('',#44966);
#11565=VERTEX_POINT('',#45013);
#11566=VERTEX_POINT('',#45014);
#11567=VERTEX_POINT('',#45067);
#11568=VERTEX_POINT('',#45068);
#11569=VERTEX_POINT('',#45115);
#11570=VERTEX_POINT('',#45116);
#11571=VERTEX_POINT('',#45163);
#11572=VERTEX_POINT('',#45164);
#11573=VERTEX_POINT('',#45217);
#11574=VERTEX_POINT('',#45218);
#11575=VERTEX_POINT('',#45265);
#11576=VERTEX_POINT('',#45266);
#11577=VERTEX_POINT('',#45313);
#11578=VERTEX_POINT('',#45314);
#11579=VERTEX_POINT('',#45367);
#11580=VERTEX_POINT('',#45368);
#11581=VERTEX_POINT('',#45415);
#11582=VERTEX_POINT('',#45416);
#11583=VERTEX_POINT('',#45463);
#11584=VERTEX_POINT('',#45464);
#11585=VERTEX_POINT('',#45517);
#11586=VERTEX_POINT('',#45518);
#11587=VERTEX_POINT('',#45565);
#11588=VERTEX_POINT('',#45566);
#11589=VERTEX_POINT('',#45613);
#11590=VERTEX_POINT('',#45614);
#11591=VERTEX_POINT('',#45667);
#11592=VERTEX_POINT('',#45668);
#11593=VERTEX_POINT('',#45715);
#11594=VERTEX_POINT('',#45716);
#11595=VERTEX_POINT('',#45763);
#11596=VERTEX_POINT('',#45764);
#11597=VERTEX_POINT('',#45766);
#11598=VERTEX_POINT('',#45774);
#11599=VERTEX_POINT('',#45782);
#11600=VERTEX_POINT('',#45783);
#11601=VERTEX_POINT('',#45807);
#11602=VERTEX_POINT('',#45808);
#11603=VERTEX_POINT('',#45831);
#11604=VERTEX_POINT('',#45832);
#11605=VERTEX_POINT('',#45856);
#11606=VERTEX_POINT('',#45857);
#11607=VERTEX_POINT('',#45881);
#11608=VERTEX_POINT('',#45882);
#11609=VERTEX_POINT('',#45905);
#11610=VERTEX_POINT('',#45906);
#11611=VERTEX_POINT('',#45930);
#11612=VERTEX_POINT('',#45931);
#11613=VERTEX_POINT('',#45955);
#11614=VERTEX_POINT('',#45956);
#11615=VERTEX_POINT('',#45979);
#11616=VERTEX_POINT('',#45980);
#11617=VERTEX_POINT('',#46004);
#11618=VERTEX_POINT('',#46005);
#11619=VERTEX_POINT('',#46029);
#11620=VERTEX_POINT('',#46030);
#11621=VERTEX_POINT('',#46053);
#11622=VERTEX_POINT('',#46054);
#11623=VERTEX_POINT('',#46078);
#11624=VERTEX_POINT('',#46079);
#11625=VERTEX_POINT('',#46103);
#11626=VERTEX_POINT('',#46104);
#11627=VERTEX_POINT('',#46127);
#11628=VERTEX_POINT('',#46128);
#11629=VERTEX_POINT('',#46152);
#11630=VERTEX_POINT('',#46153);
#11631=VERTEX_POINT('',#46177);
#11632=VERTEX_POINT('',#46178);
#11633=VERTEX_POINT('',#46201);
#11634=VERTEX_POINT('',#46202);
#11635=VERTEX_POINT('',#46226);
#11636=VERTEX_POINT('',#46227);
#11637=VERTEX_POINT('',#46251);
#11638=VERTEX_POINT('',#46252);
#11639=VERTEX_POINT('',#46275);
#11640=VERTEX_POINT('',#46276);
#11641=VERTEX_POINT('',#46299);
#11642=VERTEX_POINT('',#46300);
#11643=VERTEX_POINT('',#46324);
#11644=VERTEX_POINT('',#46325);
#11645=VERTEX_POINT('',#46327);
#11646=VERTEX_POINT('',#46350);
#11647=VERTEX_POINT('',#46397);
#11648=VERTEX_POINT('',#46399);
#11649=VERTEX_POINT('',#47081);
#11650=VERTEX_POINT('',#47813);
#11651=VERTEX_POINT('',#47814);
#11652=VERTEX_POINT('',#47816);
#11653=VERTEX_POINT('',#47820);
#11654=VERTEX_POINT('',#47822);
#11655=VERTEX_POINT('',#47828);
#11656=VERTEX_POINT('',#47834);
#11657=VERTEX_POINT('',#47835);
#11658=VERTEX_POINT('',#47837);
#11659=VERTEX_POINT('',#47841);
#11660=VERTEX_POINT('',#47843);
#11661=VERTEX_POINT('',#47849);
#11662=VERTEX_POINT('',#47855);
#11663=VERTEX_POINT('',#47856);
#11664=VERTEX_POINT('',#47858);
#11665=VERTEX_POINT('',#47862);
#11666=VERTEX_POINT('',#47864);
#11667=VERTEX_POINT('',#47870);
#11668=VERTEX_POINT('',#47876);
#11669=VERTEX_POINT('',#47877);
#11670=VERTEX_POINT('',#47879);
#11671=VERTEX_POINT('',#47883);
#11672=VERTEX_POINT('',#47885);
#11673=VERTEX_POINT('',#47891);
#11674=VERTEX_POINT('',#47897);
#11675=VERTEX_POINT('',#47898);
#11676=VERTEX_POINT('',#47900);
#11677=VERTEX_POINT('',#47904);
#11678=VERTEX_POINT('',#47906);
#11679=VERTEX_POINT('',#47912);
#11680=VERTEX_POINT('',#47918);
#11681=VERTEX_POINT('',#47919);
#11682=VERTEX_POINT('',#47921);
#11683=VERTEX_POINT('',#47925);
#11684=VERTEX_POINT('',#47927);
#11685=VERTEX_POINT('',#47933);
#11686=VERTEX_POINT('',#47939);
#11687=VERTEX_POINT('',#47940);
#11688=VERTEX_POINT('',#47942);
#11689=VERTEX_POINT('',#47946);
#11690=VERTEX_POINT('',#47948);
#11691=VERTEX_POINT('',#47954);
#11692=VERTEX_POINT('',#47960);
#11693=VERTEX_POINT('',#47961);
#11694=VERTEX_POINT('',#47963);
#11695=VERTEX_POINT('',#47967);
#11696=VERTEX_POINT('',#47969);
#11697=VERTEX_POINT('',#47975);
#11698=VERTEX_POINT('',#47981);
#11699=VERTEX_POINT('',#47982);
#11700=VERTEX_POINT('',#47984);
#11701=VERTEX_POINT('',#47988);
#11702=VERTEX_POINT('',#47990);
#11703=VERTEX_POINT('',#47996);
#11704=VERTEX_POINT('',#48002);
#11705=VERTEX_POINT('',#48003);
#11706=VERTEX_POINT('',#48005);
#11707=VERTEX_POINT('',#48009);
#11708=VERTEX_POINT('',#48011);
#11709=VERTEX_POINT('',#48017);
#11710=VERTEX_POINT('',#48023);
#11711=VERTEX_POINT('',#48024);
#11712=VERTEX_POINT('',#48026);
#11713=VERTEX_POINT('',#48030);
#11714=VERTEX_POINT('',#48032);
#11715=VERTEX_POINT('',#48038);
#11716=VERTEX_POINT('',#48044);
#11717=VERTEX_POINT('',#48045);
#11718=VERTEX_POINT('',#48047);
#11719=VERTEX_POINT('',#48051);
#11720=VERTEX_POINT('',#48053);
#11721=VERTEX_POINT('',#48059);
#11722=VERTEX_POINT('',#48065);
#11723=VERTEX_POINT('',#48066);
#11724=VERTEX_POINT('',#48068);
#11725=VERTEX_POINT('',#48072);
#11726=VERTEX_POINT('',#48074);
#11727=VERTEX_POINT('',#48080);
#11728=VERTEX_POINT('',#48086);
#11729=VERTEX_POINT('',#48087);
#11730=VERTEX_POINT('',#48089);
#11731=VERTEX_POINT('',#48093);
#11732=VERTEX_POINT('',#48095);
#11733=VERTEX_POINT('',#48101);
#11734=VERTEX_POINT('',#48107);
#11735=VERTEX_POINT('',#48108);
#11736=VERTEX_POINT('',#48110);
#11737=VERTEX_POINT('',#48114);
#11738=VERTEX_POINT('',#48116);
#11739=VERTEX_POINT('',#48122);
#11740=VERTEX_POINT('',#48128);
#11741=VERTEX_POINT('',#48129);
#11742=VERTEX_POINT('',#48131);
#11743=VERTEX_POINT('',#48135);
#11744=VERTEX_POINT('',#48137);
#11745=VERTEX_POINT('',#48143);
#11746=VERTEX_POINT('',#48149);
#11747=VERTEX_POINT('',#48150);
#11748=VERTEX_POINT('',#48152);
#11749=VERTEX_POINT('',#48156);
#11750=VERTEX_POINT('',#48158);
#11751=VERTEX_POINT('',#48164);
#11752=VERTEX_POINT('',#48170);
#11753=VERTEX_POINT('',#48171);
#11754=VERTEX_POINT('',#48173);
#11755=VERTEX_POINT('',#48175);
#11756=VERTEX_POINT('',#48179);
#11757=VERTEX_POINT('',#48181);
#11758=VERTEX_POINT('',#48187);
#11759=VERTEX_POINT('',#48193);
#11760=VERTEX_POINT('',#48194);
#11761=VERTEX_POINT('',#48196);
#11762=VERTEX_POINT('',#48200);
#11763=VERTEX_POINT('',#48202);
#11764=VERTEX_POINT('',#48208);
#11765=VERTEX_POINT('',#48214);
#11766=VERTEX_POINT('',#48215);
#11767=VERTEX_POINT('',#48217);
#11768=VERTEX_POINT('',#48221);
#11769=VERTEX_POINT('',#48223);
#11770=VERTEX_POINT('',#48229);
#11771=VERTEX_POINT('',#48235);
#11772=VERTEX_POINT('',#48236);
#11773=VERTEX_POINT('',#48238);
#11774=VERTEX_POINT('',#48242);
#11775=VERTEX_POINT('',#48244);
#11776=VERTEX_POINT('',#48250);
#11777=VERTEX_POINT('',#48256);
#11778=VERTEX_POINT('',#48257);
#11779=VERTEX_POINT('',#48259);
#11780=VERTEX_POINT('',#48263);
#11781=VERTEX_POINT('',#48265);
#11782=VERTEX_POINT('',#48271);
#11783=VERTEX_POINT('',#48277);
#11784=VERTEX_POINT('',#48278);
#11785=VERTEX_POINT('',#48280);
#11786=VERTEX_POINT('',#48284);
#11787=VERTEX_POINT('',#48286);
#11788=VERTEX_POINT('',#48292);
#11789=VERTEX_POINT('',#48298);
#11790=VERTEX_POINT('',#48299);
#11791=VERTEX_POINT('',#48301);
#11792=VERTEX_POINT('',#48305);
#11793=VERTEX_POINT('',#48307);
#11794=VERTEX_POINT('',#48313);
#11795=VERTEX_POINT('',#48319);
#11796=VERTEX_POINT('',#48320);
#11797=VERTEX_POINT('',#48322);
#11798=VERTEX_POINT('',#48326);
#11799=VERTEX_POINT('',#48328);
#11800=VERTEX_POINT('',#48334);
#11801=VERTEX_POINT('',#48340);
#11802=VERTEX_POINT('',#48341);
#11803=VERTEX_POINT('',#48343);
#11804=VERTEX_POINT('',#48347);
#11805=VERTEX_POINT('',#48349);
#11806=VERTEX_POINT('',#48355);
#11807=VERTEX_POINT('',#48361);
#11808=VERTEX_POINT('',#48362);
#11809=VERTEX_POINT('',#48364);
#11810=VERTEX_POINT('',#48368);
#11811=VERTEX_POINT('',#48370);
#11812=VERTEX_POINT('',#48376);
#11813=VERTEX_POINT('',#48382);
#11814=VERTEX_POINT('',#48383);
#11815=VERTEX_POINT('',#48385);
#11816=VERTEX_POINT('',#48389);
#11817=VERTEX_POINT('',#48391);
#11818=VERTEX_POINT('',#48397);
#11819=VERTEX_POINT('',#48403);
#11820=VERTEX_POINT('',#48404);
#11821=VERTEX_POINT('',#48406);
#11822=VERTEX_POINT('',#48410);
#11823=VERTEX_POINT('',#48412);
#11824=VERTEX_POINT('',#48418);
#11825=VERTEX_POINT('',#48424);
#11826=VERTEX_POINT('',#48425);
#11827=VERTEX_POINT('',#48427);
#11828=VERTEX_POINT('',#48431);
#11829=VERTEX_POINT('',#48433);
#11830=VERTEX_POINT('',#48439);
#11831=VERTEX_POINT('',#48445);
#11832=VERTEX_POINT('',#48446);
#11833=VERTEX_POINT('',#48448);
#11834=VERTEX_POINT('',#48452);
#11835=VERTEX_POINT('',#48454);
#11836=VERTEX_POINT('',#48460);
#11837=VERTEX_POINT('',#48466);
#11838=VERTEX_POINT('',#48467);
#11839=VERTEX_POINT('',#48469);
#11840=VERTEX_POINT('',#48473);
#11841=VERTEX_POINT('',#48475);
#11842=VERTEX_POINT('',#48481);
#11843=VERTEX_POINT('',#48487);
#11844=VERTEX_POINT('',#48488);
#11845=VERTEX_POINT('',#48490);
#11846=VERTEX_POINT('',#48494);
#11847=VERTEX_POINT('',#48496);
#11848=VERTEX_POINT('',#48502);
#11849=VERTEX_POINT('',#48508);
#11850=VERTEX_POINT('',#48509);
#11851=VERTEX_POINT('',#48511);
#11852=VERTEX_POINT('',#48515);
#11853=VERTEX_POINT('',#48517);
#11854=VERTEX_POINT('',#48523);
#11855=VERTEX_POINT('',#48529);
#11856=VERTEX_POINT('',#48530);
#11857=VERTEX_POINT('',#48532);
#11858=VERTEX_POINT('',#48536);
#11859=VERTEX_POINT('',#48538);
#11860=VERTEX_POINT('',#48544);
#11861=VERTEX_POINT('',#48567);
#11862=VERTEX_POINT('',#48587);
#11863=VERTEX_POINT('',#48589);
#11864=VERTEX_POINT('',#48591);
#11865=VERTEX_POINT('',#48593);
#11866=VERTEX_POINT('',#48597);
#11867=VERTEX_POINT('',#48599);
#11868=VERTEX_POINT('',#48611);
#11869=VERTEX_POINT('',#48615);
#11870=VERTEX_POINT('',#48616);
#11871=VERTEX_POINT('',#48620);
#11872=VERTEX_POINT('',#48621);
#11873=VERTEX_POINT('',#48623);
#11874=VERTEX_POINT('',#48625);
#11875=VERTEX_POINT('',#48629);
#11876=VERTEX_POINT('',#48631);
#11877=VERTEX_POINT('',#48635);
#11878=VERTEX_POINT('',#48637);
#11879=VERTEX_POINT('',#48641);
#11880=VERTEX_POINT('',#48643);
#11881=VERTEX_POINT('',#48647);
#11882=VERTEX_POINT('',#48649);
#11883=VERTEX_POINT('',#48657);
#11884=VERTEX_POINT('',#48664);
#14673=EDGE_CURVE('',#11545,#11546,#6594,.T.);
#14674=EDGE_CURVE('',#11545,#11547,#689,.T.);
#14675=EDGE_CURVE('',#11547,#11548,#9829,.T.);
#14676=EDGE_CURVE('',#11548,#11549,#6595,.T.);
#14677=EDGE_CURVE('',#11549,#11549,#9830,.T.);
#14678=EDGE_CURVE('',#11548,#11550,#9831,.T.);
#14679=EDGE_CURVE('',#11550,#11546,#690,.T.);
#14680=EDGE_CURVE('',#11551,#11552,#6596,.T.);
#14681=EDGE_CURVE('',#11551,#11545,#691,.T.);
#14682=EDGE_CURVE('',#11546,#11552,#692,.T.);
#14683=EDGE_CURVE('',#11553,#11554,#6597,.T.);
#14684=EDGE_CURVE('',#11553,#11551,#693,.T.);
#14685=EDGE_CURVE('',#11552,#11554,#694,.T.);
#14686=EDGE_CURVE('',#11555,#11556,#6598,.T.);
#14687=EDGE_CURVE('',#11555,#11553,#695,.T.);
#14688=EDGE_CURVE('',#11554,#11556,#696,.T.);
#14689=EDGE_CURVE('',#11557,#11558,#6599,.T.);
#14690=EDGE_CURVE('',#11557,#11555,#697,.T.);
#14691=EDGE_CURVE('',#11556,#11558,#698,.T.);
#14692=EDGE_CURVE('',#11559,#11560,#6600,.T.);
#14693=EDGE_CURVE('',#11559,#11557,#699,.T.);
#14694=EDGE_CURVE('',#11558,#11560,#700,.T.);
#14695=EDGE_CURVE('',#11561,#11562,#6601,.T.);
#14696=EDGE_CURVE('',#11561,#11559,#701,.T.);
#14697=EDGE_CURVE('',#11560,#11562,#702,.T.);
#14698=EDGE_CURVE('',#11563,#11564,#6602,.T.);
#14699=EDGE_CURVE('',#11563,#11561,#703,.T.);
#14700=EDGE_CURVE('',#11562,#11564,#704,.T.);
#14701=EDGE_CURVE('',#11565,#11566,#6603,.T.);
#14702=EDGE_CURVE('',#11565,#11563,#705,.T.);
#14703=EDGE_CURVE('',#11564,#11566,#706,.T.);
#14704=EDGE_CURVE('',#11567,#11568,#6604,.T.);
#14705=EDGE_CURVE('',#11567,#11565,#707,.T.);
#14706=EDGE_CURVE('',#11566,#11568,#708,.T.);
#14707=EDGE_CURVE('',#11569,#11570,#6605,.T.);
#14708=EDGE_CURVE('',#11569,#11567,#709,.T.);
#14709=EDGE_CURVE('',#11568,#11570,#710,.T.);
#14710=EDGE_CURVE('',#11571,#11572,#6606,.T.);
#14711=EDGE_CURVE('',#11571,#11569,#711,.T.);
#14712=EDGE_CURVE('',#11570,#11572,#712,.T.);
#14713=EDGE_CURVE('',#11573,#11574,#6607,.T.);
#14714=EDGE_CURVE('',#11573,#11571,#713,.T.);
#14715=EDGE_CURVE('',#11572,#11574,#714,.T.);
#14716=EDGE_CURVE('',#11575,#11576,#6608,.T.);
#14717=EDGE_CURVE('',#11575,#11573,#715,.T.);
#14718=EDGE_CURVE('',#11574,#11576,#716,.T.);
#14719=EDGE_CURVE('',#11577,#11578,#6609,.T.);
#14720=EDGE_CURVE('',#11577,#11575,#717,.T.);
#14721=EDGE_CURVE('',#11576,#11578,#718,.T.);
#14722=EDGE_CURVE('',#11579,#11580,#6610,.T.);
#14723=EDGE_CURVE('',#11579,#11577,#719,.T.);
#14724=EDGE_CURVE('',#11578,#11580,#720,.T.);
#14725=EDGE_CURVE('',#11581,#11582,#6611,.T.);
#14726=EDGE_CURVE('',#11581,#11579,#721,.T.);
#14727=EDGE_CURVE('',#11580,#11582,#722,.T.);
#14728=EDGE_CURVE('',#11583,#11584,#6612,.T.);
#14729=EDGE_CURVE('',#11583,#11581,#723,.T.);
#14730=EDGE_CURVE('',#11582,#11584,#724,.T.);
#14731=EDGE_CURVE('',#11585,#11586,#6613,.T.);
#14732=EDGE_CURVE('',#11585,#11583,#725,.T.);
#14733=EDGE_CURVE('',#11584,#11586,#726,.T.);
#14734=EDGE_CURVE('',#11587,#11588,#6614,.T.);
#14735=EDGE_CURVE('',#11587,#11585,#727,.T.);
#14736=EDGE_CURVE('',#11586,#11588,#728,.T.);
#14737=EDGE_CURVE('',#11589,#11590,#6615,.T.);
#14738=EDGE_CURVE('',#11589,#11587,#729,.T.);
#14739=EDGE_CURVE('',#11588,#11590,#730,.T.);
#14740=EDGE_CURVE('',#11591,#11592,#6616,.T.);
#14741=EDGE_CURVE('',#11591,#11589,#731,.T.);
#14742=EDGE_CURVE('',#11590,#11592,#732,.T.);
#14743=EDGE_CURVE('',#11593,#11594,#6617,.T.);
#14744=EDGE_CURVE('',#11593,#11591,#733,.T.);
#14745=EDGE_CURVE('',#11592,#11594,#734,.T.);
#14746=EDGE_CURVE('',#11595,#11596,#6618,.T.);
#14747=EDGE_CURVE('',#11595,#11597,#735,.T.);
#14748=EDGE_CURVE('',#11598,#11597,#9832,.T.);
#14749=EDGE_CURVE('',#11596,#11598,#736,.T.);
#14750=EDGE_CURVE('',#11599,#11600,#6619,.T.);
#14751=EDGE_CURVE('',#11599,#11595,#737,.T.);
#14752=EDGE_CURVE('',#11600,#11596,#738,.T.);
#14753=EDGE_CURVE('',#11601,#11602,#6620,.T.);
#14754=EDGE_CURVE('',#11601,#11599,#739,.T.);
#14755=EDGE_CURVE('',#11602,#11600,#740,.T.);
#14756=EDGE_CURVE('',#11603,#11604,#6621,.T.);
#14757=EDGE_CURVE('',#11603,#11601,#741,.T.);
#14758=EDGE_CURVE('',#11604,#11602,#742,.T.);
#14759=EDGE_CURVE('',#11605,#11606,#6622,.T.);
#14760=EDGE_CURVE('',#11605,#11603,#743,.T.);
#14761=EDGE_CURVE('',#11606,#11604,#744,.T.);
#14762=EDGE_CURVE('',#11607,#11608,#6623,.T.);
#14763=EDGE_CURVE('',#11607,#11605,#745,.T.);
#14764=EDGE_CURVE('',#11608,#11606,#746,.T.);
#14765=EDGE_CURVE('',#11609,#11610,#6624,.T.);
#14766=EDGE_CURVE('',#11609,#11607,#747,.T.);
#14767=EDGE_CURVE('',#11610,#11608,#748,.T.);
#14768=EDGE_CURVE('',#11611,#11612,#6625,.T.);
#14769=EDGE_CURVE('',#11611,#11609,#749,.T.);
#14770=EDGE_CURVE('',#11612,#11610,#750,.T.);
#14771=EDGE_CURVE('',#11613,#11614,#6626,.T.);
#14772=EDGE_CURVE('',#11613,#11611,#751,.T.);
#14773=EDGE_CURVE('',#11614,#11612,#752,.T.);
#14774=EDGE_CURVE('',#11615,#11616,#6627,.T.);
#14775=EDGE_CURVE('',#11615,#11613,#753,.T.);
#14776=EDGE_CURVE('',#11616,#11614,#754,.T.);
#14777=EDGE_CURVE('',#11617,#11618,#6628,.T.);
#14778=EDGE_CURVE('',#11617,#11615,#755,.T.);
#14779=EDGE_CURVE('',#11618,#11616,#756,.T.);
#14780=EDGE_CURVE('',#11619,#11620,#6629,.T.);
#14781=EDGE_CURVE('',#11619,#11617,#757,.T.);
#14782=EDGE_CURVE('',#11620,#11618,#758,.T.);
#14783=EDGE_CURVE('',#11621,#11622,#6630,.T.);
#14784=EDGE_CURVE('',#11621,#11619,#759,.T.);
#14785=EDGE_CURVE('',#11622,#11620,#760,.T.);
#14786=EDGE_CURVE('',#11623,#11624,#6631,.T.);
#14787=EDGE_CURVE('',#11623,#11621,#761,.T.);
#14788=EDGE_CURVE('',#11624,#11622,#762,.T.);
#14789=EDGE_CURVE('',#11625,#11626,#6632,.T.);
#14790=EDGE_CURVE('',#11625,#11623,#763,.T.);
#14791=EDGE_CURVE('',#11626,#11624,#764,.T.);
#14792=EDGE_CURVE('',#11627,#11628,#6633,.T.);
#14793=EDGE_CURVE('',#11627,#11625,#765,.T.);
#14794=EDGE_CURVE('',#11628,#11626,#766,.T.);
#14795=EDGE_CURVE('',#11629,#11630,#6634,.T.);
#14796=EDGE_CURVE('',#11629,#11627,#767,.T.);
#14797=EDGE_CURVE('',#11630,#11628,#768,.T.);
#14798=EDGE_CURVE('',#11631,#11632,#6635,.T.);
#14799=EDGE_CURVE('',#11631,#11629,#769,.T.);
#14800=EDGE_CURVE('',#11632,#11630,#770,.T.);
#14801=EDGE_CURVE('',#11633,#11634,#6636,.T.);
#14802=EDGE_CURVE('',#11633,#11631,#771,.T.);
#14803=EDGE_CURVE('',#11634,#11632,#772,.T.);
#14804=EDGE_CURVE('',#11635,#11636,#6637,.T.);
#14805=EDGE_CURVE('',#11635,#11633,#773,.T.);
#14806=EDGE_CURVE('',#11636,#11634,#774,.T.);
#14807=EDGE_CURVE('',#11637,#11638,#6638,.T.);
#14808=EDGE_CURVE('',#11637,#11635,#775,.T.);
#14809=EDGE_CURVE('',#11638,#11636,#776,.T.);
#14810=EDGE_CURVE('',#11639,#11640,#6639,.T.);
#14811=EDGE_CURVE('',#11639,#11637,#777,.T.);
#14812=EDGE_CURVE('',#11640,#11638,#778,.T.);
#14813=EDGE_CURVE('',#11641,#11642,#6640,.T.);
#14814=EDGE_CURVE('',#11641,#11639,#779,.T.);
#14815=EDGE_CURVE('',#11642,#11640,#780,.T.);
#14816=EDGE_CURVE('',#11643,#11644,#6641,.T.);
#14817=EDGE_CURVE('',#11645,#11643,#9833,.T.);
#14818=EDGE_CURVE('',#11645,#11641,#781,.T.);
#14819=EDGE_CURVE('',#11644,#11642,#782,.T.);
#14820=EDGE_CURVE('',#11597,#11646,#783,.T.);
#14821=EDGE_CURVE('',#11647,#11646,#9834,.T.);
#14822=EDGE_CURVE('',#11648,#11647,#9835,.T.);
#14823=EDGE_CURVE('',#11648,#11598,#784,.T.);
#14824=EDGE_CURVE('',#11594,#11648,#785,.T.);
#14825=EDGE_CURVE('',#11649,#11550,#786,.T.);
#14826=EDGE_CURVE('',#11649,#11644,#787,.T.);
#14827=EDGE_CURVE('',#11547,#11645,#788,.T.);
#14828=EDGE_CURVE('',#11643,#11649,#9836,.T.);
#14829=EDGE_CURVE('',#11646,#11593,#789,.T.);
#14830=EDGE_CURVE('',#11650,#11651,#9837,.T.);
#14831=EDGE_CURVE('',#11650,#11652,#6642,.T.);
#14832=EDGE_CURVE('',#11652,#11651,#6643,.T.);
#14833=EDGE_CURVE('',#11651,#11653,#6644,.T.);
#14834=EDGE_CURVE('',#11652,#11654,#6645,.T.);
#14835=EDGE_CURVE('',#11653,#11654,#323,.T.);
#14836=EDGE_CURVE('',#11655,#11650,#6646,.T.);
#14837=EDGE_CURVE('',#11654,#11655,#324,.T.);
#14838=EDGE_CURVE('',#11656,#11657,#9838,.T.);
#14839=EDGE_CURVE('',#11656,#11658,#6647,.T.);
#14840=EDGE_CURVE('',#11658,#11657,#6648,.T.);
#14841=EDGE_CURVE('',#11657,#11659,#6649,.T.);
#14842=EDGE_CURVE('',#11658,#11660,#6650,.T.);
#14843=EDGE_CURVE('',#11659,#11660,#325,.T.);
#14844=EDGE_CURVE('',#11661,#11656,#6651,.T.);
#14845=EDGE_CURVE('',#11660,#11661,#326,.T.);
#14846=EDGE_CURVE('',#11662,#11663,#9839,.T.);
#14847=EDGE_CURVE('',#11662,#11664,#6652,.T.);
#14848=EDGE_CURVE('',#11664,#11663,#6653,.T.);
#14849=EDGE_CURVE('',#11663,#11665,#6654,.T.);
#14850=EDGE_CURVE('',#11664,#11666,#6655,.T.);
#14851=EDGE_CURVE('',#11665,#11666,#327,.T.);
#14852=EDGE_CURVE('',#11667,#11662,#6656,.T.);
#14853=EDGE_CURVE('',#11666,#11667,#328,.T.);
#14854=EDGE_CURVE('',#11668,#11669,#9840,.T.);
#14855=EDGE_CURVE('',#11668,#11670,#6657,.T.);
#14856=EDGE_CURVE('',#11670,#11669,#6658,.T.);
#14857=EDGE_CURVE('',#11669,#11671,#6659,.T.);
#14858=EDGE_CURVE('',#11670,#11672,#6660,.T.);
#14859=EDGE_CURVE('',#11671,#11672,#329,.T.);
#14860=EDGE_CURVE('',#11673,#11668,#6661,.T.);
#14861=EDGE_CURVE('',#11672,#11673,#330,.T.);
#14862=EDGE_CURVE('',#11674,#11675,#9841,.T.);
#14863=EDGE_CURVE('',#11674,#11676,#6662,.T.);
#14864=EDGE_CURVE('',#11676,#11675,#6663,.T.);
#14865=EDGE_CURVE('',#11675,#11677,#6664,.T.);
#14866=EDGE_CURVE('',#11676,#11678,#6665,.T.);
#14867=EDGE_CURVE('',#11677,#11678,#331,.T.);
#14868=EDGE_CURVE('',#11679,#11674,#6666,.T.);
#14869=EDGE_CURVE('',#11678,#11679,#332,.T.);
#14870=EDGE_CURVE('',#11680,#11681,#9842,.T.);
#14871=EDGE_CURVE('',#11680,#11682,#6667,.T.);
#14872=EDGE_CURVE('',#11682,#11681,#6668,.T.);
#14873=EDGE_CURVE('',#11681,#11683,#6669,.T.);
#14874=EDGE_CURVE('',#11682,#11684,#6670,.T.);
#14875=EDGE_CURVE('',#11683,#11684,#333,.T.);
#14876=EDGE_CURVE('',#11685,#11680,#6671,.T.);
#14877=EDGE_CURVE('',#11684,#11685,#334,.T.);
#14878=EDGE_CURVE('',#11686,#11687,#9843,.T.);
#14879=EDGE_CURVE('',#11686,#11688,#6672,.T.);
#14880=EDGE_CURVE('',#11688,#11687,#6673,.T.);
#14881=EDGE_CURVE('',#11687,#11689,#6674,.T.);
#14882=EDGE_CURVE('',#11688,#11690,#6675,.T.);
#14883=EDGE_CURVE('',#11689,#11690,#335,.T.);
#14884=EDGE_CURVE('',#11691,#11686,#6676,.T.);
#14885=EDGE_CURVE('',#11690,#11691,#336,.T.);
#14886=EDGE_CURVE('',#11692,#11693,#9844,.T.);
#14887=EDGE_CURVE('',#11692,#11694,#6677,.T.);
#14888=EDGE_CURVE('',#11694,#11693,#6678,.T.);
#14889=EDGE_CURVE('',#11693,#11695,#6679,.T.);
#14890=EDGE_CURVE('',#11694,#11696,#6680,.T.);
#14891=EDGE_CURVE('',#11695,#11696,#337,.T.);
#14892=EDGE_CURVE('',#11697,#11692,#6681,.T.);
#14893=EDGE_CURVE('',#11696,#11697,#338,.T.);
#14894=EDGE_CURVE('',#11698,#11699,#9845,.T.);
#14895=EDGE_CURVE('',#11698,#11700,#6682,.T.);
#14896=EDGE_CURVE('',#11700,#11699,#6683,.T.);
#14897=EDGE_CURVE('',#11699,#11701,#6684,.T.);
#14898=EDGE_CURVE('',#11700,#11702,#6685,.T.);
#14899=EDGE_CURVE('',#11701,#11702,#339,.T.);
#14900=EDGE_CURVE('',#11703,#11698,#6686,.T.);
#14901=EDGE_CURVE('',#11702,#11703,#340,.T.);
#14902=EDGE_CURVE('',#11704,#11705,#9846,.T.);
#14903=EDGE_CURVE('',#11704,#11706,#6687,.T.);
#14904=EDGE_CURVE('',#11706,#11705,#6688,.T.);
#14905=EDGE_CURVE('',#11705,#11707,#6689,.T.);
#14906=EDGE_CURVE('',#11706,#11708,#6690,.T.);
#14907=EDGE_CURVE('',#11707,#11708,#341,.T.);
#14908=EDGE_CURVE('',#11709,#11704,#6691,.T.);
#14909=EDGE_CURVE('',#11708,#11709,#342,.T.);
#14910=EDGE_CURVE('',#11710,#11711,#9847,.T.);
#14911=EDGE_CURVE('',#11710,#11712,#6692,.T.);
#14912=EDGE_CURVE('',#11712,#11711,#6693,.T.);
#14913=EDGE_CURVE('',#11711,#11713,#6694,.T.);
#14914=EDGE_CURVE('',#11712,#11714,#6695,.T.);
#14915=EDGE_CURVE('',#11713,#11714,#343,.T.);
#14916=EDGE_CURVE('',#11715,#11710,#6696,.T.);
#14917=EDGE_CURVE('',#11714,#11715,#344,.T.);
#14918=EDGE_CURVE('',#11716,#11717,#9848,.T.);
#14919=EDGE_CURVE('',#11716,#11718,#6697,.T.);
#14920=EDGE_CURVE('',#11718,#11717,#6698,.T.);
#14921=EDGE_CURVE('',#11717,#11719,#6699,.T.);
#14922=EDGE_CURVE('',#11718,#11720,#6700,.T.);
#14923=EDGE_CURVE('',#11719,#11720,#345,.T.);
#14924=EDGE_CURVE('',#11721,#11716,#6701,.T.);
#14925=EDGE_CURVE('',#11720,#11721,#346,.T.);
#14926=EDGE_CURVE('',#11722,#11723,#9849,.T.);
#14927=EDGE_CURVE('',#11722,#11724,#6702,.T.);
#14928=EDGE_CURVE('',#11724,#11723,#6703,.T.);
#14929=EDGE_CURVE('',#11723,#11725,#6704,.T.);
#14930=EDGE_CURVE('',#11724,#11726,#6705,.T.);
#14931=EDGE_CURVE('',#11725,#11726,#347,.T.);
#14932=EDGE_CURVE('',#11727,#11722,#6706,.T.);
#14933=EDGE_CURVE('',#11726,#11727,#348,.T.);
#14934=EDGE_CURVE('',#11728,#11729,#9850,.T.);
#14935=EDGE_CURVE('',#11728,#11730,#6707,.T.);
#14936=EDGE_CURVE('',#11730,#11729,#6708,.T.);
#14937=EDGE_CURVE('',#11729,#11731,#6709,.T.);
#14938=EDGE_CURVE('',#11730,#11732,#6710,.T.);
#14939=EDGE_CURVE('',#11731,#11732,#349,.T.);
#14940=EDGE_CURVE('',#11733,#11728,#6711,.T.);
#14941=EDGE_CURVE('',#11732,#11733,#350,.T.);
#14942=EDGE_CURVE('',#11734,#11735,#9851,.T.);
#14943=EDGE_CURVE('',#11734,#11736,#6712,.T.);
#14944=EDGE_CURVE('',#11736,#11735,#6713,.T.);
#14945=EDGE_CURVE('',#11735,#11737,#6714,.T.);
#14946=EDGE_CURVE('',#11736,#11738,#6715,.T.);
#14947=EDGE_CURVE('',#11737,#11738,#351,.T.);
#14948=EDGE_CURVE('',#11739,#11734,#6716,.T.);
#14949=EDGE_CURVE('',#11738,#11739,#352,.T.);
#14950=EDGE_CURVE('',#11740,#11741,#9852,.T.);
#14951=EDGE_CURVE('',#11740,#11742,#6717,.T.);
#14952=EDGE_CURVE('',#11742,#11741,#6718,.T.);
#14953=EDGE_CURVE('',#11741,#11743,#6719,.T.);
#14954=EDGE_CURVE('',#11742,#11744,#6720,.T.);
#14955=EDGE_CURVE('',#11743,#11744,#353,.T.);
#14956=EDGE_CURVE('',#11745,#11740,#6721,.T.);
#14957=EDGE_CURVE('',#11744,#11745,#354,.T.);
#14958=EDGE_CURVE('',#11746,#11747,#9853,.T.);
#14959=EDGE_CURVE('',#11746,#11748,#6722,.T.);
#14960=EDGE_CURVE('',#11748,#11747,#6723,.T.);
#14961=EDGE_CURVE('',#11747,#11749,#6724,.T.);
#14962=EDGE_CURVE('',#11748,#11750,#6725,.T.);
#14963=EDGE_CURVE('',#11749,#11750,#355,.T.);
#14964=EDGE_CURVE('',#11751,#11746,#6726,.T.);
#14965=EDGE_CURVE('',#11750,#11751,#356,.T.);
#14966=EDGE_CURVE('',#11752,#11753,#9854,.T.);
#14967=EDGE_CURVE('',#11752,#11754,#6727,.T.);
#14968=EDGE_CURVE('',#11754,#11755,#6728,.T.);
#14969=EDGE_CURVE('',#11753,#11755,#9855,.T.);
#14970=EDGE_CURVE('',#11755,#11756,#6729,.T.);
#14971=EDGE_CURVE('',#11754,#11757,#6730,.T.);
#14972=EDGE_CURVE('',#11756,#11757,#357,.T.);
#14973=EDGE_CURVE('',#11758,#11752,#6731,.T.);
#14974=EDGE_CURVE('',#11757,#11758,#358,.T.);
#14975=EDGE_CURVE('',#11759,#11760,#9856,.T.);
#14976=EDGE_CURVE('',#11759,#11761,#6732,.T.);
#14977=EDGE_CURVE('',#11761,#11760,#6733,.T.);
#14978=EDGE_CURVE('',#11760,#11762,#6734,.T.);
#14979=EDGE_CURVE('',#11761,#11763,#6735,.T.);
#14980=EDGE_CURVE('',#11762,#11763,#359,.T.);
#14981=EDGE_CURVE('',#11764,#11759,#6736,.T.);
#14982=EDGE_CURVE('',#11763,#11764,#360,.T.);
#14983=EDGE_CURVE('',#11765,#11766,#9857,.T.);
#14984=EDGE_CURVE('',#11765,#11767,#6737,.T.);
#14985=EDGE_CURVE('',#11767,#11766,#6738,.T.);
#14986=EDGE_CURVE('',#11766,#11768,#6739,.T.);
#14987=EDGE_CURVE('',#11767,#11769,#6740,.T.);
#14988=EDGE_CURVE('',#11768,#11769,#361,.T.);
#14989=EDGE_CURVE('',#11770,#11765,#6741,.T.);
#14990=EDGE_CURVE('',#11769,#11770,#362,.T.);
#14991=EDGE_CURVE('',#11771,#11772,#9858,.T.);
#14992=EDGE_CURVE('',#11771,#11773,#6742,.T.);
#14993=EDGE_CURVE('',#11773,#11772,#6743,.T.);
#14994=EDGE_CURVE('',#11772,#11774,#6744,.T.);
#14995=EDGE_CURVE('',#11773,#11775,#6745,.T.);
#14996=EDGE_CURVE('',#11774,#11775,#363,.T.);
#14997=EDGE_CURVE('',#11776,#11771,#6746,.T.);
#14998=EDGE_CURVE('',#11775,#11776,#364,.T.);
#14999=EDGE_CURVE('',#11777,#11778,#9859,.T.);
#15000=EDGE_CURVE('',#11777,#11779,#6747,.T.);
#15001=EDGE_CURVE('',#11779,#11778,#6748,.T.);
#15002=EDGE_CURVE('',#11778,#11780,#6749,.T.);
#15003=EDGE_CURVE('',#11779,#11781,#6750,.T.);
#15004=EDGE_CURVE('',#11780,#11781,#365,.T.);
#15005=EDGE_CURVE('',#11782,#11777,#6751,.T.);
#15006=EDGE_CURVE('',#11781,#11782,#366,.T.);
#15007=EDGE_CURVE('',#11783,#11784,#9860,.T.);
#15008=EDGE_CURVE('',#11783,#11785,#6752,.T.);
#15009=EDGE_CURVE('',#11785,#11784,#6753,.T.);
#15010=EDGE_CURVE('',#11784,#11786,#6754,.T.);
#15011=EDGE_CURVE('',#11785,#11787,#6755,.T.);
#15012=EDGE_CURVE('',#11786,#11787,#367,.T.);
#15013=EDGE_CURVE('',#11788,#11783,#6756,.T.);
#15014=EDGE_CURVE('',#11787,#11788,#368,.T.);
#15015=EDGE_CURVE('',#11789,#11790,#9861,.T.);
#15016=EDGE_CURVE('',#11789,#11791,#6757,.T.);
#15017=EDGE_CURVE('',#11791,#11790,#6758,.T.);
#15018=EDGE_CURVE('',#11790,#11792,#6759,.T.);
#15019=EDGE_CURVE('',#11791,#11793,#6760,.T.);
#15020=EDGE_CURVE('',#11792,#11793,#369,.T.);
#15021=EDGE_CURVE('',#11794,#11789,#6761,.T.);
#15022=EDGE_CURVE('',#11793,#11794,#370,.T.);
#15023=EDGE_CURVE('',#11795,#11796,#9862,.T.);
#15024=EDGE_CURVE('',#11795,#11797,#6762,.T.);
#15025=EDGE_CURVE('',#11797,#11796,#6763,.T.);
#15026=EDGE_CURVE('',#11796,#11798,#6764,.T.);
#15027=EDGE_CURVE('',#11797,#11799,#6765,.T.);
#15028=EDGE_CURVE('',#11798,#11799,#371,.T.);
#15029=EDGE_CURVE('',#11800,#11795,#6766,.T.);
#15030=EDGE_CURVE('',#11799,#11800,#372,.T.);
#15031=EDGE_CURVE('',#11801,#11802,#9863,.T.);
#15032=EDGE_CURVE('',#11801,#11803,#6767,.T.);
#15033=EDGE_CURVE('',#11803,#11802,#6768,.T.);
#15034=EDGE_CURVE('',#11802,#11804,#6769,.T.);
#15035=EDGE_CURVE('',#11803,#11805,#6770,.T.);
#15036=EDGE_CURVE('',#11804,#11805,#373,.T.);
#15037=EDGE_CURVE('',#11806,#11801,#6771,.T.);
#15038=EDGE_CURVE('',#11805,#11806,#374,.T.);
#15039=EDGE_CURVE('',#11807,#11808,#9864,.T.);
#15040=EDGE_CURVE('',#11807,#11809,#6772,.T.);
#15041=EDGE_CURVE('',#11809,#11808,#6773,.T.);
#15042=EDGE_CURVE('',#11808,#11810,#6774,.T.);
#15043=EDGE_CURVE('',#11809,#11811,#6775,.T.);
#15044=EDGE_CURVE('',#11810,#11811,#375,.T.);
#15045=EDGE_CURVE('',#11812,#11807,#6776,.T.);
#15046=EDGE_CURVE('',#11811,#11812,#376,.T.);
#15047=EDGE_CURVE('',#11813,#11814,#9865,.T.);
#15048=EDGE_CURVE('',#11813,#11815,#6777,.T.);
#15049=EDGE_CURVE('',#11815,#11814,#6778,.T.);
#15050=EDGE_CURVE('',#11814,#11816,#6779,.T.);
#15051=EDGE_CURVE('',#11815,#11817,#6780,.T.);
#15052=EDGE_CURVE('',#11816,#11817,#377,.T.);
#15053=EDGE_CURVE('',#11818,#11813,#6781,.T.);
#15054=EDGE_CURVE('',#11817,#11818,#378,.T.);
#15055=EDGE_CURVE('',#11819,#11820,#9866,.T.);
#15056=EDGE_CURVE('',#11819,#11821,#6782,.T.);
#15057=EDGE_CURVE('',#11821,#11820,#6783,.T.);
#15058=EDGE_CURVE('',#11820,#11822,#6784,.T.);
#15059=EDGE_CURVE('',#11821,#11823,#6785,.T.);
#15060=EDGE_CURVE('',#11822,#11823,#379,.T.);
#15061=EDGE_CURVE('',#11824,#11819,#6786,.T.);
#15062=EDGE_CURVE('',#11823,#11824,#380,.T.);
#15063=EDGE_CURVE('',#11825,#11826,#9867,.T.);
#15064=EDGE_CURVE('',#11825,#11827,#6787,.T.);
#15065=EDGE_CURVE('',#11827,#11826,#6788,.T.);
#15066=EDGE_CURVE('',#11826,#11828,#6789,.T.);
#15067=EDGE_CURVE('',#11827,#11829,#6790,.T.);
#15068=EDGE_CURVE('',#11828,#11829,#381,.T.);
#15069=EDGE_CURVE('',#11830,#11825,#6791,.T.);
#15070=EDGE_CURVE('',#11829,#11830,#382,.T.);
#15071=EDGE_CURVE('',#11831,#11832,#9868,.T.);
#15072=EDGE_CURVE('',#11831,#11833,#6792,.T.);
#15073=EDGE_CURVE('',#11833,#11832,#6793,.T.);
#15074=EDGE_CURVE('',#11832,#11834,#6794,.T.);
#15075=EDGE_CURVE('',#11833,#11835,#6795,.T.);
#15076=EDGE_CURVE('',#11834,#11835,#383,.T.);
#15077=EDGE_CURVE('',#11836,#11831,#6796,.T.);
#15078=EDGE_CURVE('',#11835,#11836,#384,.T.);
#15079=EDGE_CURVE('',#11837,#11838,#9869,.T.);
#15080=EDGE_CURVE('',#11837,#11839,#6797,.T.);
#15081=EDGE_CURVE('',#11839,#11838,#6798,.T.);
#15082=EDGE_CURVE('',#11838,#11840,#6799,.T.);
#15083=EDGE_CURVE('',#11839,#11841,#6800,.T.);
#15084=EDGE_CURVE('',#11840,#11841,#385,.T.);
#15085=EDGE_CURVE('',#11842,#11837,#6801,.T.);
#15086=EDGE_CURVE('',#11841,#11842,#386,.T.);
#15087=EDGE_CURVE('',#11843,#11844,#9870,.T.);
#15088=EDGE_CURVE('',#11843,#11845,#6802,.T.);
#15089=EDGE_CURVE('',#11845,#11844,#6803,.T.);
#15090=EDGE_CURVE('',#11844,#11846,#6804,.T.);
#15091=EDGE_CURVE('',#11845,#11847,#6805,.T.);
#15092=EDGE_CURVE('',#11846,#11847,#387,.T.);
#15093=EDGE_CURVE('',#11848,#11843,#6806,.T.);
#15094=EDGE_CURVE('',#11847,#11848,#388,.T.);
#15095=EDGE_CURVE('',#11849,#11850,#9871,.T.);
#15096=EDGE_CURVE('',#11849,#11851,#6807,.T.);
#15097=EDGE_CURVE('',#11851,#11850,#6808,.T.);
#15098=EDGE_CURVE('',#11850,#11852,#6809,.T.);
#15099=EDGE_CURVE('',#11851,#11853,#6810,.T.);
#15100=EDGE_CURVE('',#11852,#11853,#389,.T.);
#15101=EDGE_CURVE('',#11854,#11849,#6811,.T.);
#15102=EDGE_CURVE('',#11853,#11854,#390,.T.);
#15103=EDGE_CURVE('',#11855,#11856,#9872,.T.);
#15104=EDGE_CURVE('',#11855,#11857,#6812,.T.);
#15105=EDGE_CURVE('',#11857,#11856,#6813,.T.);
#15106=EDGE_CURVE('',#11856,#11858,#6814,.T.);
#15107=EDGE_CURVE('',#11857,#11859,#6815,.T.);
#15108=EDGE_CURVE('',#11858,#11859,#391,.T.);
#15109=EDGE_CURVE('',#11860,#11855,#6816,.T.);
#15110=EDGE_CURVE('',#11859,#11860,#392,.T.);
#15111=EDGE_CURVE('',#11661,#11653,#9873,.T.);
#15112=EDGE_CURVE('',#11667,#11659,#9874,.T.);
#15113=EDGE_CURVE('',#11673,#11665,#9875,.T.);
#15114=EDGE_CURVE('',#11679,#11671,#9876,.T.);
#15115=EDGE_CURVE('',#11685,#11677,#9877,.T.);
#15116=EDGE_CURVE('',#11691,#11683,#9878,.T.);
#15117=EDGE_CURVE('',#11697,#11689,#9879,.T.);
#15118=EDGE_CURVE('',#11703,#11695,#9880,.T.);
#15119=EDGE_CURVE('',#11709,#11701,#9881,.T.);
#15120=EDGE_CURVE('',#11715,#11707,#9882,.T.);
#15121=EDGE_CURVE('',#11721,#11713,#9883,.T.);
#15122=EDGE_CURVE('',#11727,#11719,#9884,.T.);
#15123=EDGE_CURVE('',#11733,#11725,#9885,.T.);
#15124=EDGE_CURVE('',#11739,#11731,#9886,.T.);
#15125=EDGE_CURVE('',#11745,#11737,#9887,.T.);
#15126=EDGE_CURVE('',#11751,#11743,#9888,.T.);
#15127=EDGE_CURVE('',#11758,#11749,#9889,.T.);
#15128=EDGE_CURVE('',#11753,#11861,#6817,.T.);
#15129=EDGE_CURVE('',#11861,#11861,#9890,.T.);
#15130=EDGE_CURVE('',#11764,#11756,#9891,.T.);
#15131=EDGE_CURVE('',#11770,#11762,#9892,.T.);
#15132=EDGE_CURVE('',#11776,#11768,#9893,.T.);
#15133=EDGE_CURVE('',#11782,#11774,#9894,.T.);
#15134=EDGE_CURVE('',#11788,#11780,#9895,.T.);
#15135=EDGE_CURVE('',#11794,#11786,#9896,.T.);
#15136=EDGE_CURVE('',#11800,#11792,#9897,.T.);
#15137=EDGE_CURVE('',#11806,#11798,#9898,.T.);
#15138=EDGE_CURVE('',#11812,#11804,#9899,.T.);
#15139=EDGE_CURVE('',#11818,#11810,#9900,.T.);
#15140=EDGE_CURVE('',#11824,#11816,#9901,.T.);
#15141=EDGE_CURVE('',#11830,#11822,#9902,.T.);
#15142=EDGE_CURVE('',#11836,#11828,#9903,.T.);
#15143=EDGE_CURVE('',#11842,#11834,#9904,.T.);
#15144=EDGE_CURVE('',#11848,#11840,#9905,.T.);
#15145=EDGE_CURVE('',#11854,#11846,#9906,.T.);
#15146=EDGE_CURVE('',#11860,#11852,#9907,.T.);
#15147=EDGE_CURVE('',#11862,#11858,#9908,.T.);
#15148=EDGE_CURVE('',#11862,#11863,#6818,.T.);
#15149=EDGE_CURVE('',#11863,#11864,#9909,.T.);
#15150=EDGE_CURVE('',#11864,#11865,#6819,.T.);
#15151=EDGE_CURVE('',#11655,#11865,#9910,.T.);
#15152=EDGE_CURVE('',#11866,#11864,#6820,.T.);
#15153=EDGE_CURVE('',#11866,#11867,#6821,.T.);
#15154=EDGE_CURVE('',#11865,#11867,#393,.T.);
#15155=EDGE_CURVE('',#11867,#11862,#394,.T.);
#15156=EDGE_CURVE('',#11863,#11866,#6822,.T.);
#15157=EDGE_CURVE('',#11868,#11868,#9911,.T.);
#15158=EDGE_CURVE('',#11868,#11757,#6823,.T.);
#15159=EDGE_CURVE('',#11869,#11870,#6824,.T.);
#15160=EDGE_CURVE('',#11870,#11870,#9912,.T.);
#15161=EDGE_CURVE('',#11871,#11872,#6825,.T.);
#15162=EDGE_CURVE('',#11871,#11873,#6826,.T.);
#15163=EDGE_CURVE('',#11873,#11874,#6827,.T.);
#15164=EDGE_CURVE('',#11872,#11874,#6828,.T.);
#15165=EDGE_CURVE('',#11875,#11871,#6829,.T.);
#15166=EDGE_CURVE('',#11875,#11876,#6830,.T.);
#15167=EDGE_CURVE('',#11876,#11873,#6831,.T.);
#15168=EDGE_CURVE('',#11877,#11875,#6832,.T.);
#15169=EDGE_CURVE('',#11877,#11878,#6833,.T.);
#15170=EDGE_CURVE('',#11878,#11876,#6834,.T.);
#15171=EDGE_CURVE('',#11879,#11877,#6835,.T.);
#15172=EDGE_CURVE('',#11879,#11880,#6836,.T.);
#15173=EDGE_CURVE('',#11880,#11878,#6837,.T.);
#15174=EDGE_CURVE('',#11881,#11879,#6838,.T.);
#15175=EDGE_CURVE('',#11881,#11882,#6839,.T.);
#15176=EDGE_CURVE('',#11882,#11880,#6840,.T.);
#15177=EDGE_CURVE('',#11872,#11881,#6841,.T.);
#15178=EDGE_CURVE('',#11874,#11882,#6842,.T.);
#15179=EDGE_CURVE('',#11883,#11883,#9913,.T.);
#15180=EDGE_CURVE('',#11549,#11883,#6843,.T.);
#15181=EDGE_CURVE('',#11646,#11648,#9914,.T.);
#15182=EDGE_CURVE('',#11884,#11884,#9915,.T.);
#15183=EDGE_CURVE('',#11884,#11647,#6844,.T.);
#20530=ORIENTED_EDGE('',*,*,#14673,.F.);
#20531=ORIENTED_EDGE('',*,*,#14674,.T.);
#20532=ORIENTED_EDGE('',*,*,#14675,.T.);
#20533=ORIENTED_EDGE('',*,*,#14676,.T.);
#20534=ORIENTED_EDGE('',*,*,#14677,.T.);
#20535=ORIENTED_EDGE('',*,*,#14676,.F.);
#20536=ORIENTED_EDGE('',*,*,#14678,.T.);
#20537=ORIENTED_EDGE('',*,*,#14679,.T.);
#20538=ORIENTED_EDGE('',*,*,#14680,.F.);
#20539=ORIENTED_EDGE('',*,*,#14681,.T.);
#20540=ORIENTED_EDGE('',*,*,#14673,.T.);
#20541=ORIENTED_EDGE('',*,*,#14682,.T.);
#20542=ORIENTED_EDGE('',*,*,#14683,.F.);
#20543=ORIENTED_EDGE('',*,*,#14684,.T.);
#20544=ORIENTED_EDGE('',*,*,#14680,.T.);
#20545=ORIENTED_EDGE('',*,*,#14685,.T.);
#20546=ORIENTED_EDGE('',*,*,#14686,.F.);
#20547=ORIENTED_EDGE('',*,*,#14687,.T.);
#20548=ORIENTED_EDGE('',*,*,#14683,.T.);
#20549=ORIENTED_EDGE('',*,*,#14688,.T.);
#20550=ORIENTED_EDGE('',*,*,#14689,.F.);
#20551=ORIENTED_EDGE('',*,*,#14690,.T.);
#20552=ORIENTED_EDGE('',*,*,#14686,.T.);
#20553=ORIENTED_EDGE('',*,*,#14691,.T.);
#20554=ORIENTED_EDGE('',*,*,#14692,.F.);
#20555=ORIENTED_EDGE('',*,*,#14693,.T.);
#20556=ORIENTED_EDGE('',*,*,#14689,.T.);
#20557=ORIENTED_EDGE('',*,*,#14694,.T.);
#20558=ORIENTED_EDGE('',*,*,#14695,.F.);
#20559=ORIENTED_EDGE('',*,*,#14696,.T.);
#20560=ORIENTED_EDGE('',*,*,#14692,.T.);
#20561=ORIENTED_EDGE('',*,*,#14697,.T.);
#20562=ORIENTED_EDGE('',*,*,#14698,.F.);
#20563=ORIENTED_EDGE('',*,*,#14699,.T.);
#20564=ORIENTED_EDGE('',*,*,#14695,.T.);
#20565=ORIENTED_EDGE('',*,*,#14700,.T.);
#20566=ORIENTED_EDGE('',*,*,#14701,.F.);
#20567=ORIENTED_EDGE('',*,*,#14702,.T.);
#20568=ORIENTED_EDGE('',*,*,#14698,.T.);
#20569=ORIENTED_EDGE('',*,*,#14703,.T.);
#20570=ORIENTED_EDGE('',*,*,#14704,.F.);
#20571=ORIENTED_EDGE('',*,*,#14705,.T.);
#20572=ORIENTED_EDGE('',*,*,#14701,.T.);
#20573=ORIENTED_EDGE('',*,*,#14706,.T.);
#20574=ORIENTED_EDGE('',*,*,#14707,.F.);
#20575=ORIENTED_EDGE('',*,*,#14708,.T.);
#20576=ORIENTED_EDGE('',*,*,#14704,.T.);
#20577=ORIENTED_EDGE('',*,*,#14709,.T.);
#20578=ORIENTED_EDGE('',*,*,#14710,.F.);
#20579=ORIENTED_EDGE('',*,*,#14711,.T.);
#20580=ORIENTED_EDGE('',*,*,#14707,.T.);
#20581=ORIENTED_EDGE('',*,*,#14712,.T.);
#20582=ORIENTED_EDGE('',*,*,#14713,.F.);
#20583=ORIENTED_EDGE('',*,*,#14714,.T.);
#20584=ORIENTED_EDGE('',*,*,#14710,.T.);
#20585=ORIENTED_EDGE('',*,*,#14715,.T.);
#20586=ORIENTED_EDGE('',*,*,#14716,.F.);
#20587=ORIENTED_EDGE('',*,*,#14717,.T.);
#20588=ORIENTED_EDGE('',*,*,#14713,.T.);
#20589=ORIENTED_EDGE('',*,*,#14718,.T.);
#20590=ORIENTED_EDGE('',*,*,#14719,.F.);
#20591=ORIENTED_EDGE('',*,*,#14720,.T.);
#20592=ORIENTED_EDGE('',*,*,#14716,.T.);
#20593=ORIENTED_EDGE('',*,*,#14721,.T.);
#20594=ORIENTED_EDGE('',*,*,#14722,.F.);
#20595=ORIENTED_EDGE('',*,*,#14723,.T.);
#20596=ORIENTED_EDGE('',*,*,#14719,.T.);
#20597=ORIENTED_EDGE('',*,*,#14724,.T.);
#20598=ORIENTED_EDGE('',*,*,#14725,.F.);
#20599=ORIENTED_EDGE('',*,*,#14726,.T.);
#20600=ORIENTED_EDGE('',*,*,#14722,.T.);
#20601=ORIENTED_EDGE('',*,*,#14727,.T.);
#20602=ORIENTED_EDGE('',*,*,#14728,.F.);
#20603=ORIENTED_EDGE('',*,*,#14729,.T.);
#20604=ORIENTED_EDGE('',*,*,#14725,.T.);
#20605=ORIENTED_EDGE('',*,*,#14730,.T.);
#20606=ORIENTED_EDGE('',*,*,#14731,.F.);
#20607=ORIENTED_EDGE('',*,*,#14732,.T.);
#20608=ORIENTED_EDGE('',*,*,#14728,.T.);
#20609=ORIENTED_EDGE('',*,*,#14733,.T.);
#20610=ORIENTED_EDGE('',*,*,#14734,.F.);
#20611=ORIENTED_EDGE('',*,*,#14735,.T.);
#20612=ORIENTED_EDGE('',*,*,#14731,.T.);
#20613=ORIENTED_EDGE('',*,*,#14736,.T.);
#20614=ORIENTED_EDGE('',*,*,#14737,.F.);
#20615=ORIENTED_EDGE('',*,*,#14738,.T.);
#20616=ORIENTED_EDGE('',*,*,#14734,.T.);
#20617=ORIENTED_EDGE('',*,*,#14739,.T.);
#20618=ORIENTED_EDGE('',*,*,#14740,.F.);
#20619=ORIENTED_EDGE('',*,*,#14741,.T.);
#20620=ORIENTED_EDGE('',*,*,#14737,.T.);
#20621=ORIENTED_EDGE('',*,*,#14742,.T.);
#20622=ORIENTED_EDGE('',*,*,#14743,.F.);
#20623=ORIENTED_EDGE('',*,*,#14744,.T.);
#20624=ORIENTED_EDGE('',*,*,#14740,.T.);
#20625=ORIENTED_EDGE('',*,*,#14745,.T.);
#20626=ORIENTED_EDGE('',*,*,#14746,.F.);
#20627=ORIENTED_EDGE('',*,*,#14747,.T.);
#20628=ORIENTED_EDGE('',*,*,#14748,.F.);
#20629=ORIENTED_EDGE('',*,*,#14749,.F.);
#20630=ORIENTED_EDGE('',*,*,#14750,.F.);
#20631=ORIENTED_EDGE('',*,*,#14751,.T.);
#20632=ORIENTED_EDGE('',*,*,#14746,.T.);
#20633=ORIENTED_EDGE('',*,*,#14752,.F.);
#20634=ORIENTED_EDGE('',*,*,#14753,.F.);
#20635=ORIENTED_EDGE('',*,*,#14754,.T.);
#20636=ORIENTED_EDGE('',*,*,#14750,.T.);
#20637=ORIENTED_EDGE('',*,*,#14755,.F.);
#20638=ORIENTED_EDGE('',*,*,#14756,.F.);
#20639=ORIENTED_EDGE('',*,*,#14757,.T.);
#20640=ORIENTED_EDGE('',*,*,#14753,.T.);
#20641=ORIENTED_EDGE('',*,*,#14758,.F.);
#20642=ORIENTED_EDGE('',*,*,#14759,.F.);
#20643=ORIENTED_EDGE('',*,*,#14760,.T.);
#20644=ORIENTED_EDGE('',*,*,#14756,.T.);
#20645=ORIENTED_EDGE('',*,*,#14761,.F.);
#20646=ORIENTED_EDGE('',*,*,#14762,.F.);
#20647=ORIENTED_EDGE('',*,*,#14763,.T.);
#20648=ORIENTED_EDGE('',*,*,#14759,.T.);
#20649=ORIENTED_EDGE('',*,*,#14764,.F.);
#20650=ORIENTED_EDGE('',*,*,#14765,.F.);
#20651=ORIENTED_EDGE('',*,*,#14766,.T.);
#20652=ORIENTED_EDGE('',*,*,#14762,.T.);
#20653=ORIENTED_EDGE('',*,*,#14767,.F.);
#20654=ORIENTED_EDGE('',*,*,#14768,.F.);
#20655=ORIENTED_EDGE('',*,*,#14769,.T.);
#20656=ORIENTED_EDGE('',*,*,#14765,.T.);
#20657=ORIENTED_EDGE('',*,*,#14770,.F.);
#20658=ORIENTED_EDGE('',*,*,#14771,.F.);
#20659=ORIENTED_EDGE('',*,*,#14772,.T.);
#20660=ORIENTED_EDGE('',*,*,#14768,.T.);
#20661=ORIENTED_EDGE('',*,*,#14773,.F.);
#20662=ORIENTED_EDGE('',*,*,#14774,.F.);
#20663=ORIENTED_EDGE('',*,*,#14775,.T.);
#20664=ORIENTED_EDGE('',*,*,#14771,.T.);
#20665=ORIENTED_EDGE('',*,*,#14776,.F.);
#20666=ORIENTED_EDGE('',*,*,#14777,.F.);
#20667=ORIENTED_EDGE('',*,*,#14778,.T.);
#20668=ORIENTED_EDGE('',*,*,#14774,.T.);
#20669=ORIENTED_EDGE('',*,*,#14779,.F.);
#20670=ORIENTED_EDGE('',*,*,#14780,.F.);
#20671=ORIENTED_EDGE('',*,*,#14781,.T.);
#20672=ORIENTED_EDGE('',*,*,#14777,.T.);
#20673=ORIENTED_EDGE('',*,*,#14782,.F.);
#20674=ORIENTED_EDGE('',*,*,#14783,.F.);
#20675=ORIENTED_EDGE('',*,*,#14784,.T.);
#20676=ORIENTED_EDGE('',*,*,#14780,.T.);
#20677=ORIENTED_EDGE('',*,*,#14785,.F.);
#20678=ORIENTED_EDGE('',*,*,#14786,.F.);
#20679=ORIENTED_EDGE('',*,*,#14787,.T.);
#20680=ORIENTED_EDGE('',*,*,#14783,.T.);
#20681=ORIENTED_EDGE('',*,*,#14788,.F.);
#20682=ORIENTED_EDGE('',*,*,#14789,.F.);
#20683=ORIENTED_EDGE('',*,*,#14790,.T.);
#20684=ORIENTED_EDGE('',*,*,#14786,.T.);
#20685=ORIENTED_EDGE('',*,*,#14791,.F.);
#20686=ORIENTED_EDGE('',*,*,#14792,.F.);
#20687=ORIENTED_EDGE('',*,*,#14793,.T.);
#20688=ORIENTED_EDGE('',*,*,#14789,.T.);
#20689=ORIENTED_EDGE('',*,*,#14794,.F.);
#20690=ORIENTED_EDGE('',*,*,#14795,.F.);
#20691=ORIENTED_EDGE('',*,*,#14796,.T.);
#20692=ORIENTED_EDGE('',*,*,#14792,.T.);
#20693=ORIENTED_EDGE('',*,*,#14797,.F.);
#20694=ORIENTED_EDGE('',*,*,#14798,.F.);
#20695=ORIENTED_EDGE('',*,*,#14799,.T.);
#20696=ORIENTED_EDGE('',*,*,#14795,.T.);
#20697=ORIENTED_EDGE('',*,*,#14800,.F.);
#20698=ORIENTED_EDGE('',*,*,#14801,.F.);
#20699=ORIENTED_EDGE('',*,*,#14802,.T.);
#20700=ORIENTED_EDGE('',*,*,#14798,.T.);
#20701=ORIENTED_EDGE('',*,*,#14803,.F.);
#20702=ORIENTED_EDGE('',*,*,#14804,.F.);
#20703=ORIENTED_EDGE('',*,*,#14805,.T.);
#20704=ORIENTED_EDGE('',*,*,#14801,.T.);
#20705=ORIENTED_EDGE('',*,*,#14806,.F.);
#20706=ORIENTED_EDGE('',*,*,#14807,.F.);
#20707=ORIENTED_EDGE('',*,*,#14808,.T.);
#20708=ORIENTED_EDGE('',*,*,#14804,.T.);
#20709=ORIENTED_EDGE('',*,*,#14809,.F.);
#20710=ORIENTED_EDGE('',*,*,#14810,.F.);
#20711=ORIENTED_EDGE('',*,*,#14811,.T.);
#20712=ORIENTED_EDGE('',*,*,#14807,.T.);
#20713=ORIENTED_EDGE('',*,*,#14812,.F.);
#20714=ORIENTED_EDGE('',*,*,#14813,.F.);
#20715=ORIENTED_EDGE('',*,*,#14814,.T.);
#20716=ORIENTED_EDGE('',*,*,#14810,.T.);
#20717=ORIENTED_EDGE('',*,*,#14815,.F.);
#20718=ORIENTED_EDGE('',*,*,#14816,.F.);
#20719=ORIENTED_EDGE('',*,*,#14817,.F.);
#20720=ORIENTED_EDGE('',*,*,#14818,.T.);
#20721=ORIENTED_EDGE('',*,*,#14813,.T.);
#20722=ORIENTED_EDGE('',*,*,#14819,.F.);
#20723=ORIENTED_EDGE('',*,*,#14748,.T.);
#20724=ORIENTED_EDGE('',*,*,#14820,.T.);
#20725=ORIENTED_EDGE('',*,*,#14821,.F.);
#20726=ORIENTED_EDGE('',*,*,#14822,.F.);
#20727=ORIENTED_EDGE('',*,*,#14823,.T.);
#20728=ORIENTED_EDGE('',*,*,#14823,.F.);
#20729=ORIENTED_EDGE('',*,*,#14824,.F.);
#20730=ORIENTED_EDGE('',*,*,#14745,.F.);
#20731=ORIENTED_EDGE('',*,*,#14742,.F.);
#20732=ORIENTED_EDGE('',*,*,#14739,.F.);
#20733=ORIENTED_EDGE('',*,*,#14736,.F.);
#20734=ORIENTED_EDGE('',*,*,#14733,.F.);
#20735=ORIENTED_EDGE('',*,*,#14730,.F.);
#20736=ORIENTED_EDGE('',*,*,#14727,.F.);
#20737=ORIENTED_EDGE('',*,*,#14724,.F.);
#20738=ORIENTED_EDGE('',*,*,#14721,.F.);
#20739=ORIENTED_EDGE('',*,*,#14718,.F.);
#20740=ORIENTED_EDGE('',*,*,#14715,.F.);
#20741=ORIENTED_EDGE('',*,*,#14712,.F.);
#20742=ORIENTED_EDGE('',*,*,#14709,.F.);
#20743=ORIENTED_EDGE('',*,*,#14706,.F.);
#20744=ORIENTED_EDGE('',*,*,#14703,.F.);
#20745=ORIENTED_EDGE('',*,*,#14700,.F.);
#20746=ORIENTED_EDGE('',*,*,#14697,.F.);
#20747=ORIENTED_EDGE('',*,*,#14694,.F.);
#20748=ORIENTED_EDGE('',*,*,#14691,.F.);
#20749=ORIENTED_EDGE('',*,*,#14688,.F.);
#20750=ORIENTED_EDGE('',*,*,#14685,.F.);
#20751=ORIENTED_EDGE('',*,*,#14682,.F.);
#20752=ORIENTED_EDGE('',*,*,#14679,.F.);
#20753=ORIENTED_EDGE('',*,*,#14825,.F.);
#20754=ORIENTED_EDGE('',*,*,#14826,.T.);
#20755=ORIENTED_EDGE('',*,*,#14819,.T.);
#20756=ORIENTED_EDGE('',*,*,#14815,.T.);
#20757=ORIENTED_EDGE('',*,*,#14812,.T.);
#20758=ORIENTED_EDGE('',*,*,#14809,.T.);
#20759=ORIENTED_EDGE('',*,*,#14806,.T.);
#20760=ORIENTED_EDGE('',*,*,#14803,.T.);
#20761=ORIENTED_EDGE('',*,*,#14800,.T.);
#20762=ORIENTED_EDGE('',*,*,#14797,.T.);
#20763=ORIENTED_EDGE('',*,*,#14794,.T.);
#20764=ORIENTED_EDGE('',*,*,#14791,.T.);
#20765=ORIENTED_EDGE('',*,*,#14788,.T.);
#20766=ORIENTED_EDGE('',*,*,#14785,.T.);
#20767=ORIENTED_EDGE('',*,*,#14782,.T.);
#20768=ORIENTED_EDGE('',*,*,#14779,.T.);
#20769=ORIENTED_EDGE('',*,*,#14776,.T.);
#20770=ORIENTED_EDGE('',*,*,#14773,.T.);
#20771=ORIENTED_EDGE('',*,*,#14770,.T.);
#20772=ORIENTED_EDGE('',*,*,#14767,.T.);
#20773=ORIENTED_EDGE('',*,*,#14764,.T.);
#20774=ORIENTED_EDGE('',*,*,#14761,.T.);
#20775=ORIENTED_EDGE('',*,*,#14758,.T.);
#20776=ORIENTED_EDGE('',*,*,#14755,.T.);
#20777=ORIENTED_EDGE('',*,*,#14752,.T.);
#20778=ORIENTED_EDGE('',*,*,#14749,.T.);
#20779=ORIENTED_EDGE('',*,*,#14675,.F.);
#20780=ORIENTED_EDGE('',*,*,#14827,.T.);
#20781=ORIENTED_EDGE('',*,*,#14817,.T.);
#20782=ORIENTED_EDGE('',*,*,#14828,.T.);
#20783=ORIENTED_EDGE('',*,*,#14825,.T.);
#20784=ORIENTED_EDGE('',*,*,#14678,.F.);
#20785=ORIENTED_EDGE('',*,*,#14816,.T.);
#20786=ORIENTED_EDGE('',*,*,#14826,.F.);
#20787=ORIENTED_EDGE('',*,*,#14828,.F.);
#20788=ORIENTED_EDGE('',*,*,#14820,.F.);
#20789=ORIENTED_EDGE('',*,*,#14747,.F.);
#20790=ORIENTED_EDGE('',*,*,#14751,.F.);
#20791=ORIENTED_EDGE('',*,*,#14754,.F.);
#20792=ORIENTED_EDGE('',*,*,#14757,.F.);
#20793=ORIENTED_EDGE('',*,*,#14760,.F.);
#20794=ORIENTED_EDGE('',*,*,#14763,.F.);
#20795=ORIENTED_EDGE('',*,*,#14766,.F.);
#20796=ORIENTED_EDGE('',*,*,#14769,.F.);
#20797=ORIENTED_EDGE('',*,*,#14772,.F.);
#20798=ORIENTED_EDGE('',*,*,#14775,.F.);
#20799=ORIENTED_EDGE('',*,*,#14778,.F.);
#20800=ORIENTED_EDGE('',*,*,#14781,.F.);
#20801=ORIENTED_EDGE('',*,*,#14784,.F.);
#20802=ORIENTED_EDGE('',*,*,#14787,.F.);
#20803=ORIENTED_EDGE('',*,*,#14790,.F.);
#20804=ORIENTED_EDGE('',*,*,#14793,.F.);
#20805=ORIENTED_EDGE('',*,*,#14796,.F.);
#20806=ORIENTED_EDGE('',*,*,#14799,.F.);
#20807=ORIENTED_EDGE('',*,*,#14802,.F.);
#20808=ORIENTED_EDGE('',*,*,#14805,.F.);
#20809=ORIENTED_EDGE('',*,*,#14808,.F.);
#20810=ORIENTED_EDGE('',*,*,#14811,.F.);
#20811=ORIENTED_EDGE('',*,*,#14814,.F.);
#20812=ORIENTED_EDGE('',*,*,#14818,.F.);
#20813=ORIENTED_EDGE('',*,*,#14827,.F.);
#20814=ORIENTED_EDGE('',*,*,#14674,.F.);
#20815=ORIENTED_EDGE('',*,*,#14681,.F.);
#20816=ORIENTED_EDGE('',*,*,#14684,.F.);
#20817=ORIENTED_EDGE('',*,*,#14687,.F.);
#20818=ORIENTED_EDGE('',*,*,#14690,.F.);
#20819=ORIENTED_EDGE('',*,*,#14693,.F.);
#20820=ORIENTED_EDGE('',*,*,#14696,.F.);
#20821=ORIENTED_EDGE('',*,*,#14699,.F.);
#20822=ORIENTED_EDGE('',*,*,#14702,.F.);
#20823=ORIENTED_EDGE('',*,*,#14705,.F.);
#20824=ORIENTED_EDGE('',*,*,#14708,.F.);
#20825=ORIENTED_EDGE('',*,*,#14711,.F.);
#20826=ORIENTED_EDGE('',*,*,#14714,.F.);
#20827=ORIENTED_EDGE('',*,*,#14717,.F.);
#20828=ORIENTED_EDGE('',*,*,#14720,.F.);
#20829=ORIENTED_EDGE('',*,*,#14723,.F.);
#20830=ORIENTED_EDGE('',*,*,#14726,.F.);
#20831=ORIENTED_EDGE('',*,*,#14729,.F.);
#20832=ORIENTED_EDGE('',*,*,#14732,.F.);
#20833=ORIENTED_EDGE('',*,*,#14735,.F.);
#20834=ORIENTED_EDGE('',*,*,#14738,.F.);
#20835=ORIENTED_EDGE('',*,*,#14741,.F.);
#20836=ORIENTED_EDGE('',*,*,#14744,.F.);
#20837=ORIENTED_EDGE('',*,*,#14829,.F.);
#20838=ORIENTED_EDGE('',*,*,#14830,.F.);
#20839=ORIENTED_EDGE('',*,*,#14831,.T.);
#20840=ORIENTED_EDGE('',*,*,#14832,.T.);
#20841=ORIENTED_EDGE('',*,*,#14833,.F.);
#20842=ORIENTED_EDGE('',*,*,#14832,.F.);
#20843=ORIENTED_EDGE('',*,*,#14834,.T.);
#20844=ORIENTED_EDGE('',*,*,#14835,.F.);
#20845=ORIENTED_EDGE('',*,*,#14836,.F.);
#20846=ORIENTED_EDGE('',*,*,#14837,.F.);
#20847=ORIENTED_EDGE('',*,*,#14834,.F.);
#20848=ORIENTED_EDGE('',*,*,#14831,.F.);
#20849=ORIENTED_EDGE('',*,*,#14838,.F.);
#20850=ORIENTED_EDGE('',*,*,#14839,.T.);
#20851=ORIENTED_EDGE('',*,*,#14840,.T.);
#20852=ORIENTED_EDGE('',*,*,#14841,.F.);
#20853=ORIENTED_EDGE('',*,*,#14840,.F.);
#20854=ORIENTED_EDGE('',*,*,#14842,.T.);
#20855=ORIENTED_EDGE('',*,*,#14843,.F.);
#20856=ORIENTED_EDGE('',*,*,#14844,.F.);
#20857=ORIENTED_EDGE('',*,*,#14845,.F.);
#20858=ORIENTED_EDGE('',*,*,#14842,.F.);
#20859=ORIENTED_EDGE('',*,*,#14839,.F.);
#20860=ORIENTED_EDGE('',*,*,#14846,.F.);
#20861=ORIENTED_EDGE('',*,*,#14847,.T.);
#20862=ORIENTED_EDGE('',*,*,#14848,.T.);
#20863=ORIENTED_EDGE('',*,*,#14849,.F.);
#20864=ORIENTED_EDGE('',*,*,#14848,.F.);
#20865=ORIENTED_EDGE('',*,*,#14850,.T.);
#20866=ORIENTED_EDGE('',*,*,#14851,.F.);
#20867=ORIENTED_EDGE('',*,*,#14852,.F.);
#20868=ORIENTED_EDGE('',*,*,#14853,.F.);
#20869=ORIENTED_EDGE('',*,*,#14850,.F.);
#20870=ORIENTED_EDGE('',*,*,#14847,.F.);
#20871=ORIENTED_EDGE('',*,*,#14854,.F.);
#20872=ORIENTED_EDGE('',*,*,#14855,.T.);
#20873=ORIENTED_EDGE('',*,*,#14856,.T.);
#20874=ORIENTED_EDGE('',*,*,#14857,.F.);
#20875=ORIENTED_EDGE('',*,*,#14856,.F.);
#20876=ORIENTED_EDGE('',*,*,#14858,.T.);
#20877=ORIENTED_EDGE('',*,*,#14859,.F.);
#20878=ORIENTED_EDGE('',*,*,#14860,.F.);
#20879=ORIENTED_EDGE('',*,*,#14861,.F.);
#20880=ORIENTED_EDGE('',*,*,#14858,.F.);
#20881=ORIENTED_EDGE('',*,*,#14855,.F.);
#20882=ORIENTED_EDGE('',*,*,#14862,.F.);
#20883=ORIENTED_EDGE('',*,*,#14863,.T.);
#20884=ORIENTED_EDGE('',*,*,#14864,.T.);
#20885=ORIENTED_EDGE('',*,*,#14865,.F.);
#20886=ORIENTED_EDGE('',*,*,#14864,.F.);
#20887=ORIENTED_EDGE('',*,*,#14866,.T.);
#20888=ORIENTED_EDGE('',*,*,#14867,.F.);
#20889=ORIENTED_EDGE('',*,*,#14868,.F.);
#20890=ORIENTED_EDGE('',*,*,#14869,.F.);
#20891=ORIENTED_EDGE('',*,*,#14866,.F.);
#20892=ORIENTED_EDGE('',*,*,#14863,.F.);
#20893=ORIENTED_EDGE('',*,*,#14870,.F.);
#20894=ORIENTED_EDGE('',*,*,#14871,.T.);
#20895=ORIENTED_EDGE('',*,*,#14872,.T.);
#20896=ORIENTED_EDGE('',*,*,#14873,.F.);
#20897=ORIENTED_EDGE('',*,*,#14872,.F.);
#20898=ORIENTED_EDGE('',*,*,#14874,.T.);
#20899=ORIENTED_EDGE('',*,*,#14875,.F.);
#20900=ORIENTED_EDGE('',*,*,#14876,.F.);
#20901=ORIENTED_EDGE('',*,*,#14877,.F.);
#20902=ORIENTED_EDGE('',*,*,#14874,.F.);
#20903=ORIENTED_EDGE('',*,*,#14871,.F.);
#20904=ORIENTED_EDGE('',*,*,#14878,.F.);
#20905=ORIENTED_EDGE('',*,*,#14879,.T.);
#20906=ORIENTED_EDGE('',*,*,#14880,.T.);
#20907=ORIENTED_EDGE('',*,*,#14881,.F.);
#20908=ORIENTED_EDGE('',*,*,#14880,.F.);
#20909=ORIENTED_EDGE('',*,*,#14882,.T.);
#20910=ORIENTED_EDGE('',*,*,#14883,.F.);
#20911=ORIENTED_EDGE('',*,*,#14884,.F.);
#20912=ORIENTED_EDGE('',*,*,#14885,.F.);
#20913=ORIENTED_EDGE('',*,*,#14882,.F.);
#20914=ORIENTED_EDGE('',*,*,#14879,.F.);
#20915=ORIENTED_EDGE('',*,*,#14886,.F.);
#20916=ORIENTED_EDGE('',*,*,#14887,.T.);
#20917=ORIENTED_EDGE('',*,*,#14888,.T.);
#20918=ORIENTED_EDGE('',*,*,#14889,.F.);
#20919=ORIENTED_EDGE('',*,*,#14888,.F.);
#20920=ORIENTED_EDGE('',*,*,#14890,.T.);
#20921=ORIENTED_EDGE('',*,*,#14891,.F.);
#20922=ORIENTED_EDGE('',*,*,#14892,.F.);
#20923=ORIENTED_EDGE('',*,*,#14893,.F.);
#20924=ORIENTED_EDGE('',*,*,#14890,.F.);
#20925=ORIENTED_EDGE('',*,*,#14887,.F.);
#20926=ORIENTED_EDGE('',*,*,#14894,.F.);
#20927=ORIENTED_EDGE('',*,*,#14895,.T.);
#20928=ORIENTED_EDGE('',*,*,#14896,.T.);
#20929=ORIENTED_EDGE('',*,*,#14897,.F.);
#20930=ORIENTED_EDGE('',*,*,#14896,.F.);
#20931=ORIENTED_EDGE('',*,*,#14898,.T.);
#20932=ORIENTED_EDGE('',*,*,#14899,.F.);
#20933=ORIENTED_EDGE('',*,*,#14900,.F.);
#20934=ORIENTED_EDGE('',*,*,#14901,.F.);
#20935=ORIENTED_EDGE('',*,*,#14898,.F.);
#20936=ORIENTED_EDGE('',*,*,#14895,.F.);
#20937=ORIENTED_EDGE('',*,*,#14902,.F.);
#20938=ORIENTED_EDGE('',*,*,#14903,.T.);
#20939=ORIENTED_EDGE('',*,*,#14904,.T.);
#20940=ORIENTED_EDGE('',*,*,#14905,.F.);
#20941=ORIENTED_EDGE('',*,*,#14904,.F.);
#20942=ORIENTED_EDGE('',*,*,#14906,.T.);
#20943=ORIENTED_EDGE('',*,*,#14907,.F.);
#20944=ORIENTED_EDGE('',*,*,#14908,.F.);
#20945=ORIENTED_EDGE('',*,*,#14909,.F.);
#20946=ORIENTED_EDGE('',*,*,#14906,.F.);
#20947=ORIENTED_EDGE('',*,*,#14903,.F.);
#20948=ORIENTED_EDGE('',*,*,#14910,.F.);
#20949=ORIENTED_EDGE('',*,*,#14911,.T.);
#20950=ORIENTED_EDGE('',*,*,#14912,.T.);
#20951=ORIENTED_EDGE('',*,*,#14913,.F.);
#20952=ORIENTED_EDGE('',*,*,#14912,.F.);
#20953=ORIENTED_EDGE('',*,*,#14914,.T.);
#20954=ORIENTED_EDGE('',*,*,#14915,.F.);
#20955=ORIENTED_EDGE('',*,*,#14916,.F.);
#20956=ORIENTED_EDGE('',*,*,#14917,.F.);
#20957=ORIENTED_EDGE('',*,*,#14914,.F.);
#20958=ORIENTED_EDGE('',*,*,#14911,.F.);
#20959=ORIENTED_EDGE('',*,*,#14918,.F.);
#20960=ORIENTED_EDGE('',*,*,#14919,.T.);
#20961=ORIENTED_EDGE('',*,*,#14920,.T.);
#20962=ORIENTED_EDGE('',*,*,#14921,.F.);
#20963=ORIENTED_EDGE('',*,*,#14920,.F.);
#20964=ORIENTED_EDGE('',*,*,#14922,.T.);
#20965=ORIENTED_EDGE('',*,*,#14923,.F.);
#20966=ORIENTED_EDGE('',*,*,#14924,.F.);
#20967=ORIENTED_EDGE('',*,*,#14925,.F.);
#20968=ORIENTED_EDGE('',*,*,#14922,.F.);
#20969=ORIENTED_EDGE('',*,*,#14919,.F.);
#20970=ORIENTED_EDGE('',*,*,#14926,.F.);
#20971=ORIENTED_EDGE('',*,*,#14927,.T.);
#20972=ORIENTED_EDGE('',*,*,#14928,.T.);
#20973=ORIENTED_EDGE('',*,*,#14929,.F.);
#20974=ORIENTED_EDGE('',*,*,#14928,.F.);
#20975=ORIENTED_EDGE('',*,*,#14930,.T.);
#20976=ORIENTED_EDGE('',*,*,#14931,.F.);
#20977=ORIENTED_EDGE('',*,*,#14932,.F.);
#20978=ORIENTED_EDGE('',*,*,#14933,.F.);
#20979=ORIENTED_EDGE('',*,*,#14930,.F.);
#20980=ORIENTED_EDGE('',*,*,#14927,.F.);
#20981=ORIENTED_EDGE('',*,*,#14934,.F.);
#20982=ORIENTED_EDGE('',*,*,#14935,.T.);
#20983=ORIENTED_EDGE('',*,*,#14936,.T.);
#20984=ORIENTED_EDGE('',*,*,#14937,.F.);
#20985=ORIENTED_EDGE('',*,*,#14936,.F.);
#20986=ORIENTED_EDGE('',*,*,#14938,.T.);
#20987=ORIENTED_EDGE('',*,*,#14939,.F.);
#20988=ORIENTED_EDGE('',*,*,#14940,.F.);
#20989=ORIENTED_EDGE('',*,*,#14941,.F.);
#20990=ORIENTED_EDGE('',*,*,#14938,.F.);
#20991=ORIENTED_EDGE('',*,*,#14935,.F.);
#20992=ORIENTED_EDGE('',*,*,#14942,.F.);
#20993=ORIENTED_EDGE('',*,*,#14943,.T.);
#20994=ORIENTED_EDGE('',*,*,#14944,.T.);
#20995=ORIENTED_EDGE('',*,*,#14945,.F.);
#20996=ORIENTED_EDGE('',*,*,#14944,.F.);
#20997=ORIENTED_EDGE('',*,*,#14946,.T.);
#20998=ORIENTED_EDGE('',*,*,#14947,.F.);
#20999=ORIENTED_EDGE('',*,*,#14948,.F.);
#21000=ORIENTED_EDGE('',*,*,#14949,.F.);
#21001=ORIENTED_EDGE('',*,*,#14946,.F.);
#21002=ORIENTED_EDGE('',*,*,#14943,.F.);
#21003=ORIENTED_EDGE('',*,*,#14950,.F.);
#21004=ORIENTED_EDGE('',*,*,#14951,.T.);
#21005=ORIENTED_EDGE('',*,*,#14952,.T.);
#21006=ORIENTED_EDGE('',*,*,#14953,.F.);
#21007=ORIENTED_EDGE('',*,*,#14952,.F.);
#21008=ORIENTED_EDGE('',*,*,#14954,.T.);
#21009=ORIENTED_EDGE('',*,*,#14955,.F.);
#21010=ORIENTED_EDGE('',*,*,#14956,.F.);
#21011=ORIENTED_EDGE('',*,*,#14957,.F.);
#21012=ORIENTED_EDGE('',*,*,#14954,.F.);
#21013=ORIENTED_EDGE('',*,*,#14951,.F.);
#21014=ORIENTED_EDGE('',*,*,#14958,.F.);
#21015=ORIENTED_EDGE('',*,*,#14959,.T.);
#21016=ORIENTED_EDGE('',*,*,#14960,.T.);
#21017=ORIENTED_EDGE('',*,*,#14961,.F.);
#21018=ORIENTED_EDGE('',*,*,#14960,.F.);
#21019=ORIENTED_EDGE('',*,*,#14962,.T.);
#21020=ORIENTED_EDGE('',*,*,#14963,.F.);
#21021=ORIENTED_EDGE('',*,*,#14964,.F.);
#21022=ORIENTED_EDGE('',*,*,#14965,.F.);
#21023=ORIENTED_EDGE('',*,*,#14962,.F.);
#21024=ORIENTED_EDGE('',*,*,#14959,.F.);
#21025=ORIENTED_EDGE('',*,*,#14966,.F.);
#21026=ORIENTED_EDGE('',*,*,#14967,.T.);
#21027=ORIENTED_EDGE('',*,*,#14968,.T.);
#21028=ORIENTED_EDGE('',*,*,#14969,.F.);
#21029=ORIENTED_EDGE('',*,*,#14970,.F.);
#21030=ORIENTED_EDGE('',*,*,#14968,.F.);
#21031=ORIENTED_EDGE('',*,*,#14971,.T.);
#21032=ORIENTED_EDGE('',*,*,#14972,.F.);
#21033=ORIENTED_EDGE('',*,*,#14973,.F.);
#21034=ORIENTED_EDGE('',*,*,#14974,.F.);
#21035=ORIENTED_EDGE('',*,*,#14971,.F.);
#21036=ORIENTED_EDGE('',*,*,#14967,.F.);
#21037=ORIENTED_EDGE('',*,*,#14975,.F.);
#21038=ORIENTED_EDGE('',*,*,#14976,.T.);
#21039=ORIENTED_EDGE('',*,*,#14977,.T.);
#21040=ORIENTED_EDGE('',*,*,#14978,.F.);
#21041=ORIENTED_EDGE('',*,*,#14977,.F.);
#21042=ORIENTED_EDGE('',*,*,#14979,.T.);
#21043=ORIENTED_EDGE('',*,*,#14980,.F.);
#21044=ORIENTED_EDGE('',*,*,#14981,.F.);
#21045=ORIENTED_EDGE('',*,*,#14982,.F.);
#21046=ORIENTED_EDGE('',*,*,#14979,.F.);
#21047=ORIENTED_EDGE('',*,*,#14976,.F.);
#21048=ORIENTED_EDGE('',*,*,#14983,.F.);
#21049=ORIENTED_EDGE('',*,*,#14984,.T.);
#21050=ORIENTED_EDGE('',*,*,#14985,.T.);
#21051=ORIENTED_EDGE('',*,*,#14986,.F.);
#21052=ORIENTED_EDGE('',*,*,#14985,.F.);
#21053=ORIENTED_EDGE('',*,*,#14987,.T.);
#21054=ORIENTED_EDGE('',*,*,#14988,.F.);
#21055=ORIENTED_EDGE('',*,*,#14989,.F.);
#21056=ORIENTED_EDGE('',*,*,#14990,.F.);
#21057=ORIENTED_EDGE('',*,*,#14987,.F.);
#21058=ORIENTED_EDGE('',*,*,#14984,.F.);
#21059=ORIENTED_EDGE('',*,*,#14991,.F.);
#21060=ORIENTED_EDGE('',*,*,#14992,.T.);
#21061=ORIENTED_EDGE('',*,*,#14993,.T.);
#21062=ORIENTED_EDGE('',*,*,#14994,.F.);
#21063=ORIENTED_EDGE('',*,*,#14993,.F.);
#21064=ORIENTED_EDGE('',*,*,#14995,.T.);
#21065=ORIENTED_EDGE('',*,*,#14996,.F.);
#21066=ORIENTED_EDGE('',*,*,#14997,.F.);
#21067=ORIENTED_EDGE('',*,*,#14998,.F.);
#21068=ORIENTED_EDGE('',*,*,#14995,.F.);
#21069=ORIENTED_EDGE('',*,*,#14992,.F.);
#21070=ORIENTED_EDGE('',*,*,#14999,.F.);
#21071=ORIENTED_EDGE('',*,*,#15000,.T.);
#21072=ORIENTED_EDGE('',*,*,#15001,.T.);
#21073=ORIENTED_EDGE('',*,*,#15002,.F.);
#21074=ORIENTED_EDGE('',*,*,#15001,.F.);
#21075=ORIENTED_EDGE('',*,*,#15003,.T.);
#21076=ORIENTED_EDGE('',*,*,#15004,.F.);
#21077=ORIENTED_EDGE('',*,*,#15005,.F.);
#21078=ORIENTED_EDGE('',*,*,#15006,.F.);
#21079=ORIENTED_EDGE('',*,*,#15003,.F.);
#21080=ORIENTED_EDGE('',*,*,#15000,.F.);
#21081=ORIENTED_EDGE('',*,*,#15007,.F.);
#21082=ORIENTED_EDGE('',*,*,#15008,.T.);
#21083=ORIENTED_EDGE('',*,*,#15009,.T.);
#21084=ORIENTED_EDGE('',*,*,#15010,.F.);
#21085=ORIENTED_EDGE('',*,*,#15009,.F.);
#21086=ORIENTED_EDGE('',*,*,#15011,.T.);
#21087=ORIENTED_EDGE('',*,*,#15012,.F.);
#21088=ORIENTED_EDGE('',*,*,#15013,.F.);
#21089=ORIENTED_EDGE('',*,*,#15014,.F.);
#21090=ORIENTED_EDGE('',*,*,#15011,.F.);
#21091=ORIENTED_EDGE('',*,*,#15008,.F.);
#21092=ORIENTED_EDGE('',*,*,#15015,.F.);
#21093=ORIENTED_EDGE('',*,*,#15016,.T.);
#21094=ORIENTED_EDGE('',*,*,#15017,.T.);
#21095=ORIENTED_EDGE('',*,*,#15018,.F.);
#21096=ORIENTED_EDGE('',*,*,#15017,.F.);
#21097=ORIENTED_EDGE('',*,*,#15019,.T.);
#21098=ORIENTED_EDGE('',*,*,#15020,.F.);
#21099=ORIENTED_EDGE('',*,*,#15021,.F.);
#21100=ORIENTED_EDGE('',*,*,#15022,.F.);
#21101=ORIENTED_EDGE('',*,*,#15019,.F.);
#21102=ORIENTED_EDGE('',*,*,#15016,.F.);
#21103=ORIENTED_EDGE('',*,*,#15023,.F.);
#21104=ORIENTED_EDGE('',*,*,#15024,.T.);
#21105=ORIENTED_EDGE('',*,*,#15025,.T.);
#21106=ORIENTED_EDGE('',*,*,#15026,.F.);
#21107=ORIENTED_EDGE('',*,*,#15025,.F.);
#21108=ORIENTED_EDGE('',*,*,#15027,.T.);
#21109=ORIENTED_EDGE('',*,*,#15028,.F.);
#21110=ORIENTED_EDGE('',*,*,#15029,.F.);
#21111=ORIENTED_EDGE('',*,*,#15030,.F.);
#21112=ORIENTED_EDGE('',*,*,#15027,.F.);
#21113=ORIENTED_EDGE('',*,*,#15024,.F.);
#21114=ORIENTED_EDGE('',*,*,#15031,.F.);
#21115=ORIENTED_EDGE('',*,*,#15032,.T.);
#21116=ORIENTED_EDGE('',*,*,#15033,.T.);
#21117=ORIENTED_EDGE('',*,*,#15034,.F.);
#21118=ORIENTED_EDGE('',*,*,#15033,.F.);
#21119=ORIENTED_EDGE('',*,*,#15035,.T.);
#21120=ORIENTED_EDGE('',*,*,#15036,.F.);
#21121=ORIENTED_EDGE('',*,*,#15037,.F.);
#21122=ORIENTED_EDGE('',*,*,#15038,.F.);
#21123=ORIENTED_EDGE('',*,*,#15035,.F.);
#21124=ORIENTED_EDGE('',*,*,#15032,.F.);
#21125=ORIENTED_EDGE('',*,*,#15039,.F.);
#21126=ORIENTED_EDGE('',*,*,#15040,.T.);
#21127=ORIENTED_EDGE('',*,*,#15041,.T.);
#21128=ORIENTED_EDGE('',*,*,#15042,.F.);
#21129=ORIENTED_EDGE('',*,*,#15041,.F.);
#21130=ORIENTED_EDGE('',*,*,#15043,.T.);
#21131=ORIENTED_EDGE('',*,*,#15044,.F.);
#21132=ORIENTED_EDGE('',*,*,#15045,.F.);
#21133=ORIENTED_EDGE('',*,*,#15046,.F.);
#21134=ORIENTED_EDGE('',*,*,#15043,.F.);
#21135=ORIENTED_EDGE('',*,*,#15040,.F.);
#21136=ORIENTED_EDGE('',*,*,#15047,.F.);
#21137=ORIENTED_EDGE('',*,*,#15048,.T.);
#21138=ORIENTED_EDGE('',*,*,#15049,.T.);
#21139=ORIENTED_EDGE('',*,*,#15050,.F.);
#21140=ORIENTED_EDGE('',*,*,#15049,.F.);
#21141=ORIENTED_EDGE('',*,*,#15051,.T.);
#21142=ORIENTED_EDGE('',*,*,#15052,.F.);
#21143=ORIENTED_EDGE('',*,*,#15053,.F.);
#21144=ORIENTED_EDGE('',*,*,#15054,.F.);
#21145=ORIENTED_EDGE('',*,*,#15051,.F.);
#21146=ORIENTED_EDGE('',*,*,#15048,.F.);
#21147=ORIENTED_EDGE('',*,*,#15055,.F.);
#21148=ORIENTED_EDGE('',*,*,#15056,.T.);
#21149=ORIENTED_EDGE('',*,*,#15057,.T.);
#21150=ORIENTED_EDGE('',*,*,#15058,.F.);
#21151=ORIENTED_EDGE('',*,*,#15057,.F.);
#21152=ORIENTED_EDGE('',*,*,#15059,.T.);
#21153=ORIENTED_EDGE('',*,*,#15060,.F.);
#21154=ORIENTED_EDGE('',*,*,#15061,.F.);
#21155=ORIENTED_EDGE('',*,*,#15062,.F.);
#21156=ORIENTED_EDGE('',*,*,#15059,.F.);
#21157=ORIENTED_EDGE('',*,*,#15056,.F.);
#21158=ORIENTED_EDGE('',*,*,#15063,.F.);
#21159=ORIENTED_EDGE('',*,*,#15064,.T.);
#21160=ORIENTED_EDGE('',*,*,#15065,.T.);
#21161=ORIENTED_EDGE('',*,*,#15066,.F.);
#21162=ORIENTED_EDGE('',*,*,#15065,.F.);
#21163=ORIENTED_EDGE('',*,*,#15067,.T.);
#21164=ORIENTED_EDGE('',*,*,#15068,.F.);
#21165=ORIENTED_EDGE('',*,*,#15069,.F.);
#21166=ORIENTED_EDGE('',*,*,#15070,.F.);
#21167=ORIENTED_EDGE('',*,*,#15067,.F.);
#21168=ORIENTED_EDGE('',*,*,#15064,.F.);
#21169=ORIENTED_EDGE('',*,*,#15071,.F.);
#21170=ORIENTED_EDGE('',*,*,#15072,.T.);
#21171=ORIENTED_EDGE('',*,*,#15073,.T.);
#21172=ORIENTED_EDGE('',*,*,#15074,.F.);
#21173=ORIENTED_EDGE('',*,*,#15073,.F.);
#21174=ORIENTED_EDGE('',*,*,#15075,.T.);
#21175=ORIENTED_EDGE('',*,*,#15076,.F.);
#21176=ORIENTED_EDGE('',*,*,#15077,.F.);
#21177=ORIENTED_EDGE('',*,*,#15078,.F.);
#21178=ORIENTED_EDGE('',*,*,#15075,.F.);
#21179=ORIENTED_EDGE('',*,*,#15072,.F.);
#21180=ORIENTED_EDGE('',*,*,#15079,.F.);
#21181=ORIENTED_EDGE('',*,*,#15080,.T.);
#21182=ORIENTED_EDGE('',*,*,#15081,.T.);
#21183=ORIENTED_EDGE('',*,*,#15082,.F.);
#21184=ORIENTED_EDGE('',*,*,#15081,.F.);
#21185=ORIENTED_EDGE('',*,*,#15083,.T.);
#21186=ORIENTED_EDGE('',*,*,#15084,.F.);
#21187=ORIENTED_EDGE('',*,*,#15085,.F.);
#21188=ORIENTED_EDGE('',*,*,#15086,.F.);
#21189=ORIENTED_EDGE('',*,*,#15083,.F.);
#21190=ORIENTED_EDGE('',*,*,#15080,.F.);
#21191=ORIENTED_EDGE('',*,*,#15087,.F.);
#21192=ORIENTED_EDGE('',*,*,#15088,.T.);
#21193=ORIENTED_EDGE('',*,*,#15089,.T.);
#21194=ORIENTED_EDGE('',*,*,#15090,.F.);
#21195=ORIENTED_EDGE('',*,*,#15089,.F.);
#21196=ORIENTED_EDGE('',*,*,#15091,.T.);
#21197=ORIENTED_EDGE('',*,*,#15092,.F.);
#21198=ORIENTED_EDGE('',*,*,#15093,.F.);
#21199=ORIENTED_EDGE('',*,*,#15094,.F.);
#21200=ORIENTED_EDGE('',*,*,#15091,.F.);
#21201=ORIENTED_EDGE('',*,*,#15088,.F.);
#21202=ORIENTED_EDGE('',*,*,#15095,.F.);
#21203=ORIENTED_EDGE('',*,*,#15096,.T.);
#21204=ORIENTED_EDGE('',*,*,#15097,.T.);
#21205=ORIENTED_EDGE('',*,*,#15098,.F.);
#21206=ORIENTED_EDGE('',*,*,#15097,.F.);
#21207=ORIENTED_EDGE('',*,*,#15099,.T.);
#21208=ORIENTED_EDGE('',*,*,#15100,.F.);
#21209=ORIENTED_EDGE('',*,*,#15101,.F.);
#21210=ORIENTED_EDGE('',*,*,#15102,.F.);
#21211=ORIENTED_EDGE('',*,*,#15099,.F.);
#21212=ORIENTED_EDGE('',*,*,#15096,.F.);
#21213=ORIENTED_EDGE('',*,*,#15103,.F.);
#21214=ORIENTED_EDGE('',*,*,#15104,.T.);
#21215=ORIENTED_EDGE('',*,*,#15105,.T.);
#21216=ORIENTED_EDGE('',*,*,#15106,.F.);
#21217=ORIENTED_EDGE('',*,*,#15105,.F.);
#21218=ORIENTED_EDGE('',*,*,#15107,.T.);
#21219=ORIENTED_EDGE('',*,*,#15108,.F.);
#21220=ORIENTED_EDGE('',*,*,#15109,.F.);
#21221=ORIENTED_EDGE('',*,*,#15110,.F.);
#21222=ORIENTED_EDGE('',*,*,#15107,.F.);
#21223=ORIENTED_EDGE('',*,*,#15104,.F.);
#21224=ORIENTED_EDGE('',*,*,#14836,.T.);
#21225=ORIENTED_EDGE('',*,*,#14830,.T.);
#21226=ORIENTED_EDGE('',*,*,#14833,.T.);
#21227=ORIENTED_EDGE('',*,*,#15111,.F.);
#21228=ORIENTED_EDGE('',*,*,#14844,.T.);
#21229=ORIENTED_EDGE('',*,*,#14838,.T.);
#21230=ORIENTED_EDGE('',*,*,#14841,.T.);
#21231=ORIENTED_EDGE('',*,*,#15112,.F.);
#21232=ORIENTED_EDGE('',*,*,#14852,.T.);
#21233=ORIENTED_EDGE('',*,*,#14846,.T.);
#21234=ORIENTED_EDGE('',*,*,#14849,.T.);
#21235=ORIENTED_EDGE('',*,*,#15113,.F.);
#21236=ORIENTED_EDGE('',*,*,#14860,.T.);
#21237=ORIENTED_EDGE('',*,*,#14854,.T.);
#21238=ORIENTED_EDGE('',*,*,#14857,.T.);
#21239=ORIENTED_EDGE('',*,*,#15114,.F.);
#21240=ORIENTED_EDGE('',*,*,#14868,.T.);
#21241=ORIENTED_EDGE('',*,*,#14862,.T.);
#21242=ORIENTED_EDGE('',*,*,#14865,.T.);
#21243=ORIENTED_EDGE('',*,*,#15115,.F.);
#21244=ORIENTED_EDGE('',*,*,#14876,.T.);
#21245=ORIENTED_EDGE('',*,*,#14870,.T.);
#21246=ORIENTED_EDGE('',*,*,#14873,.T.);
#21247=ORIENTED_EDGE('',*,*,#15116,.F.);
#21248=ORIENTED_EDGE('',*,*,#14884,.T.);
#21249=ORIENTED_EDGE('',*,*,#14878,.T.);
#21250=ORIENTED_EDGE('',*,*,#14881,.T.);
#21251=ORIENTED_EDGE('',*,*,#15117,.F.);
#21252=ORIENTED_EDGE('',*,*,#14892,.T.);
#21253=ORIENTED_EDGE('',*,*,#14886,.T.);
#21254=ORIENTED_EDGE('',*,*,#14889,.T.);
#21255=ORIENTED_EDGE('',*,*,#15118,.F.);
#21256=ORIENTED_EDGE('',*,*,#14900,.T.);
#21257=ORIENTED_EDGE('',*,*,#14894,.T.);
#21258=ORIENTED_EDGE('',*,*,#14897,.T.);
#21259=ORIENTED_EDGE('',*,*,#15119,.F.);
#21260=ORIENTED_EDGE('',*,*,#14908,.T.);
#21261=ORIENTED_EDGE('',*,*,#14902,.T.);
#21262=ORIENTED_EDGE('',*,*,#14905,.T.);
#21263=ORIENTED_EDGE('',*,*,#15120,.F.);
#21264=ORIENTED_EDGE('',*,*,#14916,.T.);
#21265=ORIENTED_EDGE('',*,*,#14910,.T.);
#21266=ORIENTED_EDGE('',*,*,#14913,.T.);
#21267=ORIENTED_EDGE('',*,*,#15121,.F.);
#21268=ORIENTED_EDGE('',*,*,#14924,.T.);
#21269=ORIENTED_EDGE('',*,*,#14918,.T.);
#21270=ORIENTED_EDGE('',*,*,#14921,.T.);
#21271=ORIENTED_EDGE('',*,*,#15122,.F.);
#21272=ORIENTED_EDGE('',*,*,#14932,.T.);
#21273=ORIENTED_EDGE('',*,*,#14926,.T.);
#21274=ORIENTED_EDGE('',*,*,#14929,.T.);
#21275=ORIENTED_EDGE('',*,*,#15123,.F.);
#21276=ORIENTED_EDGE('',*,*,#14940,.T.);
#21277=ORIENTED_EDGE('',*,*,#14934,.T.);
#21278=ORIENTED_EDGE('',*,*,#14937,.T.);
#21279=ORIENTED_EDGE('',*,*,#15124,.F.);
#21280=ORIENTED_EDGE('',*,*,#14948,.T.);
#21281=ORIENTED_EDGE('',*,*,#14942,.T.);
#21282=ORIENTED_EDGE('',*,*,#14945,.T.);
#21283=ORIENTED_EDGE('',*,*,#15125,.F.);
#21284=ORIENTED_EDGE('',*,*,#14956,.T.);
#21285=ORIENTED_EDGE('',*,*,#14950,.T.);
#21286=ORIENTED_EDGE('',*,*,#14953,.T.);
#21287=ORIENTED_EDGE('',*,*,#15126,.F.);
#21288=ORIENTED_EDGE('',*,*,#14964,.T.);
#21289=ORIENTED_EDGE('',*,*,#14958,.T.);
#21290=ORIENTED_EDGE('',*,*,#14961,.T.);
#21291=ORIENTED_EDGE('',*,*,#15127,.F.);
#21292=ORIENTED_EDGE('',*,*,#14973,.T.);
#21293=ORIENTED_EDGE('',*,*,#14966,.T.);
#21294=ORIENTED_EDGE('',*,*,#15128,.T.);
#21295=ORIENTED_EDGE('',*,*,#15129,.T.);
#21296=ORIENTED_EDGE('',*,*,#15128,.F.);
#21297=ORIENTED_EDGE('',*,*,#14969,.T.);
#21298=ORIENTED_EDGE('',*,*,#14970,.T.);
#21299=ORIENTED_EDGE('',*,*,#15130,.F.);
#21300=ORIENTED_EDGE('',*,*,#14981,.T.);
#21301=ORIENTED_EDGE('',*,*,#14975,.T.);
#21302=ORIENTED_EDGE('',*,*,#14978,.T.);
#21303=ORIENTED_EDGE('',*,*,#15131,.F.);
#21304=ORIENTED_EDGE('',*,*,#14989,.T.);
#21305=ORIENTED_EDGE('',*,*,#14983,.T.);
#21306=ORIENTED_EDGE('',*,*,#14986,.T.);
#21307=ORIENTED_EDGE('',*,*,#15132,.F.);
#21308=ORIENTED_EDGE('',*,*,#14997,.T.);
#21309=ORIENTED_EDGE('',*,*,#14991,.T.);
#21310=ORIENTED_EDGE('',*,*,#14994,.T.);
#21311=ORIENTED_EDGE('',*,*,#15133,.F.);
#21312=ORIENTED_EDGE('',*,*,#15005,.T.);
#21313=ORIENTED_EDGE('',*,*,#14999,.T.);
#21314=ORIENTED_EDGE('',*,*,#15002,.T.);
#21315=ORIENTED_EDGE('',*,*,#15134,.F.);
#21316=ORIENTED_EDGE('',*,*,#15013,.T.);
#21317=ORIENTED_EDGE('',*,*,#15007,.T.);
#21318=ORIENTED_EDGE('',*,*,#15010,.T.);
#21319=ORIENTED_EDGE('',*,*,#15135,.F.);
#21320=ORIENTED_EDGE('',*,*,#15021,.T.);
#21321=ORIENTED_EDGE('',*,*,#15015,.T.);
#21322=ORIENTED_EDGE('',*,*,#15018,.T.);
#21323=ORIENTED_EDGE('',*,*,#15136,.F.);
#21324=ORIENTED_EDGE('',*,*,#15029,.T.);
#21325=ORIENTED_EDGE('',*,*,#15023,.T.);
#21326=ORIENTED_EDGE('',*,*,#15026,.T.);
#21327=ORIENTED_EDGE('',*,*,#15137,.F.);
#21328=ORIENTED_EDGE('',*,*,#15037,.T.);
#21329=ORIENTED_EDGE('',*,*,#15031,.T.);
#21330=ORIENTED_EDGE('',*,*,#15034,.T.);
#21331=ORIENTED_EDGE('',*,*,#15138,.F.);
#21332=ORIENTED_EDGE('',*,*,#15045,.T.);
#21333=ORIENTED_EDGE('',*,*,#15039,.T.);
#21334=ORIENTED_EDGE('',*,*,#15042,.T.);
#21335=ORIENTED_EDGE('',*,*,#15139,.F.);
#21336=ORIENTED_EDGE('',*,*,#15053,.T.);
#21337=ORIENTED_EDGE('',*,*,#15047,.T.);
#21338=ORIENTED_EDGE('',*,*,#15050,.T.);
#21339=ORIENTED_EDGE('',*,*,#15140,.F.);
#21340=ORIENTED_EDGE('',*,*,#15061,.T.);
#21341=ORIENTED_EDGE('',*,*,#15055,.T.);
#21342=ORIENTED_EDGE('',*,*,#15058,.T.);
#21343=ORIENTED_EDGE('',*,*,#15141,.F.);
#21344=ORIENTED_EDGE('',*,*,#15069,.T.);
#21345=ORIENTED_EDGE('',*,*,#15063,.T.);
#21346=ORIENTED_EDGE('',*,*,#15066,.T.);
#21347=ORIENTED_EDGE('',*,*,#15142,.F.);
#21348=ORIENTED_EDGE('',*,*,#15077,.T.);
#21349=ORIENTED_EDGE('',*,*,#15071,.T.);
#21350=ORIENTED_EDGE('',*,*,#15074,.T.);
#21351=ORIENTED_EDGE('',*,*,#15143,.F.);
#21352=ORIENTED_EDGE('',*,*,#15085,.T.);
#21353=ORIENTED_EDGE('',*,*,#15079,.T.);
#21354=ORIENTED_EDGE('',*,*,#15082,.T.);
#21355=ORIENTED_EDGE('',*,*,#15144,.F.);
#21356=ORIENTED_EDGE('',*,*,#15093,.T.);
#21357=ORIENTED_EDGE('',*,*,#15087,.T.);
#21358=ORIENTED_EDGE('',*,*,#15090,.T.);
#21359=ORIENTED_EDGE('',*,*,#15145,.F.);
#21360=ORIENTED_EDGE('',*,*,#15101,.T.);
#21361=ORIENTED_EDGE('',*,*,#15095,.T.);
#21362=ORIENTED_EDGE('',*,*,#15098,.T.);
#21363=ORIENTED_EDGE('',*,*,#15146,.F.);
#21364=ORIENTED_EDGE('',*,*,#15109,.T.);
#21365=ORIENTED_EDGE('',*,*,#15103,.T.);
#21366=ORIENTED_EDGE('',*,*,#15106,.T.);
#21367=ORIENTED_EDGE('',*,*,#15147,.F.);
#21368=ORIENTED_EDGE('',*,*,#15148,.T.);
#21369=ORIENTED_EDGE('',*,*,#15149,.T.);
#21370=ORIENTED_EDGE('',*,*,#15150,.T.);
#21371=ORIENTED_EDGE('',*,*,#15151,.F.);
#21372=ORIENTED_EDGE('',*,*,#15150,.F.);
#21373=ORIENTED_EDGE('',*,*,#15152,.F.);
#21374=ORIENTED_EDGE('',*,*,#15153,.T.);
#21375=ORIENTED_EDGE('',*,*,#15154,.F.);
#21376=ORIENTED_EDGE('',*,*,#15155,.F.);
#21377=ORIENTED_EDGE('',*,*,#15153,.F.);
#21378=ORIENTED_EDGE('',*,*,#15156,.F.);
#21379=ORIENTED_EDGE('',*,*,#15148,.F.);
#21380=ORIENTED_EDGE('',*,*,#15149,.F.);
#21381=ORIENTED_EDGE('',*,*,#15156,.T.);
#21382=ORIENTED_EDGE('',*,*,#15152,.T.);
#21383=ORIENTED_EDGE('',*,*,#15157,.F.);
#21384=ORIENTED_EDGE('',*,*,#15158,.T.);
#21385=ORIENTED_EDGE('',*,*,#14974,.T.);
#21386=ORIENTED_EDGE('',*,*,#15127,.T.);
#21387=ORIENTED_EDGE('',*,*,#14963,.T.);
#21388=ORIENTED_EDGE('',*,*,#14965,.T.);
#21389=ORIENTED_EDGE('',*,*,#15126,.T.);
#21390=ORIENTED_EDGE('',*,*,#14955,.T.);
#21391=ORIENTED_EDGE('',*,*,#14957,.T.);
#21392=ORIENTED_EDGE('',*,*,#15125,.T.);
#21393=ORIENTED_EDGE('',*,*,#14947,.T.);
#21394=ORIENTED_EDGE('',*,*,#14949,.T.);
#21395=ORIENTED_EDGE('',*,*,#15124,.T.);
#21396=ORIENTED_EDGE('',*,*,#14939,.T.);
#21397=ORIENTED_EDGE('',*,*,#14941,.T.);
#21398=ORIENTED_EDGE('',*,*,#15123,.T.);
#21399=ORIENTED_EDGE('',*,*,#14931,.T.);
#21400=ORIENTED_EDGE('',*,*,#14933,.T.);
#21401=ORIENTED_EDGE('',*,*,#15122,.T.);
#21402=ORIENTED_EDGE('',*,*,#14923,.T.);
#21403=ORIENTED_EDGE('',*,*,#14925,.T.);
#21404=ORIENTED_EDGE('',*,*,#15121,.T.);
#21405=ORIENTED_EDGE('',*,*,#14915,.T.);
#21406=ORIENTED_EDGE('',*,*,#14917,.T.);
#21407=ORIENTED_EDGE('',*,*,#15120,.T.);
#21408=ORIENTED_EDGE('',*,*,#14907,.T.);
#21409=ORIENTED_EDGE('',*,*,#14909,.T.);
#21410=ORIENTED_EDGE('',*,*,#15119,.T.);
#21411=ORIENTED_EDGE('',*,*,#14899,.T.);
#21412=ORIENTED_EDGE('',*,*,#14901,.T.);
#21413=ORIENTED_EDGE('',*,*,#15118,.T.);
#21414=ORIENTED_EDGE('',*,*,#14891,.T.);
#21415=ORIENTED_EDGE('',*,*,#14893,.T.);
#21416=ORIENTED_EDGE('',*,*,#15117,.T.);
#21417=ORIENTED_EDGE('',*,*,#14883,.T.);
#21418=ORIENTED_EDGE('',*,*,#14885,.T.);
#21419=ORIENTED_EDGE('',*,*,#15116,.T.);
#21420=ORIENTED_EDGE('',*,*,#14875,.T.);
#21421=ORIENTED_EDGE('',*,*,#14877,.T.);
#21422=ORIENTED_EDGE('',*,*,#15115,.T.);
#21423=ORIENTED_EDGE('',*,*,#14867,.T.);
#21424=ORIENTED_EDGE('',*,*,#14869,.T.);
#21425=ORIENTED_EDGE('',*,*,#15114,.T.);
#21426=ORIENTED_EDGE('',*,*,#14859,.T.);
#21427=ORIENTED_EDGE('',*,*,#14861,.T.);
#21428=ORIENTED_EDGE('',*,*,#15113,.T.);
#21429=ORIENTED_EDGE('',*,*,#14851,.T.);
#21430=ORIENTED_EDGE('',*,*,#14853,.T.);
#21431=ORIENTED_EDGE('',*,*,#15112,.T.);
#21432=ORIENTED_EDGE('',*,*,#14843,.T.);
#21433=ORIENTED_EDGE('',*,*,#14845,.T.);
#21434=ORIENTED_EDGE('',*,*,#15111,.T.);
#21435=ORIENTED_EDGE('',*,*,#14835,.T.);
#21436=ORIENTED_EDGE('',*,*,#14837,.T.);
#21437=ORIENTED_EDGE('',*,*,#15151,.T.);
#21438=ORIENTED_EDGE('',*,*,#15154,.T.);
#21439=ORIENTED_EDGE('',*,*,#15155,.T.);
#21440=ORIENTED_EDGE('',*,*,#15147,.T.);
#21441=ORIENTED_EDGE('',*,*,#15108,.T.);
#21442=ORIENTED_EDGE('',*,*,#15110,.T.);
#21443=ORIENTED_EDGE('',*,*,#15146,.T.);
#21444=ORIENTED_EDGE('',*,*,#15100,.T.);
#21445=ORIENTED_EDGE('',*,*,#15102,.T.);
#21446=ORIENTED_EDGE('',*,*,#15145,.T.);
#21447=ORIENTED_EDGE('',*,*,#15092,.T.);
#21448=ORIENTED_EDGE('',*,*,#15094,.T.);
#21449=ORIENTED_EDGE('',*,*,#15144,.T.);
#21450=ORIENTED_EDGE('',*,*,#15084,.T.);
#21451=ORIENTED_EDGE('',*,*,#15086,.T.);
#21452=ORIENTED_EDGE('',*,*,#15143,.T.);
#21453=ORIENTED_EDGE('',*,*,#15076,.T.);
#21454=ORIENTED_EDGE('',*,*,#15078,.T.);
#21455=ORIENTED_EDGE('',*,*,#15142,.T.);
#21456=ORIENTED_EDGE('',*,*,#15068,.T.);
#21457=ORIENTED_EDGE('',*,*,#15070,.T.);
#21458=ORIENTED_EDGE('',*,*,#15141,.T.);
#21459=ORIENTED_EDGE('',*,*,#15060,.T.);
#21460=ORIENTED_EDGE('',*,*,#15062,.T.);
#21461=ORIENTED_EDGE('',*,*,#15140,.T.);
#21462=ORIENTED_EDGE('',*,*,#15052,.T.);
#21463=ORIENTED_EDGE('',*,*,#15054,.T.);
#21464=ORIENTED_EDGE('',*,*,#15139,.T.);
#21465=ORIENTED_EDGE('',*,*,#15044,.T.);
#21466=ORIENTED_EDGE('',*,*,#15046,.T.);
#21467=ORIENTED_EDGE('',*,*,#15138,.T.);
#21468=ORIENTED_EDGE('',*,*,#15036,.T.);
#21469=ORIENTED_EDGE('',*,*,#15038,.T.);
#21470=ORIENTED_EDGE('',*,*,#15137,.T.);
#21471=ORIENTED_EDGE('',*,*,#15028,.T.);
#21472=ORIENTED_EDGE('',*,*,#15030,.T.);
#21473=ORIENTED_EDGE('',*,*,#15136,.T.);
#21474=ORIENTED_EDGE('',*,*,#15020,.T.);
#21475=ORIENTED_EDGE('',*,*,#15022,.T.);
#21476=ORIENTED_EDGE('',*,*,#15135,.T.);
#21477=ORIENTED_EDGE('',*,*,#15012,.T.);
#21478=ORIENTED_EDGE('',*,*,#15014,.T.);
#21479=ORIENTED_EDGE('',*,*,#15134,.T.);
#21480=ORIENTED_EDGE('',*,*,#15004,.T.);
#21481=ORIENTED_EDGE('',*,*,#15006,.T.);
#21482=ORIENTED_EDGE('',*,*,#15133,.T.);
#21483=ORIENTED_EDGE('',*,*,#14996,.T.);
#21484=ORIENTED_EDGE('',*,*,#14998,.T.);
#21485=ORIENTED_EDGE('',*,*,#15132,.T.);
#21486=ORIENTED_EDGE('',*,*,#14988,.T.);
#21487=ORIENTED_EDGE('',*,*,#14990,.T.);
#21488=ORIENTED_EDGE('',*,*,#15131,.T.);
#21489=ORIENTED_EDGE('',*,*,#14980,.T.);
#21490=ORIENTED_EDGE('',*,*,#14982,.T.);
#21491=ORIENTED_EDGE('',*,*,#15130,.T.);
#21492=ORIENTED_EDGE('',*,*,#14972,.T.);
#21493=ORIENTED_EDGE('',*,*,#15158,.F.);
#21494=ORIENTED_EDGE('',*,*,#15159,.T.);
#21495=ORIENTED_EDGE('',*,*,#15160,.F.);
#21496=ORIENTED_EDGE('',*,*,#15159,.F.);
#21497=ORIENTED_EDGE('',*,*,#15161,.F.);
#21498=ORIENTED_EDGE('',*,*,#15162,.T.);
#21499=ORIENTED_EDGE('',*,*,#15163,.T.);
#21500=ORIENTED_EDGE('',*,*,#15164,.F.);
#21501=ORIENTED_EDGE('',*,*,#15165,.F.);
#21502=ORIENTED_EDGE('',*,*,#15166,.T.);
#21503=ORIENTED_EDGE('',*,*,#15167,.T.);
#21504=ORIENTED_EDGE('',*,*,#15162,.F.);
#21505=ORIENTED_EDGE('',*,*,#15168,.F.);
#21506=ORIENTED_EDGE('',*,*,#15169,.T.);
#21507=ORIENTED_EDGE('',*,*,#15170,.T.);
#21508=ORIENTED_EDGE('',*,*,#15166,.F.);
#21509=ORIENTED_EDGE('',*,*,#15171,.F.);
#21510=ORIENTED_EDGE('',*,*,#15172,.T.);
#21511=ORIENTED_EDGE('',*,*,#15173,.T.);
#21512=ORIENTED_EDGE('',*,*,#15169,.F.);
#21513=ORIENTED_EDGE('',*,*,#15174,.F.);
#21514=ORIENTED_EDGE('',*,*,#15175,.T.);
#21515=ORIENTED_EDGE('',*,*,#15176,.T.);
#21516=ORIENTED_EDGE('',*,*,#15172,.F.);
#21517=ORIENTED_EDGE('',*,*,#15177,.F.);
#21518=ORIENTED_EDGE('',*,*,#15164,.T.);
#21519=ORIENTED_EDGE('',*,*,#15178,.T.);
#21520=ORIENTED_EDGE('',*,*,#15175,.F.);
#21521=ORIENTED_EDGE('',*,*,#15178,.F.);
#21522=ORIENTED_EDGE('',*,*,#15163,.F.);
#21523=ORIENTED_EDGE('',*,*,#15167,.F.);
#21524=ORIENTED_EDGE('',*,*,#15170,.F.);
#21525=ORIENTED_EDGE('',*,*,#15173,.F.);
#21526=ORIENTED_EDGE('',*,*,#15176,.F.);
#21527=ORIENTED_EDGE('',*,*,#15160,.T.);
#21528=ORIENTED_EDGE('',*,*,#15179,.F.);
#21529=ORIENTED_EDGE('',*,*,#14677,.F.);
#21530=ORIENTED_EDGE('',*,*,#15180,.T.);
#21531=ORIENTED_EDGE('',*,*,#15179,.T.);
#21532=ORIENTED_EDGE('',*,*,#15180,.F.);
#21533=ORIENTED_EDGE('',*,*,#14743,.T.);
#21534=ORIENTED_EDGE('',*,*,#14824,.T.);
#21535=ORIENTED_EDGE('',*,*,#15181,.F.);
#21536=ORIENTED_EDGE('',*,*,#14829,.T.);
#21537=ORIENTED_EDGE('',*,*,#15182,.F.);
#21538=ORIENTED_EDGE('',*,*,#15183,.T.);
#21539=ORIENTED_EDGE('',*,*,#14821,.T.);
#21540=ORIENTED_EDGE('',*,*,#15181,.T.);
#21541=ORIENTED_EDGE('',*,*,#14822,.T.);
#21542=ORIENTED_EDGE('',*,*,#15183,.F.);
#21543=ORIENTED_EDGE('',*,*,#15129,.F.);
#21544=ORIENTED_EDGE('',*,*,#15182,.T.);
#21545=ORIENTED_EDGE('',*,*,#15157,.T.);
#21546=ORIENTED_EDGE('',*,*,#15161,.T.);
#21547=ORIENTED_EDGE('',*,*,#15177,.T.);
#21548=ORIENTED_EDGE('',*,*,#15174,.T.);
#21549=ORIENTED_EDGE('',*,*,#15171,.T.);
#21550=ORIENTED_EDGE('',*,*,#15168,.T.);
#21551=ORIENTED_EDGE('',*,*,#15165,.T.);
#23153=CONICAL_SURFACE('',#26766,0.1825,0.785398163397448);
#23154=CONICAL_SURFACE('',#26768,0.0346410161513776,1.00188494390461);
#23155=CONICAL_SURFACE('',#26779,0.088,0.785398163397448);
#23156=CONICAL_SURFACE('',#26782,0.105,0.785398163397449);
#24104=ADVANCED_FACE('',(#3351),#2281,.T.);
#24105=ADVANCED_FACE('',(#3352),#2282,.T.);
#24106=ADVANCED_FACE('',(#3353),#2283,.T.);
#24107=ADVANCED_FACE('',(#3354),#2284,.T.);
#24108=ADVANCED_FACE('',(#3355),#2285,.T.);
#24109=ADVANCED_FACE('',(#3356),#2286,.T.);
#24110=ADVANCED_FACE('',(#3357),#2287,.T.);
#24111=ADVANCED_FACE('',(#3358),#2288,.T.);
#24112=ADVANCED_FACE('',(#3359),#2289,.T.);
#24113=ADVANCED_FACE('',(#3360),#2290,.T.);
#24114=ADVANCED_FACE('',(#3361),#2291,.T.);
#24115=ADVANCED_FACE('',(#3362),#2292,.T.);
#24116=ADVANCED_FACE('',(#3363),#2293,.T.);
#24117=ADVANCED_FACE('',(#3364),#2294,.T.);
#24118=ADVANCED_FACE('',(#3365),#2295,.T.);
#24119=ADVANCED_FACE('',(#3366),#2296,.T.);
#24120=ADVANCED_FACE('',(#3367),#2297,.T.);
#24121=ADVANCED_FACE('',(#3368),#2298,.T.);
#24122=ADVANCED_FACE('',(#3369),#2299,.T.);
#24123=ADVANCED_FACE('',(#3370),#2300,.T.);
#24124=ADVANCED_FACE('',(#3371),#2301,.T.);
#24125=ADVANCED_FACE('',(#3372),#2302,.T.);
#24126=ADVANCED_FACE('',(#3373),#2303,.T.);
#24127=ADVANCED_FACE('',(#3374),#2304,.T.);
#24128=ADVANCED_FACE('',(#3375),#2305,.T.);
#24129=ADVANCED_FACE('',(#3376),#2306,.T.);
#24130=ADVANCED_FACE('',(#3377),#2307,.T.);
#24131=ADVANCED_FACE('',(#3378),#2308,.T.);
#24132=ADVANCED_FACE('',(#3379),#2309,.T.);
#24133=ADVANCED_FACE('',(#3380),#2310,.T.);
#24134=ADVANCED_FACE('',(#3381),#2311,.T.);
#24135=ADVANCED_FACE('',(#3382),#2312,.T.);
#24136=ADVANCED_FACE('',(#3383),#2313,.T.);
#24137=ADVANCED_FACE('',(#3384),#2314,.T.);
#24138=ADVANCED_FACE('',(#3385),#2315,.T.);
#24139=ADVANCED_FACE('',(#3386),#2316,.T.);
#24140=ADVANCED_FACE('',(#3387),#2317,.T.);
#24141=ADVANCED_FACE('',(#3388),#2318,.T.);
#24142=ADVANCED_FACE('',(#3389),#2319,.T.);
#24143=ADVANCED_FACE('',(#3390),#2320,.T.);
#24144=ADVANCED_FACE('',(#3391),#2321,.T.);
#24145=ADVANCED_FACE('',(#3392),#2322,.T.);
#24146=ADVANCED_FACE('',(#3393),#2323,.T.);
#24147=ADVANCED_FACE('',(#3394),#2324,.T.);
#24148=ADVANCED_FACE('',(#3395),#2325,.T.);
#24149=ADVANCED_FACE('',(#3396),#2326,.T.);
#24150=ADVANCED_FACE('',(#3397),#2327,.T.);
#24151=ADVANCED_FACE('',(#3398),#1678,.F.);
#24152=ADVANCED_FACE('',(#3399),#476,.F.);
#24153=ADVANCED_FACE('',(#3400),#1679,.T.);
#24154=ADVANCED_FACE('',(#3401),#2328,.T.);
#24155=ADVANCED_FACE('',(#3402),#477,.F.);
#24156=ADVANCED_FACE('',(#3403),#1680,.T.);
#24157=ADVANCED_FACE('',(#3404),#1681,.F.);
#24158=ADVANCED_FACE('',(#3405),#1682,.F.);
#24159=ADVANCED_FACE('',(#3406),#1683,.T.);
#24160=ADVANCED_FACE('',(#3407),#1684,.F.);
#24161=ADVANCED_FACE('',(#3408),#1685,.F.);
#24162=ADVANCED_FACE('',(#3409),#1686,.T.);
#24163=ADVANCED_FACE('',(#3410),#1687,.F.);
#24164=ADVANCED_FACE('',(#3411),#1688,.F.);
#24165=ADVANCED_FACE('',(#3412),#1689,.T.);
#24166=ADVANCED_FACE('',(#3413),#1690,.F.);
#24167=ADVANCED_FACE('',(#3414),#1691,.F.);
#24168=ADVANCED_FACE('',(#3415),#1692,.T.);
#24169=ADVANCED_FACE('',(#3416),#1693,.F.);
#24170=ADVANCED_FACE('',(#3417),#1694,.F.);
#24171=ADVANCED_FACE('',(#3418),#1695,.T.);
#24172=ADVANCED_FACE('',(#3419),#1696,.F.);
#24173=ADVANCED_FACE('',(#3420),#1697,.F.);
#24174=ADVANCED_FACE('',(#3421),#1698,.T.);
#24175=ADVANCED_FACE('',(#3422),#1699,.F.);
#24176=ADVANCED_FACE('',(#3423),#1700,.F.);
#24177=ADVANCED_FACE('',(#3424),#1701,.T.);
#24178=ADVANCED_FACE('',(#3425),#1702,.F.);
#24179=ADVANCED_FACE('',(#3426),#1703,.F.);
#24180=ADVANCED_FACE('',(#3427),#1704,.T.);
#24181=ADVANCED_FACE('',(#3428),#1705,.F.);
#24182=ADVANCED_FACE('',(#3429),#1706,.F.);
#24183=ADVANCED_FACE('',(#3430),#1707,.T.);
#24184=ADVANCED_FACE('',(#3431),#1708,.F.);
#24185=ADVANCED_FACE('',(#3432),#1709,.F.);
#24186=ADVANCED_FACE('',(#3433),#1710,.T.);
#24187=ADVANCED_FACE('',(#3434),#1711,.F.);
#24188=ADVANCED_FACE('',(#3435),#1712,.F.);
#24189=ADVANCED_FACE('',(#3436),#1713,.T.);
#24190=ADVANCED_FACE('',(#3437),#1714,.F.);
#24191=ADVANCED_FACE('',(#3438),#1715,.F.);
#24192=ADVANCED_FACE('',(#3439),#1716,.T.);
#24193=ADVANCED_FACE('',(#3440),#1717,.F.);
#24194=ADVANCED_FACE('',(#3441),#1718,.F.);
#24195=ADVANCED_FACE('',(#3442),#1719,.T.);
#24196=ADVANCED_FACE('',(#3443),#1720,.F.);
#24197=ADVANCED_FACE('',(#3444),#1721,.F.);
#24198=ADVANCED_FACE('',(#3445),#1722,.T.);
#24199=ADVANCED_FACE('',(#3446),#1723,.F.);
#24200=ADVANCED_FACE('',(#3447),#1724,.F.);
#24201=ADVANCED_FACE('',(#3448),#1725,.T.);
#24202=ADVANCED_FACE('',(#3449),#1726,.F.);
#24203=ADVANCED_FACE('',(#3450),#1727,.F.);
#24204=ADVANCED_FACE('',(#3451),#1728,.T.);
#24205=ADVANCED_FACE('',(#3452),#1729,.F.);
#24206=ADVANCED_FACE('',(#3453),#1730,.F.);
#24207=ADVANCED_FACE('',(#3454),#1731,.T.);
#24208=ADVANCED_FACE('',(#3455),#1732,.F.);
#24209=ADVANCED_FACE('',(#3456),#1733,.F.);
#24210=ADVANCED_FACE('',(#3457),#1734,.T.);
#24211=ADVANCED_FACE('',(#3458),#1735,.F.);
#24212=ADVANCED_FACE('',(#3459),#1736,.F.);
#24213=ADVANCED_FACE('',(#3460),#1737,.T.);
#24214=ADVANCED_FACE('',(#3461),#1738,.F.);
#24215=ADVANCED_FACE('',(#3462),#1739,.F.);
#24216=ADVANCED_FACE('',(#3463),#1740,.T.);
#24217=ADVANCED_FACE('',(#3464),#1741,.F.);
#24218=ADVANCED_FACE('',(#3465),#1742,.F.);
#24219=ADVANCED_FACE('',(#3466),#1743,.T.);
#24220=ADVANCED_FACE('',(#3467),#1744,.F.);
#24221=ADVANCED_FACE('',(#3468),#1745,.F.);
#24222=ADVANCED_FACE('',(#3469),#1746,.T.);
#24223=ADVANCED_FACE('',(#3470),#1747,.F.);
#24224=ADVANCED_FACE('',(#3471),#1748,.F.);
#24225=ADVANCED_FACE('',(#3472),#1749,.T.);
#24226=ADVANCED_FACE('',(#3473),#1750,.F.);
#24227=ADVANCED_FACE('',(#3474),#1751,.F.);
#24228=ADVANCED_FACE('',(#3475),#1752,.T.);
#24229=ADVANCED_FACE('',(#3476),#1753,.F.);
#24230=ADVANCED_FACE('',(#3477),#1754,.F.);
#24231=ADVANCED_FACE('',(#3478),#1755,.T.);
#24232=ADVANCED_FACE('',(#3479),#1756,.F.);
#24233=ADVANCED_FACE('',(#3480),#1757,.F.);
#24234=ADVANCED_FACE('',(#3481),#1758,.T.);
#24235=ADVANCED_FACE('',(#3482),#1759,.F.);
#24236=ADVANCED_FACE('',(#3483),#1760,.F.);
#24237=ADVANCED_FACE('',(#3484),#1761,.T.);
#24238=ADVANCED_FACE('',(#3485),#1762,.F.);
#24239=ADVANCED_FACE('',(#3486),#1763,.F.);
#24240=ADVANCED_FACE('',(#3487),#1764,.T.);
#24241=ADVANCED_FACE('',(#3488),#1765,.F.);
#24242=ADVANCED_FACE('',(#3489),#1766,.F.);
#24243=ADVANCED_FACE('',(#3490),#1767,.T.);
#24244=ADVANCED_FACE('',(#3491),#1768,.F.);
#24245=ADVANCED_FACE('',(#3492),#1769,.F.);
#24246=ADVANCED_FACE('',(#3493),#1770,.T.);
#24247=ADVANCED_FACE('',(#3494),#1771,.F.);
#24248=ADVANCED_FACE('',(#3495),#1772,.F.);
#24249=ADVANCED_FACE('',(#3496),#1773,.T.);
#24250=ADVANCED_FACE('',(#3497),#1774,.F.);
#24251=ADVANCED_FACE('',(#3498),#1775,.F.);
#24252=ADVANCED_FACE('',(#3499),#1776,.T.);
#24253=ADVANCED_FACE('',(#3500),#1777,.F.);
#24254=ADVANCED_FACE('',(#3501),#1778,.F.);
#24255=ADVANCED_FACE('',(#3502),#1779,.T.);
#24256=ADVANCED_FACE('',(#3503),#1780,.F.);
#24257=ADVANCED_FACE('',(#3504),#1781,.F.);
#24258=ADVANCED_FACE('',(#3505),#1782,.T.);
#24259=ADVANCED_FACE('',(#3506),#1783,.F.);
#24260=ADVANCED_FACE('',(#3507),#1784,.F.);
#24261=ADVANCED_FACE('',(#3508),#2329,.T.);
#24262=ADVANCED_FACE('',(#3509),#1785,.F.);
#24263=ADVANCED_FACE('',(#3510),#1786,.F.);
#24264=ADVANCED_FACE('',(#3511),#1787,.T.);
#24265=ADVANCED_FACE('',(#3512),#23153,.T.);
#24266=ADVANCED_FACE('',(#3513),#23154,.F.);
#24267=ADVANCED_FACE('',(#3514),#1788,.F.);
#24268=ADVANCED_FACE('',(#3515),#1789,.F.);
#24269=ADVANCED_FACE('',(#3516),#1790,.F.);
#24270=ADVANCED_FACE('',(#3517),#1791,.F.);
#24271=ADVANCED_FACE('',(#3518),#1792,.F.);
#24272=ADVANCED_FACE('',(#3519),#1793,.F.);
#24273=ADVANCED_FACE('',(#3520,#1266),#1794,.F.);
#24274=ADVANCED_FACE('',(#3521),#1795,.T.);
#24275=ADVANCED_FACE('',(#3522),#23155,.T.);
#24276=ADVANCED_FACE('',(#3523),#2330,.T.);
#24277=ADVANCED_FACE('',(#3524),#23156,.T.);
#24278=ADVANCED_FACE('',(#3525,#1267),#1796,.T.);
#24279=ADVANCED_FACE('',(#3526,#1268),#1797,.T.);
#24545=CLOSED_SHELL('',(#24104,#24105,#24106,#24107,#24108,#24109,#24110,
#24111,#24112,#24113,#24114,#24115,#24116,#24117,#24118,#24119,#24120,#24121,
#24122,#24123,#24124,#24125,#24126,#24127,#24128,#24129,#24130,#24131,#24132,
#24133,#24134,#24135,#24136,#24137,#24138,#24139,#24140,#24141,#24142,#24143,
#24144,#24145,#24146,#24147,#24148,#24149,#24150,#24151,#24152,#24153,#24154,
#24155,#24156,#24157,#24158,#24159,#24160,#24161,#24162,#24163,#24164,#24165,
#24166,#24167,#24168,#24169,#24170,#24171,#24172,#24173,#24174,#24175,#24176,
#24177,#24178,#24179,#24180,#24181,#24182,#24183,#24184,#24185,#24186,#24187,
#24188,#24189,#24190,#24191,#24192,#24193,#24194,#24195,#24196,#24197,#24198,
#24199,#24200,#24201,#24202,#24203,#24204,#24205,#24206,#24207,#24208,#24209,
#24210,#24211,#24212,#24213,#24214,#24215,#24216,#24217,#24218,#24219,#24220,
#24221,#24222,#24223,#24224,#24225,#24226,#24227,#24228,#24229,#24230,#24231,
#24232,#24233,#24234,#24235,#24236,#24237,#24238,#24239,#24240,#24241,#24242,
#24243,#24244,#24245,#24246,#24247,#24248,#24249,#24250,#24251,#24252,#24253,
#24254,#24255,#24256,#24257,#24258,#24259,#24260,#24261,#24262,#24263,#24264,
#24265,#24266,#24267,#24268,#24269,#24270,#24271,#24272,#24273,#24274,#24275,
#24276,#24277,#24278,#24279));
#26524=AXIS2_PLACEMENT_3D('',#44628,#31918,#31919);
#26525=AXIS2_PLACEMENT_3D('',#44629,#31920,#31921);
#26526=AXIS2_PLACEMENT_3D('',#44648,#31923,#31924);
#26527=AXIS2_PLACEMENT_3D('',#44651,#31926,#31927);
#26528=AXIS2_PLACEMENT_3D('',#44653,#31928,#31929);
#26529=AXIS2_PLACEMENT_3D('',#44664,#31930,#31931);
#26530=AXIS2_PLACEMENT_3D('',#44718,#31933,#31934);
#26531=AXIS2_PLACEMENT_3D('',#44766,#31936,#31937);
#26532=AXIS2_PLACEMENT_3D('',#44814,#31939,#31940);
#26533=AXIS2_PLACEMENT_3D('',#44862,#31942,#31943);
#26534=AXIS2_PLACEMENT_3D('',#44916,#31945,#31946);
#26535=AXIS2_PLACEMENT_3D('',#44964,#31948,#31949);
#26536=AXIS2_PLACEMENT_3D('',#45012,#31951,#31952);
#26537=AXIS2_PLACEMENT_3D('',#45066,#31954,#31955);
#26538=AXIS2_PLACEMENT_3D('',#45114,#31957,#31958);
#26539=AXIS2_PLACEMENT_3D('',#45162,#31960,#31961);
#26540=AXIS2_PLACEMENT_3D('',#45216,#31963,#31964);
#26541=AXIS2_PLACEMENT_3D('',#45264,#31966,#31967);
#26542=AXIS2_PLACEMENT_3D('',#45312,#31969,#31970);
#26543=AXIS2_PLACEMENT_3D('',#45366,#31972,#31973);
#26544=AXIS2_PLACEMENT_3D('',#45414,#31975,#31976);
#26545=AXIS2_PLACEMENT_3D('',#45462,#31978,#31979);
#26546=AXIS2_PLACEMENT_3D('',#45516,#31981,#31982);
#26547=AXIS2_PLACEMENT_3D('',#45564,#31984,#31985);
#26548=AXIS2_PLACEMENT_3D('',#45612,#31987,#31988);
#26549=AXIS2_PLACEMENT_3D('',#45666,#31990,#31991);
#26550=AXIS2_PLACEMENT_3D('',#45714,#31993,#31994);
#26551=AXIS2_PLACEMENT_3D('',#45762,#31996,#31997);
#26552=AXIS2_PLACEMENT_3D('',#45775,#31999,#32000);
#26553=AXIS2_PLACEMENT_3D('',#45781,#32001,#32002);
#26554=AXIS2_PLACEMENT_3D('',#45806,#32004,#32005);
#26555=AXIS2_PLACEMENT_3D('',#45830,#32007,#32008);
#26556=AXIS2_PLACEMENT_3D('',#45855,#32010,#32011);
#26557=AXIS2_PLACEMENT_3D('',#45880,#32013,#32014);
#26558=AXIS2_PLACEMENT_3D('',#45904,#32016,#32017);
#26559=AXIS2_PLACEMENT_3D('',#45929,#32019,#32020);
#26560=AXIS2_PLACEMENT_3D('',#45954,#32022,#32023);
#26561=AXIS2_PLACEMENT_3D('',#45978,#32025,#32026);
#26562=AXIS2_PLACEMENT_3D('',#46003,#32028,#32029);
#26563=AXIS2_PLACEMENT_3D('',#46028,#32031,#32032);
#26564=AXIS2_PLACEMENT_3D('',#46052,#32034,#32035);
#26565=AXIS2_PLACEMENT_3D('',#46077,#32037,#32038);
#26566=AXIS2_PLACEMENT_3D('',#46102,#32040,#32041);
#26567=AXIS2_PLACEMENT_3D('',#46126,#32043,#32044);
#26568=AXIS2_PLACEMENT_3D('',#46151,#32046,#32047);
#26569=AXIS2_PLACEMENT_3D('',#46176,#32049,#32050);
#26570=AXIS2_PLACEMENT_3D('',#46200,#32052,#32053);
#26571=AXIS2_PLACEMENT_3D('',#46225,#32055,#32056);
#26572=AXIS2_PLACEMENT_3D('',#46250,#32058,#32059);
#26573=AXIS2_PLACEMENT_3D('',#46274,#32061,#32062);
#26574=AXIS2_PLACEMENT_3D('',#46298,#32064,#32065);
#26575=AXIS2_PLACEMENT_3D('',#46323,#32067,#32068);
#26576=AXIS2_PLACEMENT_3D('',#46328,#32070,#32071);
#26577=AXIS2_PLACEMENT_3D('',#46349,#32072,#32073);
#26578=AXIS2_PLACEMENT_3D('',#46398,#32074,#32075);
#26579=AXIS2_PLACEMENT_3D('',#46400,#32076,#32077);
#26580=AXIS2_PLACEMENT_3D('',#47132,#32078,#32079);
#26581=AXIS2_PLACEMENT_3D('',#47179,#32080,#32081);
#26582=AXIS2_PLACEMENT_3D('',#47180,#32082,#32083);
#26583=AXIS2_PLACEMENT_3D('',#47812,#32084,#32085);
#26584=AXIS2_PLACEMENT_3D('',#47815,#32086,#32087);
#26585=AXIS2_PLACEMENT_3D('',#47819,#32090,#32091);
#26586=AXIS2_PLACEMENT_3D('',#47827,#32094,#32095);
#26587=AXIS2_PLACEMENT_3D('',#47833,#32097,#32098);
#26588=AXIS2_PLACEMENT_3D('',#47836,#32099,#32100);
#26589=AXIS2_PLACEMENT_3D('',#47840,#32103,#32104);
#26590=AXIS2_PLACEMENT_3D('',#47848,#32107,#32108);
#26591=AXIS2_PLACEMENT_3D('',#47854,#32110,#32111);
#26592=AXIS2_PLACEMENT_3D('',#47857,#32112,#32113);
#26593=AXIS2_PLACEMENT_3D('',#47861,#32116,#32117);
#26594=AXIS2_PLACEMENT_3D('',#47869,#32120,#32121);
#26595=AXIS2_PLACEMENT_3D('',#47875,#32123,#32124);
#26596=AXIS2_PLACEMENT_3D('',#47878,#32125,#32126);
#26597=AXIS2_PLACEMENT_3D('',#47882,#32129,#32130);
#26598=AXIS2_PLACEMENT_3D('',#47890,#32133,#32134);
#26599=AXIS2_PLACEMENT_3D('',#47896,#32136,#32137);
#26600=AXIS2_PLACEMENT_3D('',#47899,#32138,#32139);
#26601=AXIS2_PLACEMENT_3D('',#47903,#32142,#32143);
#26602=AXIS2_PLACEMENT_3D('',#47911,#32146,#32147);
#26603=AXIS2_PLACEMENT_3D('',#47917,#32149,#32150);
#26604=AXIS2_PLACEMENT_3D('',#47920,#32151,#32152);
#26605=AXIS2_PLACEMENT_3D('',#47924,#32155,#32156);
#26606=AXIS2_PLACEMENT_3D('',#47932,#32159,#32160);
#26607=AXIS2_PLACEMENT_3D('',#47938,#32162,#32163);
#26608=AXIS2_PLACEMENT_3D('',#47941,#32164,#32165);
#26609=AXIS2_PLACEMENT_3D('',#47945,#32168,#32169);
#26610=AXIS2_PLACEMENT_3D('',#47953,#32172,#32173);
#26611=AXIS2_PLACEMENT_3D('',#47959,#32175,#32176);
#26612=AXIS2_PLACEMENT_3D('',#47962,#32177,#32178);
#26613=AXIS2_PLACEMENT_3D('',#47966,#32181,#32182);
#26614=AXIS2_PLACEMENT_3D('',#47974,#32185,#32186);
#26615=AXIS2_PLACEMENT_3D('',#47980,#32188,#32189);
#26616=AXIS2_PLACEMENT_3D('',#47983,#32190,#32191);
#26617=AXIS2_PLACEMENT_3D('',#47987,#32194,#32195);
#26618=AXIS2_PLACEMENT_3D('',#47995,#32198,#32199);
#26619=AXIS2_PLACEMENT_3D('',#48001,#32201,#32202);
#26620=AXIS2_PLACEMENT_3D('',#48004,#32203,#32204);
#26621=AXIS2_PLACEMENT_3D('',#48008,#32207,#32208);
#26622=AXIS2_PLACEMENT_3D('',#48016,#32211,#32212);
#26623=AXIS2_PLACEMENT_3D('',#48022,#32214,#32215);
#26624=AXIS2_PLACEMENT_3D('',#48025,#32216,#32217);
#26625=AXIS2_PLACEMENT_3D('',#48029,#32220,#32221);
#26626=AXIS2_PLACEMENT_3D('',#48037,#32224,#32225);
#26627=AXIS2_PLACEMENT_3D('',#48043,#32227,#32228);
#26628=AXIS2_PLACEMENT_3D('',#48046,#32229,#32230);
#26629=AXIS2_PLACEMENT_3D('',#48050,#32233,#32234);
#26630=AXIS2_PLACEMENT_3D('',#48058,#32237,#32238);
#26631=AXIS2_PLACEMENT_3D('',#48064,#32240,#32241);
#26632=AXIS2_PLACEMENT_3D('',#48067,#32242,#32243);
#26633=AXIS2_PLACEMENT_3D('',#48071,#32246,#32247);
#26634=AXIS2_PLACEMENT_3D('',#48079,#32250,#32251);
#26635=AXIS2_PLACEMENT_3D('',#48085,#32253,#32254);
#26636=AXIS2_PLACEMENT_3D('',#48088,#32255,#32256);
#26637=AXIS2_PLACEMENT_3D('',#48092,#32259,#32260);
#26638=AXIS2_PLACEMENT_3D('',#48100,#32263,#32264);
#26639=AXIS2_PLACEMENT_3D('',#48106,#32266,#32267);
#26640=AXIS2_PLACEMENT_3D('',#48109,#32268,#32269);
#26641=AXIS2_PLACEMENT_3D('',#48113,#32272,#32273);
#26642=AXIS2_PLACEMENT_3D('',#48121,#32276,#32277);
#26643=AXIS2_PLACEMENT_3D('',#48127,#32279,#32280);
#26644=AXIS2_PLACEMENT_3D('',#48130,#32281,#32282);
#26645=AXIS2_PLACEMENT_3D('',#48134,#32285,#32286);
#26646=AXIS2_PLACEMENT_3D('',#48142,#32289,#32290);
#26647=AXIS2_PLACEMENT_3D('',#48148,#32292,#32293);
#26648=AXIS2_PLACEMENT_3D('',#48151,#32294,#32295);
#26649=AXIS2_PLACEMENT_3D('',#48155,#32298,#32299);
#26650=AXIS2_PLACEMENT_3D('',#48163,#32302,#32303);
#26651=AXIS2_PLACEMENT_3D('',#48169,#32305,#32306);
#26652=AXIS2_PLACEMENT_3D('',#48172,#32307,#32308);
#26653=AXIS2_PLACEMENT_3D('',#48177,#32311,#32312);
#26654=AXIS2_PLACEMENT_3D('',#48178,#32313,#32314);
#26655=AXIS2_PLACEMENT_3D('',#48186,#32317,#32318);
#26656=AXIS2_PLACEMENT_3D('',#48192,#32320,#32321);
#26657=AXIS2_PLACEMENT_3D('',#48195,#32322,#32323);
#26658=AXIS2_PLACEMENT_3D('',#48199,#32326,#32327);
#26659=AXIS2_PLACEMENT_3D('',#48207,#32330,#32331);
#26660=AXIS2_PLACEMENT_3D('',#48213,#32333,#32334);
#26661=AXIS2_PLACEMENT_3D('',#48216,#32335,#32336);
#26662=AXIS2_PLACEMENT_3D('',#48220,#32339,#32340);
#26663=AXIS2_PLACEMENT_3D('',#48228,#32343,#32344);
#26664=AXIS2_PLACEMENT_3D('',#48234,#32346,#32347);
#26665=AXIS2_PLACEMENT_3D('',#48237,#32348,#32349);
#26666=AXIS2_PLACEMENT_3D('',#48241,#32352,#32353);
#26667=AXIS2_PLACEMENT_3D('',#48249,#32356,#32357);
#26668=AXIS2_PLACEMENT_3D('',#48255,#32359,#32360);
#26669=AXIS2_PLACEMENT_3D('',#48258,#32361,#32362);
#26670=AXIS2_PLACEMENT_3D('',#48262,#32365,#32366);
#26671=AXIS2_PLACEMENT_3D('',#48270,#32369,#32370);
#26672=AXIS2_PLACEMENT_3D('',#48276,#32372,#32373);
#26673=AXIS2_PLACEMENT_3D('',#48279,#32374,#32375);
#26674=AXIS2_PLACEMENT_3D('',#48283,#32378,#32379);
#26675=AXIS2_PLACEMENT_3D('',#48291,#32382,#32383);
#26676=AXIS2_PLACEMENT_3D('',#48297,#32385,#32386);
#26677=AXIS2_PLACEMENT_3D('',#48300,#32387,#32388);
#26678=AXIS2_PLACEMENT_3D('',#48304,#32391,#32392);
#26679=AXIS2_PLACEMENT_3D('',#48312,#32395,#32396);
#26680=AXIS2_PLACEMENT_3D('',#48318,#32398,#32399);
#26681=AXIS2_PLACEMENT_3D('',#48321,#32400,#32401);
#26682=AXIS2_PLACEMENT_3D('',#48325,#32404,#32405);
#26683=AXIS2_PLACEMENT_3D('',#48333,#32408,#32409);
#26684=AXIS2_PLACEMENT_3D('',#48339,#32411,#32412);
#26685=AXIS2_PLACEMENT_3D('',#48342,#32413,#32414);
#26686=AXIS2_PLACEMENT_3D('',#48346,#32417,#32418);
#26687=AXIS2_PLACEMENT_3D('',#48354,#32421,#32422);
#26688=AXIS2_PLACEMENT_3D('',#48360,#32424,#32425);
#26689=AXIS2_PLACEMENT_3D('',#48363,#32426,#32427);
#26690=AXIS2_PLACEMENT_3D('',#48367,#32430,#32431);
#26691=AXIS2_PLACEMENT_3D('',#48375,#32434,#32435);
#26692=AXIS2_PLACEMENT_3D('',#48381,#32437,#32438);
#26693=AXIS2_PLACEMENT_3D('',#48384,#32439,#32440);
#26694=AXIS2_PLACEMENT_3D('',#48388,#32443,#32444);
#26695=AXIS2_PLACEMENT_3D('',#48396,#32447,#32448);
#26696=AXIS2_PLACEMENT_3D('',#48402,#32450,#32451);
#26697=AXIS2_PLACEMENT_3D('',#48405,#32452,#32453);
#26698=AXIS2_PLACEMENT_3D('',#48409,#32456,#32457);
#26699=AXIS2_PLACEMENT_3D('',#48417,#32460,#32461);
#26700=AXIS2_PLACEMENT_3D('',#48423,#32463,#32464);
#26701=AXIS2_PLACEMENT_3D('',#48426,#32465,#32466);
#26702=AXIS2_PLACEMENT_3D('',#48430,#32469,#32470);
#26703=AXIS2_PLACEMENT_3D('',#48438,#32473,#32474);
#26704=AXIS2_PLACEMENT_3D('',#48444,#32476,#32477);
#26705=AXIS2_PLACEMENT_3D('',#48447,#32478,#32479);
#26706=AXIS2_PLACEMENT_3D('',#48451,#32482,#32483);
#26707=AXIS2_PLACEMENT_3D('',#48459,#32486,#32487);
#26708=AXIS2_PLACEMENT_3D('',#48465,#32489,#32490);
#26709=AXIS2_PLACEMENT_3D('',#48468,#32491,#32492);
#26710=AXIS2_PLACEMENT_3D('',#48472,#32495,#32496);
#26711=AXIS2_PLACEMENT_3D('',#48480,#32499,#32500);
#26712=AXIS2_PLACEMENT_3D('',#48486,#32502,#32503);
#26713=AXIS2_PLACEMENT_3D('',#48489,#32504,#32505);
#26714=AXIS2_PLACEMENT_3D('',#48493,#32508,#32509);
#26715=AXIS2_PLACEMENT_3D('',#48501,#32512,#32513);
#26716=AXIS2_PLACEMENT_3D('',#48507,#32515,#32516);
#26717=AXIS2_PLACEMENT_3D('',#48510,#32517,#32518);
#26718=AXIS2_PLACEMENT_3D('',#48514,#32521,#32522);
#26719=AXIS2_PLACEMENT_3D('',#48522,#32525,#32526);
#26720=AXIS2_PLACEMENT_3D('',#48528,#32528,#32529);
#26721=AXIS2_PLACEMENT_3D('',#48531,#32530,#32531);
#26722=AXIS2_PLACEMENT_3D('',#48535,#32534,#32535);
#26723=AXIS2_PLACEMENT_3D('',#48543,#32538,#32539);
#26724=AXIS2_PLACEMENT_3D('',#48549,#32541,#32542);
#26725=AXIS2_PLACEMENT_3D('',#48550,#32543,#32544);
#26726=AXIS2_PLACEMENT_3D('',#48551,#32545,#32546);
#26727=AXIS2_PLACEMENT_3D('',#48552,#32547,#32548);
#26728=AXIS2_PLACEMENT_3D('',#48553,#32549,#32550);
#26729=AXIS2_PLACEMENT_3D('',#48554,#32551,#32552);
#26730=AXIS2_PLACEMENT_3D('',#48555,#32553,#32554);
#26731=AXIS2_PLACEMENT_3D('',#48556,#32555,#32556);
#26732=AXIS2_PLACEMENT_3D('',#48557,#32557,#32558);
#26733=AXIS2_PLACEMENT_3D('',#48558,#32559,#32560);
#26734=AXIS2_PLACEMENT_3D('',#48559,#32561,#32562);
#26735=AXIS2_PLACEMENT_3D('',#48560,#32563,#32564);
#26736=AXIS2_PLACEMENT_3D('',#48561,#32565,#32566);
#26737=AXIS2_PLACEMENT_3D('',#48562,#32567,#32568);
#26738=AXIS2_PLACEMENT_3D('',#48563,#32569,#32570);
#26739=AXIS2_PLACEMENT_3D('',#48564,#32571,#32572);
#26740=AXIS2_PLACEMENT_3D('',#48565,#32573,#32574);
#26741=AXIS2_PLACEMENT_3D('',#48566,#32575,#32576);
#26742=AXIS2_PLACEMENT_3D('',#48569,#32578,#32579);
#26743=AXIS2_PLACEMENT_3D('',#48570,#32580,#32581);
#26744=AXIS2_PLACEMENT_3D('',#48571,#32582,#32583);
#26745=AXIS2_PLACEMENT_3D('',#48572,#32584,#32585);
#26746=AXIS2_PLACEMENT_3D('',#48573,#32586,#32587);
#26747=AXIS2_PLACEMENT_3D('',#48574,#32588,#32589);
#26748=AXIS2_PLACEMENT_3D('',#48575,#32590,#32591);
#26749=AXIS2_PLACEMENT_3D('',#48576,#32592,#32593);
#26750=AXIS2_PLACEMENT_3D('',#48577,#32594,#32595);
#26751=AXIS2_PLACEMENT_3D('',#48578,#32596,#32597);
#26752=AXIS2_PLACEMENT_3D('',#48579,#32598,#32599);
#26753=AXIS2_PLACEMENT_3D('',#48580,#32600,#32601);
#26754=AXIS2_PLACEMENT_3D('',#48581,#32602,#32603);
#26755=AXIS2_PLACEMENT_3D('',#48582,#32604,#32605);
#26756=AXIS2_PLACEMENT_3D('',#48583,#32606,#32607);
#26757=AXIS2_PLACEMENT_3D('',#48584,#32608,#32609);
#26758=AXIS2_PLACEMENT_3D('',#48585,#32610,#32611);
#26759=AXIS2_PLACEMENT_3D('',#48586,#32612,#32613);
#26760=AXIS2_PLACEMENT_3D('',#48588,#32614,#32615);
#26761=AXIS2_PLACEMENT_3D('',#48592,#32617,#32618);
#26762=AXIS2_PLACEMENT_3D('',#48595,#32620,#32621);
#26763=AXIS2_PLACEMENT_3D('',#48596,#32622,#32623);
#26764=AXIS2_PLACEMENT_3D('',#48604,#32626,#32627);
#26765=AXIS2_PLACEMENT_3D('',#48609,#32629,#32630);
#26766=AXIS2_PLACEMENT_3D('',#48610,#32631,#32632);
#26767=AXIS2_PLACEMENT_3D('',#48612,#32633,#32634);
#26768=AXIS2_PLACEMENT_3D('',#48614,#32636,#32637);
#26769=AXIS2_PLACEMENT_3D('',#48618,#32639,#32640);
#26770=AXIS2_PLACEMENT_3D('',#48619,#32641,#32642);
#26771=AXIS2_PLACEMENT_3D('',#48628,#32647,#32648);
#26772=AXIS2_PLACEMENT_3D('',#48634,#32652,#32653);
#26773=AXIS2_PLACEMENT_3D('',#48640,#32657,#32658);
#26774=AXIS2_PLACEMENT_3D('',#48646,#32662,#32663);
#26775=AXIS2_PLACEMENT_3D('',#48652,#32667,#32668);
#26776=AXIS2_PLACEMENT_3D('',#48655,#32671,#32672);
#26777=AXIS2_PLACEMENT_3D('',#48656,#32673,#32674);
#26778=AXIS2_PLACEMENT_3D('',#48658,#32675,#32676);
#26779=AXIS2_PLACEMENT_3D('',#48659,#32677,#32678);
#26780=AXIS2_PLACEMENT_3D('',#48661,#32680,#32681);
#26781=AXIS2_PLACEMENT_3D('',#48662,#32682,#32683);
#26782=AXIS2_PLACEMENT_3D('',#48663,#32684,#32685);
#26783=AXIS2_PLACEMENT_3D('',#48665,#32686,#32687);
#26784=AXIS2_PLACEMENT_3D('',#48667,#32689,#32690);
#26785=AXIS2_PLACEMENT_3D('',#48668,#32691,#32692);
#31918=DIRECTION('axis',(0.,0.,1.));
#31919=DIRECTION('refdir',(1.,0.,0.));
#31920=DIRECTION('center_axis',(0.,0.,1.));
#31921=DIRECTION('ref_axis',(1.,0.,0.));
#31922=DIRECTION('',(0.,0.,-1.));
#31923=DIRECTION('center_axis',(0.,0.,-1.));
#31924=DIRECTION('ref_axis',(1.,0.,0.));
#31925=DIRECTION('',(0.,0.,-1.));
#31926=DIRECTION('center_axis',(0.,0.,1.));
#31927=DIRECTION('ref_axis',(1.,0.,0.));
#31928=DIRECTION('center_axis',(0.,0.,-1.));
#31929=DIRECTION('ref_axis',(1.,0.,0.));
#31930=DIRECTION('center_axis',(0.,0.,1.));
#31931=DIRECTION('ref_axis',(1.,0.,0.));
#31932=DIRECTION('',(0.,0.,-1.));
#31933=DIRECTION('center_axis',(0.,0.,1.));
#31934=DIRECTION('ref_axis',(1.,0.,0.));
#31935=DIRECTION('',(0.,0.,-1.));
#31936=DIRECTION('center_axis',(0.,0.,1.));
#31937=DIRECTION('ref_axis',(1.,0.,0.));
#31938=DIRECTION('',(0.,0.,-1.));
#31939=DIRECTION('center_axis',(0.,0.,1.));
#31940=DIRECTION('ref_axis',(1.,0.,0.));
#31941=DIRECTION('',(0.,0.,-1.));
#31942=DIRECTION('center_axis',(0.,0.,1.));
#31943=DIRECTION('ref_axis',(1.,0.,0.));
#31944=DIRECTION('',(0.,0.,-1.));
#31945=DIRECTION('center_axis',(0.,0.,1.));
#31946=DIRECTION('ref_axis',(1.,0.,0.));
#31947=DIRECTION('',(0.,0.,-1.));
#31948=DIRECTION('center_axis',(0.,0.,1.));
#31949=DIRECTION('ref_axis',(1.,0.,0.));
#31950=DIRECTION('',(0.,0.,-1.));
#31951=DIRECTION('center_axis',(0.,0.,1.));
#31952=DIRECTION('ref_axis',(1.,0.,0.));
#31953=DIRECTION('',(0.,0.,-1.));
#31954=DIRECTION('center_axis',(0.,0.,1.));
#31955=DIRECTION('ref_axis',(1.,0.,0.));
#31956=DIRECTION('',(0.,0.,-1.));
#31957=DIRECTION('center_axis',(0.,0.,1.));
#31958=DIRECTION('ref_axis',(1.,0.,0.));
#31959=DIRECTION('',(0.,0.,-1.));
#31960=DIRECTION('center_axis',(0.,0.,1.));
#31961=DIRECTION('ref_axis',(1.,0.,0.));
#31962=DIRECTION('',(0.,0.,-1.));
#31963=DIRECTION('center_axis',(0.,0.,1.));
#31964=DIRECTION('ref_axis',(1.,0.,0.));
#31965=DIRECTION('',(0.,0.,-1.));
#31966=DIRECTION('center_axis',(0.,0.,1.));
#31967=DIRECTION('ref_axis',(1.,0.,0.));
#31968=DIRECTION('',(0.,0.,-1.));
#31969=DIRECTION('center_axis',(0.,0.,1.));
#31970=DIRECTION('ref_axis',(1.,0.,0.));
#31971=DIRECTION('',(0.,0.,-1.));
#31972=DIRECTION('center_axis',(0.,0.,1.));
#31973=DIRECTION('ref_axis',(1.,0.,0.));
#31974=DIRECTION('',(0.,0.,-1.));
#31975=DIRECTION('center_axis',(0.,0.,1.));
#31976=DIRECTION('ref_axis',(1.,0.,0.));
#31977=DIRECTION('',(0.,0.,-1.));
#31978=DIRECTION('center_axis',(0.,0.,1.));
#31979=DIRECTION('ref_axis',(1.,0.,0.));
#31980=DIRECTION('',(0.,0.,-1.));
#31981=DIRECTION('center_axis',(0.,0.,1.));
#31982=DIRECTION('ref_axis',(1.,0.,0.));
#31983=DIRECTION('',(0.,0.,-1.));
#31984=DIRECTION('center_axis',(0.,0.,1.));
#31985=DIRECTION('ref_axis',(1.,0.,0.));
#31986=DIRECTION('',(0.,0.,-1.));
#31987=DIRECTION('center_axis',(0.,0.,1.));
#31988=DIRECTION('ref_axis',(1.,0.,0.));
#31989=DIRECTION('',(0.,0.,-1.));
#31990=DIRECTION('center_axis',(0.,0.,1.));
#31991=DIRECTION('ref_axis',(1.,0.,0.));
#31992=DIRECTION('',(0.,0.,-1.));
#31993=DIRECTION('center_axis',(0.,0.,1.));
#31994=DIRECTION('ref_axis',(1.,0.,0.));
#31995=DIRECTION('',(0.,0.,-1.));
#31996=DIRECTION('center_axis',(0.,0.,1.));
#31997=DIRECTION('ref_axis',(-0.0038548301263327,-0.999992570114747,0.));
#31998=DIRECTION('',(0.,0.,1.));
#31999=DIRECTION('center_axis',(0.,0.,1.));
#32000=DIRECTION('ref_axis',(1.,-8.97481250249747E-15,0.));
#32001=DIRECTION('center_axis',(0.,0.,1.));
#32002=DIRECTION('ref_axis',(1.,-8.97481250249747E-15,0.));
#32003=DIRECTION('',(0.,0.,1.));
#32004=DIRECTION('center_axis',(0.,0.,1.));
#32005=DIRECTION('ref_axis',(1.,-8.97481250249747E-15,0.));
#32006=DIRECTION('',(0.,0.,1.));
#32007=DIRECTION('center_axis',(0.,0.,1.));
#32008=DIRECTION('ref_axis',(1.,-8.97481250249747E-15,0.));
#32009=DIRECTION('',(0.,0.,1.));
#32010=DIRECTION('center_axis',(0.,0.,1.));
#32011=DIRECTION('ref_axis',(1.,-8.97481250249747E-15,0.));
#32012=DIRECTION('',(0.,0.,1.));
#32013=DIRECTION('center_axis',(0.,0.,1.));
#32014=DIRECTION('ref_axis',(1.,-8.97481250249747E-15,0.));
#32015=DIRECTION('',(0.,0.,1.));
#32016=DIRECTION('center_axis',(0.,0.,1.));
#32017=DIRECTION('ref_axis',(1.,-8.97481250249747E-15,0.));
#32018=DIRECTION('',(0.,0.,1.));
#32019=DIRECTION('center_axis',(0.,0.,1.));
#32020=DIRECTION('ref_axis',(1.,-8.97481250249747E-15,0.));
#32021=DIRECTION('',(0.,0.,1.));
#32022=DIRECTION('center_axis',(0.,0.,1.));
#32023=DIRECTION('ref_axis',(1.,-8.97481250249747E-15,0.));
#32024=DIRECTION('',(0.,0.,1.));
#32025=DIRECTION('center_axis',(0.,0.,1.));
#32026=DIRECTION('ref_axis',(1.,-8.97481250249747E-15,0.));
#32027=DIRECTION('',(0.,0.,1.));
#32028=DIRECTION('center_axis',(0.,0.,1.));
#32029=DIRECTION('ref_axis',(1.,-8.97481250249747E-15,0.));
#32030=DIRECTION('',(0.,0.,1.));
#32031=DIRECTION('center_axis',(0.,0.,1.));
#32032=DIRECTION('ref_axis',(1.,-8.97481250249747E-15,0.));
#32033=DIRECTION('',(0.,0.,1.));
#32034=DIRECTION('center_axis',(0.,0.,1.));
#32035=DIRECTION('ref_axis',(1.,-8.97481250249747E-15,0.));
#32036=DIRECTION('',(0.,0.,1.));
#32037=DIRECTION('center_axis',(0.,0.,1.));
#32038=DIRECTION('ref_axis',(1.,-8.97481250249747E-15,0.));
#32039=DIRECTION('',(0.,0.,1.));
#32040=DIRECTION('center_axis',(0.,0.,1.));
#32041=DIRECTION('ref_axis',(1.,-8.97481250249747E-15,0.));
#32042=DIRECTION('',(0.,0.,1.));
#32043=DIRECTION('center_axis',(0.,0.,1.));
#32044=DIRECTION('ref_axis',(1.,-8.97481250249747E-15,0.));
#32045=DIRECTION('',(0.,0.,1.));
#32046=DIRECTION('center_axis',(0.,0.,1.));
#32047=DIRECTION('ref_axis',(1.,-8.97481250249747E-15,0.));
#32048=DIRECTION('',(0.,0.,1.));
#32049=DIRECTION('center_axis',(0.,0.,1.));
#32050=DIRECTION('ref_axis',(1.,-8.97481250249747E-15,0.));
#32051=DIRECTION('',(0.,0.,1.));
#32052=DIRECTION('center_axis',(0.,0.,1.));
#32053=DIRECTION('ref_axis',(1.,-8.97481250249747E-15,0.));
#32054=DIRECTION('',(0.,0.,1.));
#32055=DIRECTION('center_axis',(0.,0.,1.));
#32056=DIRECTION('ref_axis',(1.,-8.97481250249747E-15,0.));
#32057=DIRECTION('',(0.,0.,1.));
#32058=DIRECTION('center_axis',(0.,0.,1.));
#32059=DIRECTION('ref_axis',(1.,-8.97481250249747E-15,0.));
#32060=DIRECTION('',(0.,0.,1.));
#32061=DIRECTION('center_axis',(0.,0.,1.));
#32062=DIRECTION('ref_axis',(1.,-8.97481250249747E-15,0.));
#32063=DIRECTION('',(0.,0.,1.));
#32064=DIRECTION('center_axis',(0.,0.,1.));
#32065=DIRECTION('ref_axis',(1.,-8.97481250249747E-15,0.));
#32066=DIRECTION('',(0.,0.,1.));
#32067=DIRECTION('center_axis',(0.,0.,1.));
#32068=DIRECTION('ref_axis',(1.,-8.97481250249747E-15,0.));
#32069=DIRECTION('',(0.,0.,1.));
#32070=DIRECTION('center_axis',(0.,0.,-1.));
#32071=DIRECTION('ref_axis',(1.,-8.97481250249747E-15,0.));
#32072=DIRECTION('center_axis',(0.,0.,1.));
#32073=DIRECTION('ref_axis',(1.,0.,0.));
#32074=DIRECTION('center_axis',(0.,0.,1.));
#32075=DIRECTION('ref_axis',(1.,0.,0.));
#32076=DIRECTION('center_axis',(0.,0.,1.));
#32077=DIRECTION('ref_axis',(1.,0.,0.));
#32078=DIRECTION('center_axis',(0.,0.,1.));
#32079=DIRECTION('ref_axis',(1.,0.,0.));
#32080=DIRECTION('center_axis',(0.,0.,-1.));
#32081=DIRECTION('ref_axis',(1.,-8.97481250249747E-15,0.));
#32082=DIRECTION('center_axis',(0.,0.,1.));
#32083=DIRECTION('ref_axis',(-0.952277678384196,0.305233063823706,0.));
#32084=DIRECTION('center_axis',(0.,0.,1.));
#32085=DIRECTION('ref_axis',(0.984807753012208,-0.17364817766693,0.));
#32086=DIRECTION('center_axis',(0.,0.,-1.));
#32087=DIRECTION('ref_axis',(1.,0.,0.));
#32088=DIRECTION('',(-0.996089805327885,-0.0883464754353932,0.));
#32089=DIRECTION('',(0.905801965515954,-0.423701309022563,0.));
#32090=DIRECTION('center_axis',(-0.423701309022563,-0.905801965515954,0.));
#32091=DIRECTION('ref_axis',(0.905801965515954,-0.423701309022563,0.));
#32092=DIRECTION('',(0.,0.,1.));
#32093=DIRECTION('',(0.,0.,1.));
#32094=DIRECTION('center_axis',(-0.0883464754353932,0.996089805327885,0.));
#32095=DIRECTION('ref_axis',(-0.996089805327885,-0.0883464754353932,0.));
#32096=DIRECTION('',(0.,0.,-1.));
#32097=DIRECTION('center_axis',(0.,0.,1.));
#32098=DIRECTION('ref_axis',(0.939692620785908,-0.342020143325669,0.));
#32099=DIRECTION('center_axis',(0.,0.,-1.));
#32100=DIRECTION('ref_axis',(1.,0.,0.));
#32101=DIRECTION('',(-0.996298167445974,0.0859648855277176,0.));
#32102=DIRECTION('',(0.818465838146947,-0.574555194725812,0.));
#32103=DIRECTION('center_axis',(-0.574555194725812,-0.818465838146947,0.));
#32104=DIRECTION('ref_axis',(0.818465838146947,-0.574555194725812,0.));
#32105=DIRECTION('',(0.,0.,1.));
#32106=DIRECTION('',(0.,0.,1.));
#32107=DIRECTION('center_axis',(0.0859648855277176,0.996298167445974,0.));
#32108=DIRECTION('ref_axis',(-0.996298167445974,0.0859648855277176,0.));
#32109=DIRECTION('',(0.,0.,-1.));
#32110=DIRECTION('center_axis',(0.,0.,1.));
#32111=DIRECTION('ref_axis',(0.866025403784438,-0.5,0.));
#32112=DIRECTION('center_axis',(0.,0.,-1.));
#32113=DIRECTION('ref_axis',(1.,0.,0.));
#32114=DIRECTION('',(-0.966234513897416,0.257664246944399,0.));
#32115=DIRECTION('',(0.706261040449543,-0.707951511576272,0.));
#32116=DIRECTION('center_axis',(-0.707951511576272,-0.706261040449543,0.));
#32117=DIRECTION('ref_axis',(0.706261040449543,-0.707951511576272,0.));
#32118=DIRECTION('',(0.,0.,1.));
#32119=DIRECTION('',(0.,0.,1.));
#32120=DIRECTION('center_axis',(0.257664246944399,0.966234513897416,0.));
#32121=DIRECTION('ref_axis',(-0.966234513897416,0.257664246944399,0.));
#32122=DIRECTION('',(0.,0.,-1.));
#32123=DIRECTION('center_axis',(0.,0.,1.));
#32124=DIRECTION('ref_axis',(0.766044443118978,-0.64278760968654,0.));
#32125=DIRECTION('center_axis',(0.,0.,-1.));
#32126=DIRECTION('ref_axis',(1.,0.,0.));
#32127=DIRECTION('',(-0.906812313582341,0.421534610602074,0.));
#32128=DIRECTION('',(0.572596858423411,-0.819837079988238,0.));
#32129=DIRECTION('center_axis',(-0.819837079988238,-0.572596858423411,0.));
#32130=DIRECTION('ref_axis',(0.572596858423411,-0.819837079988238,0.));
#32131=DIRECTION('',(0.,0.,1.));
#32132=DIRECTION('',(0.,0.,1.));
#32133=DIRECTION('center_axis',(0.421534610602074,0.906812313582341,0.));
#32134=DIRECTION('ref_axis',(-0.906812313582341,0.421534610602074,0.));
#32135=DIRECTION('',(0.,0.,-1.));
#32136=DIRECTION('center_axis',(0.,0.,1.));
#32137=DIRECTION('ref_axis',(0.642787609686539,-0.766044443118978,0.));
#32138=DIRECTION('center_axis',(0.,0.,-1.));
#32139=DIRECTION('ref_axis',(1.,0.,0.));
#32140=DIRECTION('',(-0.819837079988238,0.572596858423411,0.));
#32141=DIRECTION('',(0.421534610602074,-0.906812313582341,0.));
#32142=DIRECTION('center_axis',(-0.906812313582341,-0.421534610602074,0.));
#32143=DIRECTION('ref_axis',(0.421534610602074,-0.906812313582341,0.));
#32144=DIRECTION('',(0.,0.,1.));
#32145=DIRECTION('',(0.,0.,1.));
#32146=DIRECTION('center_axis',(0.572596858423411,0.819837079988238,0.));
#32147=DIRECTION('ref_axis',(-0.819837079988238,0.572596858423411,0.));
#32148=DIRECTION('',(0.,0.,-1.));
#32149=DIRECTION('center_axis',(0.,0.,1.));
#32150=DIRECTION('ref_axis',(0.5,-0.866025403784438,0.));
#32151=DIRECTION('center_axis',(0.,0.,-1.));
#32152=DIRECTION('ref_axis',(1.,0.,0.));
#32153=DIRECTION('',(-0.707951511576272,0.706261040449544,0.));
#32154=DIRECTION('',(0.257664246944398,-0.966234513897416,0.));
#32155=DIRECTION('center_axis',(-0.966234513897416,-0.257664246944398,0.));
#32156=DIRECTION('ref_axis',(0.257664246944398,-0.966234513897416,0.));
#32157=DIRECTION('',(0.,0.,1.));
#32158=DIRECTION('',(0.,0.,1.));
#32159=DIRECTION('center_axis',(0.706261040449544,0.707951511576272,0.));
#32160=DIRECTION('ref_axis',(-0.707951511576272,0.706261040449544,0.));
#32161=DIRECTION('',(0.,0.,-1.));
#32162=DIRECTION('center_axis',(0.,0.,1.));
#32163=DIRECTION('ref_axis',(0.342020143325668,-0.939692620785909,0.));
#32164=DIRECTION('center_axis',(0.,0.,-1.));
#32165=DIRECTION('ref_axis',(1.,0.,0.));
#32166=DIRECTION('',(-0.57455519472581,0.818465838146948,0.));
#32167=DIRECTION('',(0.0859648855277162,-0.996298167445974,0.));
#32168=DIRECTION('center_axis',(-0.996298167445974,-0.0859648855277162,
0.));
#32169=DIRECTION('ref_axis',(0.0859648855277162,-0.996298167445974,0.));
#32170=DIRECTION('',(0.,0.,1.));
#32171=DIRECTION('',(0.,0.,1.));
#32172=DIRECTION('center_axis',(0.818465838146948,0.57455519472581,0.));
#32173=DIRECTION('ref_axis',(-0.57455519472581,0.818465838146948,0.));
#32174=DIRECTION('',(0.,0.,-1.));
#32175=DIRECTION('center_axis',(0.,0.,1.));
#32176=DIRECTION('ref_axis',(0.17364817766693,-0.984807753012208,0.));
#32177=DIRECTION('center_axis',(0.,0.,-1.));
#32178=DIRECTION('ref_axis',(1.,0.,0.));
#32179=DIRECTION('',(-0.423701309022563,0.905801965515955,0.));
#32180=DIRECTION('',(-0.0883464754353936,-0.996089805327885,0.));
#32181=DIRECTION('center_axis',(-0.996089805327885,0.0883464754353937,0.));
#32182=DIRECTION('ref_axis',(-0.0883464754353937,-0.996089805327885,0.));
#32183=DIRECTION('',(0.,0.,1.));
#32184=DIRECTION('',(0.,0.,1.));
#32185=DIRECTION('center_axis',(0.905801965515955,0.423701309022563,0.));
#32186=DIRECTION('ref_axis',(-0.423701309022563,0.905801965515955,0.));
#32187=DIRECTION('',(0.,0.,-1.));
#32188=DIRECTION('center_axis',(0.,0.,1.));
#32189=DIRECTION('ref_axis',(-1.94289029309402E-16,-1.,0.));
#32190=DIRECTION('center_axis',(0.,0.,-1.));
#32191=DIRECTION('ref_axis',(1.,0.,0.));
#32192=DIRECTION('',(-0.259973473447872,0.96561575852067,0.));
#32193=DIRECTION('',(-0.259973473447873,-0.96561575852067,0.));
#32194=DIRECTION('center_axis',(-0.96561575852067,0.259973473447873,0.));
#32195=DIRECTION('ref_axis',(-0.259973473447873,-0.96561575852067,0.));
#32196=DIRECTION('',(0.,0.,1.));
#32197=DIRECTION('',(0.,0.,1.));
#32198=DIRECTION('center_axis',(0.96561575852067,0.259973473447872,0.));
#32199=DIRECTION('ref_axis',(-0.259973473447872,0.96561575852067,0.));
#32200=DIRECTION('',(0.,0.,-1.));
#32201=DIRECTION('center_axis',(0.,0.,1.));
#32202=DIRECTION('ref_axis',(-0.17364817766693,-0.984807753012208,0.));
#32203=DIRECTION('center_axis',(0.,0.,-1.));
#32204=DIRECTION('ref_axis',(1.,0.,0.));
#32205=DIRECTION('',(-0.0883464754353933,0.996089805327885,0.));
#32206=DIRECTION('',(-0.423701309022563,-0.905801965515955,0.));
#32207=DIRECTION('center_axis',(-0.905801965515955,0.423701309022563,0.));
#32208=DIRECTION('ref_axis',(-0.423701309022563,-0.905801965515955,0.));
#32209=DIRECTION('',(0.,0.,1.));
#32210=DIRECTION('',(0.,0.,1.));
#32211=DIRECTION('center_axis',(0.996089805327885,0.0883464754353932,0.));
#32212=DIRECTION('ref_axis',(-0.0883464754353932,0.996089805327885,0.));
#32213=DIRECTION('',(0.,0.,-1.));
#32214=DIRECTION('center_axis',(0.,0.,1.));
#32215=DIRECTION('ref_axis',(-0.342020143325669,-0.939692620785908,0.));
#32216=DIRECTION('center_axis',(0.,0.,-1.));
#32217=DIRECTION('ref_axis',(1.,0.,0.));
#32218=DIRECTION('',(0.0859648855277175,0.996298167445974,0.));
#32219=DIRECTION('',(-0.574555194725811,-0.818465838146947,0.));
#32220=DIRECTION('center_axis',(-0.818465838146947,0.574555194725811,0.));
#32221=DIRECTION('ref_axis',(-0.574555194725811,-0.818465838146947,0.));
#32222=DIRECTION('',(0.,0.,1.));
#32223=DIRECTION('',(0.,0.,1.));
#32224=DIRECTION('center_axis',(0.996298167445974,-0.0859648855277175,0.));
#32225=DIRECTION('ref_axis',(0.0859648855277175,0.996298167445974,0.));
#32226=DIRECTION('',(0.,0.,-1.));
#32227=DIRECTION('center_axis',(0.,0.,1.));
#32228=DIRECTION('ref_axis',(-0.5,-0.866025403784438,0.));
#32229=DIRECTION('center_axis',(0.,0.,-1.));
#32230=DIRECTION('ref_axis',(1.,0.,0.));
#32231=DIRECTION('',(0.257664246944399,0.966234513897416,0.));
#32232=DIRECTION('',(-0.707951511576272,-0.706261040449543,0.));
#32233=DIRECTION('center_axis',(-0.706261040449543,0.707951511576272,0.));
#32234=DIRECTION('ref_axis',(-0.707951511576272,-0.706261040449543,0.));
#32235=DIRECTION('',(0.,0.,1.));
#32236=DIRECTION('',(0.,0.,1.));
#32237=DIRECTION('center_axis',(0.966234513897416,-0.257664246944399,0.));
#32238=DIRECTION('ref_axis',(0.257664246944399,0.966234513897416,0.));
#32239=DIRECTION('',(0.,0.,-1.));
#32240=DIRECTION('center_axis',(0.,0.,1.));
#32241=DIRECTION('ref_axis',(-0.642787609686539,-0.766044443118978,0.));
#32242=DIRECTION('center_axis',(0.,0.,-1.));
#32243=DIRECTION('ref_axis',(1.,0.,0.));
#32244=DIRECTION('',(0.421534610602074,0.906812313582341,0.));
#32245=DIRECTION('',(-0.819837079988238,-0.572596858423411,0.));
#32246=DIRECTION('center_axis',(-0.572596858423411,0.819837079988238,0.));
#32247=DIRECTION('ref_axis',(-0.819837079988238,-0.572596858423411,0.));
#32248=DIRECTION('',(0.,0.,1.));
#32249=DIRECTION('',(0.,0.,1.));
#32250=DIRECTION('center_axis',(0.906812313582341,-0.421534610602074,0.));
#32251=DIRECTION('ref_axis',(0.421534610602074,0.906812313582341,0.));
#32252=DIRECTION('',(0.,0.,-1.));
#32253=DIRECTION('center_axis',(0.,0.,1.));
#32254=DIRECTION('ref_axis',(-0.766044443118978,-0.642787609686539,0.));
#32255=DIRECTION('center_axis',(0.,0.,-1.));
#32256=DIRECTION('ref_axis',(1.,0.,0.));
#32257=DIRECTION('',(0.572596858423411,0.819837079988238,0.));
#32258=DIRECTION('',(-0.906812313582341,-0.421534610602074,0.));
#32259=DIRECTION('center_axis',(-0.421534610602074,0.906812313582341,0.));
#32260=DIRECTION('ref_axis',(-0.906812313582341,-0.421534610602074,0.));
#32261=DIRECTION('',(0.,0.,1.));
#32262=DIRECTION('',(0.,0.,1.));
#32263=DIRECTION('center_axis',(0.819837079988238,-0.572596858423411,0.));
#32264=DIRECTION('ref_axis',(0.572596858423411,0.819837079988238,0.));
#32265=DIRECTION('',(0.,0.,-1.));
#32266=DIRECTION('center_axis',(0.,0.,1.));
#32267=DIRECTION('ref_axis',(-0.866025403784439,-0.5,0.));
#32268=DIRECTION('center_axis',(0.,0.,-1.));
#32269=DIRECTION('ref_axis',(1.,0.,0.));
#32270=DIRECTION('',(0.706261040449544,0.707951511576271,0.));
#32271=DIRECTION('',(-0.966234513897416,-0.257664246944398,0.));
#32272=DIRECTION('center_axis',(-0.257664246944398,0.966234513897416,0.));
#32273=DIRECTION('ref_axis',(-0.966234513897416,-0.257664246944398,0.));
#32274=DIRECTION('',(0.,0.,1.));
#32275=DIRECTION('',(0.,0.,1.));
#32276=DIRECTION('center_axis',(0.707951511576271,-0.706261040449544,0.));
#32277=DIRECTION('ref_axis',(0.706261040449544,0.707951511576271,0.));
#32278=DIRECTION('',(0.,0.,-1.));
#32279=DIRECTION('center_axis',(0.,0.,1.));
#32280=DIRECTION('ref_axis',(-0.939692620785909,-0.342020143325669,0.));
#32281=DIRECTION('center_axis',(0.,0.,-1.));
#32282=DIRECTION('ref_axis',(1.,0.,0.));
#32283=DIRECTION('',(0.818465838146948,0.574555194725811,0.));
#32284=DIRECTION('',(-0.996298167445974,-0.0859648855277167,0.));
#32285=DIRECTION('center_axis',(-0.0859648855277167,0.996298167445974,0.));
#32286=DIRECTION('ref_axis',(-0.996298167445974,-0.0859648855277167,0.));
#32287=DIRECTION('',(0.,0.,1.));
#32288=DIRECTION('',(0.,0.,1.));
#32289=DIRECTION('center_axis',(0.574555194725811,-0.818465838146948,0.));
#32290=DIRECTION('ref_axis',(0.818465838146948,0.574555194725811,0.));
#32291=DIRECTION('',(0.,0.,-1.));
#32292=DIRECTION('center_axis',(0.,0.,1.));
#32293=DIRECTION('ref_axis',(-0.984807753012208,-0.17364817766693,0.));
#32294=DIRECTION('center_axis',(0.,0.,-1.));
#32295=DIRECTION('ref_axis',(1.,0.,0.));
#32296=DIRECTION('',(0.905801965515955,0.423701309022563,0.));
#32297=DIRECTION('',(-0.996089805327885,0.0883464754353936,0.));
#32298=DIRECTION('center_axis',(0.0883464754353936,0.996089805327885,0.));
#32299=DIRECTION('ref_axis',(-0.996089805327885,0.0883464754353936,0.));
#32300=DIRECTION('',(0.,0.,1.));
#32301=DIRECTION('',(0.,0.,1.));
#32302=DIRECTION('center_axis',(0.423701309022563,-0.905801965515955,0.));
#32303=DIRECTION('ref_axis',(0.905801965515955,0.423701309022563,0.));
#32304=DIRECTION('',(0.,0.,-1.));
#32305=DIRECTION('center_axis',(0.,0.,1.));
#32306=DIRECTION('ref_axis',(-1.,1.11022302462516E-16,0.));
#32307=DIRECTION('center_axis',(0.,0.,-1.));
#32308=DIRECTION('ref_axis',(1.,0.,0.));
#32309=DIRECTION('',(0.96561575852067,0.259973473447872,0.));
#32310=DIRECTION('',(-0.96561575852067,0.259973473447873,0.));
#32311=DIRECTION('center_axis',(0.,0.,-1.));
#32312=DIRECTION('ref_axis',(1.,0.,0.));
#32313=DIRECTION('center_axis',(0.259973473447873,0.96561575852067,0.));
#32314=DIRECTION('ref_axis',(-0.96561575852067,0.259973473447873,0.));
#32315=DIRECTION('',(0.,0.,1.));
#32316=DIRECTION('',(0.,0.,1.));
#32317=DIRECTION('center_axis',(0.259973473447872,-0.96561575852067,0.));
#32318=DIRECTION('ref_axis',(0.96561575852067,0.259973473447872,0.));
#32319=DIRECTION('',(0.,0.,-1.));
#32320=DIRECTION('center_axis',(0.,0.,1.));
#32321=DIRECTION('ref_axis',(-0.984807753012208,0.173648177666931,0.));
#32322=DIRECTION('center_axis',(0.,0.,-1.));
#32323=DIRECTION('ref_axis',(1.,0.,0.));
#32324=DIRECTION('',(0.996089805327885,0.0883464754353928,0.));
#32325=DIRECTION('',(-0.905801965515954,0.423701309022564,0.));
#32326=DIRECTION('center_axis',(0.423701309022564,0.905801965515954,0.));
#32327=DIRECTION('ref_axis',(-0.905801965515954,0.423701309022564,0.));
#32328=DIRECTION('',(0.,0.,1.));
#32329=DIRECTION('',(0.,0.,1.));
#32330=DIRECTION('center_axis',(0.0883464754353928,-0.996089805327885,0.));
#32331=DIRECTION('ref_axis',(0.996089805327885,0.0883464754353928,0.));
#32332=DIRECTION('',(0.,0.,-1.));
#32333=DIRECTION('center_axis',(0.,0.,1.));
#32334=DIRECTION('ref_axis',(-0.939692620785908,0.342020143325669,0.));
#32335=DIRECTION('center_axis',(0.,0.,-1.));
#32336=DIRECTION('ref_axis',(1.,0.,0.));
#32337=DIRECTION('',(0.996298167445974,-0.085964885527717,0.));
#32338=DIRECTION('',(-0.818465838146948,0.574555194725811,0.));
#32339=DIRECTION('center_axis',(0.574555194725811,0.818465838146948,0.));
#32340=DIRECTION('ref_axis',(-0.818465838146948,0.574555194725811,0.));
#32341=DIRECTION('',(0.,0.,1.));
#32342=DIRECTION('',(0.,0.,1.));
#32343=DIRECTION('center_axis',(-0.085964885527717,-0.996298167445974,0.));
#32344=DIRECTION('ref_axis',(0.996298167445974,-0.085964885527717,0.));
#32345=DIRECTION('',(0.,0.,-1.));
#32346=DIRECTION('center_axis',(0.,0.,1.));
#32347=DIRECTION('ref_axis',(-0.866025403784439,0.5,0.));
#32348=DIRECTION('center_axis',(0.,0.,-1.));
#32349=DIRECTION('ref_axis',(1.,0.,0.));
#32350=DIRECTION('',(0.966234513897416,-0.257664246944398,0.));
#32351=DIRECTION('',(-0.706261040449544,0.707951511576272,0.));
#32352=DIRECTION('center_axis',(0.707951511576272,0.706261040449544,0.));
#32353=DIRECTION('ref_axis',(-0.706261040449544,0.707951511576272,0.));
#32354=DIRECTION('',(0.,0.,1.));
#32355=DIRECTION('',(0.,0.,1.));
#32356=DIRECTION('center_axis',(-0.257664246944398,-0.966234513897416,0.));
#32357=DIRECTION('ref_axis',(0.966234513897416,-0.257664246944398,0.));
#32358=DIRECTION('',(0.,0.,-1.));
#32359=DIRECTION('center_axis',(0.,0.,1.));
#32360=DIRECTION('ref_axis',(-0.766044443118978,0.642787609686539,0.));
#32361=DIRECTION('center_axis',(0.,0.,-1.));
#32362=DIRECTION('ref_axis',(1.,0.,0.));
#32363=DIRECTION('',(0.906812313582341,-0.421534610602074,0.));
#32364=DIRECTION('',(-0.572596858423411,0.819837079988238,0.));
#32365=DIRECTION('center_axis',(0.819837079988238,0.572596858423411,0.));
#32366=DIRECTION('ref_axis',(-0.572596858423411,0.819837079988238,0.));
#32367=DIRECTION('',(0.,0.,1.));
#32368=DIRECTION('',(0.,0.,1.));
#32369=DIRECTION('center_axis',(-0.421534610602074,-0.906812313582341,0.));
#32370=DIRECTION('ref_axis',(0.906812313582341,-0.421534610602074,0.));
#32371=DIRECTION('',(0.,0.,-1.));
#32372=DIRECTION('center_axis',(0.,0.,1.));
#32373=DIRECTION('ref_axis',(-0.642787609686539,0.766044443118978,0.));
#32374=DIRECTION('center_axis',(0.,0.,-1.));
#32375=DIRECTION('ref_axis',(1.,0.,0.));
#32376=DIRECTION('',(0.819837079988238,-0.572596858423411,0.));
#32377=DIRECTION('',(-0.421534610602074,0.906812313582341,0.));
#32378=DIRECTION('center_axis',(0.906812313582341,0.421534610602074,0.));
#32379=DIRECTION('ref_axis',(-0.421534610602074,0.906812313582341,0.));
#32380=DIRECTION('',(0.,0.,1.));
#32381=DIRECTION('',(0.,0.,1.));
#32382=DIRECTION('center_axis',(-0.572596858423411,-0.819837079988238,0.));
#32383=DIRECTION('ref_axis',(0.819837079988238,-0.572596858423411,0.));
#32384=DIRECTION('',(0.,0.,-1.));
#32385=DIRECTION('center_axis',(0.,0.,1.));
#32386=DIRECTION('ref_axis',(-0.5,0.866025403784439,0.));
#32387=DIRECTION('center_axis',(0.,0.,-1.));
#32388=DIRECTION('ref_axis',(1.,0.,0.));
#32389=DIRECTION('',(0.707951511576272,-0.706261040449544,0.));
#32390=DIRECTION('',(-0.257664246944398,0.966234513897416,0.));
#32391=DIRECTION('center_axis',(0.966234513897416,0.257664246944398,0.));
#32392=DIRECTION('ref_axis',(-0.257664246944398,0.966234513897416,0.));
#32393=DIRECTION('',(0.,0.,1.));
#32394=DIRECTION('',(0.,0.,1.));
#32395=DIRECTION('center_axis',(-0.706261040449544,-0.707951511576272,0.));
#32396=DIRECTION('ref_axis',(0.707951511576272,-0.706261040449544,0.));
#32397=DIRECTION('',(0.,0.,-1.));
#32398=DIRECTION('center_axis',(0.,0.,1.));
#32399=DIRECTION('ref_axis',(-0.342020143325669,0.939692620785909,0.));
#32400=DIRECTION('center_axis',(0.,0.,-1.));
#32401=DIRECTION('ref_axis',(1.,0.,0.));
#32402=DIRECTION('',(0.574555194725811,-0.818465838146948,0.));
#32403=DIRECTION('',(-0.0859648855277167,0.996298167445974,0.));
#32404=DIRECTION('center_axis',(0.996298167445974,0.0859648855277167,0.));
#32405=DIRECTION('ref_axis',(-0.0859648855277167,0.996298167445974,0.));
#32406=DIRECTION('',(0.,0.,1.));
#32407=DIRECTION('',(0.,0.,1.));
#32408=DIRECTION('center_axis',(-0.818465838146948,-0.574555194725811,0.));
#32409=DIRECTION('ref_axis',(0.574555194725811,-0.818465838146948,0.));
#32410=DIRECTION('',(0.,0.,-1.));
#32411=DIRECTION('center_axis',(0.,0.,1.));
#32412=DIRECTION('ref_axis',(-0.17364817766693,0.984807753012208,0.));
#32413=DIRECTION('center_axis',(0.,0.,-1.));
#32414=DIRECTION('ref_axis',(1.,0.,0.));
#32415=DIRECTION('',(0.423701309022563,-0.905801965515955,0.));
#32416=DIRECTION('',(0.0883464754353932,0.996089805327885,0.));
#32417=DIRECTION('center_axis',(0.996089805327885,-0.0883464754353932,0.));
#32418=DIRECTION('ref_axis',(0.0883464754353932,0.996089805327885,0.));
#32419=DIRECTION('',(0.,0.,1.));
#32420=DIRECTION('',(0.,0.,1.));
#32421=DIRECTION('center_axis',(-0.905801965515955,-0.423701309022563,0.));
#32422=DIRECTION('ref_axis',(0.423701309022563,-0.905801965515955,0.));
#32423=DIRECTION('',(0.,0.,-1.));
#32424=DIRECTION('center_axis',(0.,0.,1.));
#32425=DIRECTION('ref_axis',(5.55111512312578E-17,1.,0.));
#32426=DIRECTION('center_axis',(0.,0.,-1.));
#32427=DIRECTION('ref_axis',(1.,0.,0.));
#32428=DIRECTION('',(0.259973473447872,-0.96561575852067,0.));
#32429=DIRECTION('',(0.259973473447872,0.96561575852067,0.));
#32430=DIRECTION('center_axis',(0.96561575852067,-0.259973473447873,0.));
#32431=DIRECTION('ref_axis',(0.259973473447873,0.96561575852067,0.));
#32432=DIRECTION('',(0.,0.,1.));
#32433=DIRECTION('',(0.,0.,1.));
#32434=DIRECTION('center_axis',(-0.96561575852067,-0.259973473447872,0.));
#32435=DIRECTION('ref_axis',(0.259973473447872,-0.96561575852067,0.));
#32436=DIRECTION('',(0.,0.,-1.));
#32437=DIRECTION('center_axis',(0.,0.,1.));
#32438=DIRECTION('ref_axis',(0.17364817766693,0.984807753012208,0.));
#32439=DIRECTION('center_axis',(0.,0.,-1.));
#32440=DIRECTION('ref_axis',(1.,0.,0.));
#32441=DIRECTION('',(0.0883464754353931,-0.996089805327885,0.));
#32442=DIRECTION('',(0.423701309022563,0.905801965515954,0.));
#32443=DIRECTION('center_axis',(0.905801965515954,-0.423701309022563,0.));
#32444=DIRECTION('ref_axis',(0.423701309022563,0.905801965515954,0.));
#32445=DIRECTION('',(0.,0.,1.));
#32446=DIRECTION('',(0.,0.,1.));
#32447=DIRECTION('center_axis',(-0.996089805327885,-0.0883464754353932,
0.));
#32448=DIRECTION('ref_axis',(0.0883464754353932,-0.996089805327885,0.));
#32449=DIRECTION('',(0.,0.,-1.));
#32450=DIRECTION('center_axis',(0.,0.,1.));
#32451=DIRECTION('ref_axis',(0.342020143325669,0.939692620785908,0.));
#32452=DIRECTION('center_axis',(0.,0.,-1.));
#32453=DIRECTION('ref_axis',(1.,0.,0.));
#32454=DIRECTION('',(-0.085964885527717,-0.996298167445974,0.));
#32455=DIRECTION('',(0.574555194725811,0.818465838146948,0.));
#32456=DIRECTION('center_axis',(0.818465838146948,-0.574555194725811,0.));
#32457=DIRECTION('ref_axis',(0.574555194725811,0.818465838146948,0.));
#32458=DIRECTION('',(0.,0.,1.));
#32459=DIRECTION('',(0.,0.,1.));
#32460=DIRECTION('center_axis',(-0.996298167445974,0.085964885527717,0.));
#32461=DIRECTION('ref_axis',(-0.085964885527717,-0.996298167445974,0.));
#32462=DIRECTION('',(0.,0.,-1.));
#32463=DIRECTION('center_axis',(0.,0.,1.));
#32464=DIRECTION('ref_axis',(0.5,0.866025403784439,0.));
#32465=DIRECTION('center_axis',(0.,0.,-1.));
#32466=DIRECTION('ref_axis',(1.,0.,0.));
#32467=DIRECTION('',(-0.257664246944398,-0.966234513897416,0.));
#32468=DIRECTION('',(0.707951511576272,0.706261040449544,0.));
#32469=DIRECTION('center_axis',(0.706261040449544,-0.707951511576272,0.));
#32470=DIRECTION('ref_axis',(0.707951511576272,0.706261040449544,0.));
#32471=DIRECTION('',(0.,0.,1.));
#32472=DIRECTION('',(0.,0.,1.));
#32473=DIRECTION('center_axis',(-0.966234513897416,0.257664246944398,0.));
#32474=DIRECTION('ref_axis',(-0.257664246944398,-0.966234513897416,0.));
#32475=DIRECTION('',(0.,0.,-1.));
#32476=DIRECTION('center_axis',(0.,0.,1.));
#32477=DIRECTION('ref_axis',(0.642787609686539,0.766044443118978,0.));
#32478=DIRECTION('center_axis',(0.,0.,-1.));
#32479=DIRECTION('ref_axis',(1.,0.,0.));
#32480=DIRECTION('',(-0.421534610602074,-0.906812313582341,0.));
#32481=DIRECTION('',(0.819837079988238,0.572596858423411,0.));
#32482=DIRECTION('center_axis',(0.572596858423411,-0.819837079988238,0.));
#32483=DIRECTION('ref_axis',(0.819837079988238,0.572596858423411,0.));
#32484=DIRECTION('',(0.,0.,1.));
#32485=DIRECTION('',(0.,0.,1.));
#32486=DIRECTION('center_axis',(-0.906812313582341,0.421534610602074,0.));
#32487=DIRECTION('ref_axis',(-0.421534610602074,-0.906812313582341,0.));
#32488=DIRECTION('',(0.,0.,-1.));
#32489=DIRECTION('center_axis',(0.,0.,1.));
#32490=DIRECTION('ref_axis',(0.766044443118978,0.642787609686539,0.));
#32491=DIRECTION('center_axis',(0.,0.,-1.));
#32492=DIRECTION('ref_axis',(1.,0.,0.));
#32493=DIRECTION('',(-0.572596858423411,-0.819837079988238,0.));
#32494=DIRECTION('',(0.906812313582341,0.421534610602074,0.));
#32495=DIRECTION('center_axis',(0.421534610602074,-0.906812313582341,0.));
#32496=DIRECTION('ref_axis',(0.906812313582341,0.421534610602074,0.));
#32497=DIRECTION('',(0.,0.,1.));
#32498=DIRECTION('',(0.,0.,1.));
#32499=DIRECTION('center_axis',(-0.819837079988238,0.572596858423411,0.));
#32500=DIRECTION('ref_axis',(-0.572596858423411,-0.819837079988238,0.));
#32501=DIRECTION('',(0.,0.,-1.));
#32502=DIRECTION('center_axis',(0.,0.,1.));
#32503=DIRECTION('ref_axis',(0.866025403784439,0.5,0.));
#32504=DIRECTION('center_axis',(0.,0.,-1.));
#32505=DIRECTION('ref_axis',(1.,0.,0.));
#32506=DIRECTION('',(-0.706261040449544,-0.707951511576272,0.));
#32507=DIRECTION('',(0.966234513897416,0.257664246944398,0.));
#32508=DIRECTION('center_axis',(0.257664246944398,-0.966234513897416,0.));
#32509=DIRECTION('ref_axis',(0.966234513897416,0.257664246944398,0.));
#32510=DIRECTION('',(0.,0.,1.));
#32511=DIRECTION('',(0.,0.,1.));
#32512=DIRECTION('center_axis',(-0.707951511576272,0.706261040449544,0.));
#32513=DIRECTION('ref_axis',(-0.706261040449544,-0.707951511576272,0.));
#32514=DIRECTION('',(0.,0.,-1.));
#32515=DIRECTION('center_axis',(0.,0.,1.));
#32516=DIRECTION('ref_axis',(0.939692620785909,0.342020143325669,0.));
#32517=DIRECTION('center_axis',(0.,0.,-1.));
#32518=DIRECTION('ref_axis',(1.,0.,0.));
#32519=DIRECTION('',(-0.818465838146948,-0.574555194725811,0.));
#32520=DIRECTION('',(0.996298167445974,0.0859648855277167,0.));
#32521=DIRECTION('center_axis',(0.0859648855277167,-0.996298167445974,0.));
#32522=DIRECTION('ref_axis',(0.996298167445974,0.0859648855277167,0.));
#32523=DIRECTION('',(0.,0.,1.));
#32524=DIRECTION('',(0.,0.,1.));
#32525=DIRECTION('center_axis',(-0.574555194725811,0.818465838146948,0.));
#32526=DIRECTION('ref_axis',(-0.818465838146948,-0.574555194725811,0.));
#32527=DIRECTION('',(0.,0.,-1.));
#32528=DIRECTION('center_axis',(0.,0.,1.));
#32529=DIRECTION('ref_axis',(0.984807753012208,0.17364817766693,0.));
#32530=DIRECTION('center_axis',(0.,0.,-1.));
#32531=DIRECTION('ref_axis',(1.,0.,0.));
#32532=DIRECTION('',(-0.905801965515955,-0.423701309022563,0.));
#32533=DIRECTION('',(0.996089805327885,-0.0883464754353932,0.));
#32534=DIRECTION('center_axis',(-0.0883464754353933,-0.996089805327885,
0.));
#32535=DIRECTION('ref_axis',(0.996089805327885,-0.0883464754353933,0.));
#32536=DIRECTION('',(0.,0.,1.));
#32537=DIRECTION('',(0.,0.,1.));
#32538=DIRECTION('center_axis',(-0.423701309022563,0.905801965515955,0.));
#32539=DIRECTION('ref_axis',(-0.905801965515954,-0.423701309022563,0.));
#32540=DIRECTION('',(0.,0.,-1.));
#32541=DIRECTION('center_axis',(0.,0.,1.));
#32542=DIRECTION('ref_axis',(1.,0.,0.));
#32543=DIRECTION('center_axis',(0.,0.,1.));
#32544=DIRECTION('ref_axis',(1.,0.,0.));
#32545=DIRECTION('center_axis',(0.,0.,1.));
#32546=DIRECTION('ref_axis',(1.,0.,0.));
#32547=DIRECTION('center_axis',(0.,0.,1.));
#32548=DIRECTION('ref_axis',(1.,0.,0.));
#32549=DIRECTION('center_axis',(0.,0.,1.));
#32550=DIRECTION('ref_axis',(1.,0.,0.));
#32551=DIRECTION('center_axis',(0.,0.,1.));
#32552=DIRECTION('ref_axis',(1.,0.,0.));
#32553=DIRECTION('center_axis',(0.,0.,1.));
#32554=DIRECTION('ref_axis',(1.,0.,0.));
#32555=DIRECTION('center_axis',(0.,0.,1.));
#32556=DIRECTION('ref_axis',(1.,0.,0.));
#32557=DIRECTION('center_axis',(0.,0.,1.));
#32558=DIRECTION('ref_axis',(1.,0.,0.));
#32559=DIRECTION('center_axis',(0.,0.,1.));
#32560=DIRECTION('ref_axis',(1.,0.,0.));
#32561=DIRECTION('center_axis',(0.,0.,1.));
#32562=DIRECTION('ref_axis',(1.,0.,0.));
#32563=DIRECTION('center_axis',(0.,0.,1.));
#32564=DIRECTION('ref_axis',(1.,0.,0.));
#32565=DIRECTION('center_axis',(0.,0.,1.));
#32566=DIRECTION('ref_axis',(1.,0.,0.));
#32567=DIRECTION('center_axis',(0.,0.,1.));
#32568=DIRECTION('ref_axis',(1.,0.,0.));
#32569=DIRECTION('center_axis',(0.,0.,1.));
#32570=DIRECTION('ref_axis',(1.,0.,0.));
#32571=DIRECTION('center_axis',(0.,0.,1.));
#32572=DIRECTION('ref_axis',(1.,0.,0.));
#32573=DIRECTION('center_axis',(0.,0.,1.));
#32574=DIRECTION('ref_axis',(1.,0.,0.));
#32575=DIRECTION('center_axis',(0.,0.,1.));
#32576=DIRECTION('ref_axis',(1.,0.,0.));
#32577=DIRECTION('',(0.,0.,-1.));
#32578=DIRECTION('center_axis',(0.,0.,1.));
#32579=DIRECTION('ref_axis',(1.,0.,0.));
#32580=DIRECTION('center_axis',(0.,0.,1.));
#32581=DIRECTION('ref_axis',(1.,0.,0.));
#32582=DIRECTION('center_axis',(0.,0.,1.));
#32583=DIRECTION('ref_axis',(1.,0.,0.));
#32584=DIRECTION('center_axis',(0.,0.,1.));
#32585=DIRECTION('ref_axis',(1.,0.,0.));
#32586=DIRECTION('center_axis',(0.,0.,1.));
#32587=DIRECTION('ref_axis',(1.,0.,0.));
#32588=DIRECTION('center_axis',(0.,0.,1.));
#32589=DIRECTION('ref_axis',(1.,0.,0.));
#32590=DIRECTION('center_axis',(0.,0.,1.));
#32591=DIRECTION('ref_axis',(1.,0.,0.));
#32592=DIRECTION('center_axis',(0.,0.,1.));
#32593=DIRECTION('ref_axis',(1.,0.,0.));
#32594=DIRECTION('center_axis',(0.,0.,1.));
#32595=DIRECTION('ref_axis',(1.,0.,0.));
#32596=DIRECTION('center_axis',(0.,0.,1.));
#32597=DIRECTION('ref_axis',(1.,0.,0.));
#32598=DIRECTION('center_axis',(0.,0.,1.));
#32599=DIRECTION('ref_axis',(1.,0.,0.));
#32600=DIRECTION('center_axis',(0.,0.,1.));
#32601=DIRECTION('ref_axis',(1.,0.,0.));
#32602=DIRECTION('center_axis',(0.,0.,1.));
#32603=DIRECTION('ref_axis',(1.,0.,0.));
#32604=DIRECTION('center_axis',(0.,0.,1.));
#32605=DIRECTION('ref_axis',(1.,0.,0.));
#32606=DIRECTION('center_axis',(0.,0.,1.));
#32607=DIRECTION('ref_axis',(1.,0.,0.));
#32608=DIRECTION('center_axis',(0.,0.,1.));
#32609=DIRECTION('ref_axis',(1.,0.,0.));
#32610=DIRECTION('center_axis',(0.,0.,1.));
#32611=DIRECTION('ref_axis',(1.,0.,0.));
#32612=DIRECTION('center_axis',(0.,0.,1.));
#32613=DIRECTION('ref_axis',(1.,0.,0.));
#32614=DIRECTION('center_axis',(0.,0.,1.));
#32615=DIRECTION('ref_axis',(1.,0.,0.));
#32616=DIRECTION('',(0.,0.,-1.));
#32617=DIRECTION('center_axis',(0.,0.,-1.));
#32618=DIRECTION('ref_axis',(1.,0.,0.));
#32619=DIRECTION('',(0.,0.,1.));
#32620=DIRECTION('center_axis',(0.,0.,1.));
#32621=DIRECTION('ref_axis',(1.,0.,0.));
#32622=DIRECTION('center_axis',(-0.259973473447872,-0.96561575852067,0.));
#32623=DIRECTION('ref_axis',(0.96561575852067,-0.259973473447872,0.));
#32624=DIRECTION('',(0.96561575852067,-0.259973473447872,0.));
#32625=DIRECTION('',(0.,0.,1.));
#32626=DIRECTION('center_axis',(-0.259973473447872,0.96561575852067,0.));
#32627=DIRECTION('ref_axis',(-0.96561575852067,-0.259973473447872,0.));
#32628=DIRECTION('',(-0.96561575852067,-0.259973473447872,0.));
#32629=DIRECTION('center_axis',(0.,0.,1.));
#32630=DIRECTION('ref_axis',(1.,0.,0.));
#32631=DIRECTION('center_axis',(0.,0.,-1.));
#32632=DIRECTION('ref_axis',(1.,0.,0.));
#32633=DIRECTION('center_axis',(0.,0.,1.));
#32634=DIRECTION('ref_axis',(1.,0.,0.));
#32635=DIRECTION('',(-0.707106781186548,-8.65956056235493E-17,-0.707106781186548));
#32636=DIRECTION('center_axis',(0.,0.,1.));
#32637=DIRECTION('ref_axis',(1.,0.,0.));
#32638=DIRECTION('',(-0.842487928864452,-1.03175014540413E-16,0.538715221353255));
#32639=DIRECTION('center_axis',(0.,0.,-1.));
#32640=DIRECTION('ref_axis',(1.,0.,0.));
#32641=DIRECTION('center_axis',(0.5,0.866025403784439,0.));
#32642=DIRECTION('ref_axis',(0.866025403784439,-0.5,0.));
#32643=DIRECTION('',(0.866025403784439,-0.5,0.));
#32644=DIRECTION('',(0.,0.,-1.));
#32645=DIRECTION('',(0.866025403784439,-0.5,0.));
#32646=DIRECTION('',(0.,0.,-1.));
#32647=DIRECTION('center_axis',(-0.5,0.866025403784439,0.));
#32648=DIRECTION('ref_axis',(0.866025403784439,0.5,0.));
#32649=DIRECTION('',(0.866025403784439,0.5,0.));
#32650=DIRECTION('',(0.,0.,-1.));
#32651=DIRECTION('',(0.866025403784439,0.5,0.));
#32652=DIRECTION('center_axis',(-1.,-1.60246890531964E-16,0.));
#32653=DIRECTION('ref_axis',(-1.60246890531964E-16,1.,0.));
#32654=DIRECTION('',(-1.60246890531964E-16,1.,0.));
#32655=DIRECTION('',(0.,0.,-1.));
#32656=DIRECTION('',(-1.60246890531964E-16,1.,0.));
#32657=DIRECTION('center_axis',(-0.5,-0.866025403784439,0.));
#32658=DIRECTION('ref_axis',(-0.866025403784439,0.5,0.));
#32659=DIRECTION('',(-0.866025403784439,0.5,0.));
#32660=DIRECTION('',(0.,0.,-1.));
#32661=DIRECTION('',(-0.866025403784439,0.5,0.));
#32662=DIRECTION('center_axis',(0.5,-0.866025403784439,0.));
#32663=DIRECTION('ref_axis',(-0.866025403784439,-0.5,0.));
#32664=DIRECTION('',(-0.866025403784439,-0.5,0.));
#32665=DIRECTION('',(0.,0.,-1.));
#32666=DIRECTION('',(-0.866025403784439,-0.5,0.));
#32667=DIRECTION('center_axis',(1.,-3.20493781063927E-16,0.));
#32668=DIRECTION('ref_axis',(-3.20493781063927E-16,-1.,0.));
#32669=DIRECTION('',(-3.20493781063927E-16,-1.,0.));
#32670=DIRECTION('',(-3.20493781063927E-16,-1.,0.));
#32671=DIRECTION('center_axis',(0.,0.,-1.));
#32672=DIRECTION('ref_axis',(-1.,0.,0.));
#32673=DIRECTION('center_axis',(0.,0.,-1.));
#32674=DIRECTION('ref_axis',(-1.,0.,0.));
#32675=DIRECTION('center_axis',(0.,0.,1.));
#32676=DIRECTION('ref_axis',(1.,0.,0.));
#32677=DIRECTION('center_axis',(0.,0.,1.));
#32678=DIRECTION('ref_axis',(1.,0.,0.));
#32679=DIRECTION('',(0.707106781186547,8.65956056235493E-17,-0.707106781186548));
#32680=DIRECTION('center_axis',(0.,0.,1.));
#32681=DIRECTION('ref_axis',(1.,0.,0.));
#32682=DIRECTION('center_axis',(0.,0.,1.));
#32683=DIRECTION('ref_axis',(1.,0.,0.));
#32684=DIRECTION('center_axis',(0.,0.,1.));
#32685=DIRECTION('ref_axis',(1.,0.,0.));
#32686=DIRECTION('center_axis',(0.,0.,1.));
#32687=DIRECTION('ref_axis',(1.,0.,0.));
#32688=DIRECTION('',(0.707106781186548,8.65956056235494E-17,-0.707106781186547));
#32689=DIRECTION('center_axis',(0.,0.,-1.));
#32690=DIRECTION('ref_axis',(-1.,0.,0.));
#32691=DIRECTION('center_axis',(0.,0.,1.));
#32692=DIRECTION('ref_axis',(1.,0.,0.));
#44628=CARTESIAN_POINT('',(0.,0.,0.));
#44629=CARTESIAN_POINT('Origin',(0.,0.,-0.493));
#44630=CARTESIAN_POINT('',(-0.0966111239073705,-8.03799554811163E-5,-0.926426408311032));
#44631=CARTESIAN_POINT('',(-0.0966191160461945,-8.04235544959989E-5,-0.932223591688968));
#44632=CARTESIAN_POINT('',(-0.096675,-1.1839272930757E-17,-0.493));
#44633=CARTESIAN_POINT('',(0.0869479092309507,-0.0426124462865253,-0.949325));
#44634=CARTESIAN_POINT('Ctrl Pts',(-0.0966111239073705,-8.03799554811163E-5,
-0.926426408311032));
#44635=CARTESIAN_POINT('Ctrl Pts',(-0.0964350902968673,0.0222712561995875,
-0.927896221307833));
#44636=CARTESIAN_POINT('Ctrl Pts',(-0.0887114911241552,0.044734022366812,
-0.929366034304633));
#44637=CARTESIAN_POINT('Ctrl Pts',(-0.0745208699991529,0.0618333618915069,
-0.930835847301434));
#44638=CARTESIAN_POINT('Ctrl Pts',(-0.0541569551612004,0.0863713641959035,
-0.932945067640058));
#44639=CARTESIAN_POINT('Ctrl Pts',(-0.0204754984960076,0.0998644590952887,
-0.935054287978682));
#44640=CARTESIAN_POINT('Ctrl Pts',(0.0111920394192712,0.0961816327255734,
-0.937163508317306));
#44641=CARTESIAN_POINT('Ctrl Pts',(0.0428595773345502,0.0924988063558581,
-0.93927272865593));
#44642=CARTESIAN_POINT('Ctrl Pts',(0.0725131964999154,0.0716400587170422,
-0.941381948994554));
#44643=CARTESIAN_POINT('Ctrl Pts',(0.0867090407236772,0.0430821191108494,
-0.943491169333178));
#44644=CARTESIAN_POINT('Ctrl Pts',(0.0997969971053929,0.0167529299463267,
-0.945435779555452));
#44645=CARTESIAN_POINT('Ctrl Pts',(0.0997457751378415,-0.0161206070811178,
-0.947380389777726));
#44646=CARTESIAN_POINT('Ctrl Pts',(0.0869479092309507,-0.0426124462865253,
-0.949325));
#44647=CARTESIAN_POINT('',(-0.096675,-1.1839272930757E-17,-0.949325));
#44648=CARTESIAN_POINT('Origin',(0.,0.,-0.949325));
#44649=CARTESIAN_POINT('',(-0.096675,-1.1839272930757E-17,-0.979325));
#44650=CARTESIAN_POINT('',(-0.096675,-1.1839272930757E-17,-0.493));
#44651=CARTESIAN_POINT('Origin',(0.,0.,-0.979325));
#44652=CARTESIAN_POINT('',(0.0868262223680489,0.042511912851507,-0.949325));
#44653=CARTESIAN_POINT('Origin',(0.,0.,-0.949325));
#44654=CARTESIAN_POINT('Ctrl Pts',(0.0868262223680489,0.042511912851507,
-0.949325));
#44655=CARTESIAN_POINT('Ctrl Pts',(0.0727413643237034,0.0712787909934627,
-0.947215779661376));
#44656=CARTESIAN_POINT('Ctrl Pts',(0.0433671481397557,0.0922558111466541,
-0.945106559322752));
#44657=CARTESIAN_POINT('Ctrl Pts',(0.0117674690472282,0.0961065728543937,
-0.942997338984128));
#44658=CARTESIAN_POINT('Ctrl Pts',(-0.0198322100452994,0.0999573345621333,
-0.940888118645504));
#44659=CARTESIAN_POINT('Ctrl Pts',(-0.0536573520464067,0.0866818378244212,
-0.938778898306881));
#44660=CARTESIAN_POINT('Ctrl Pts',(-0.0741790245420598,0.0622672145784177,
-0.936669677968257));
#44661=CARTESIAN_POINT('Ctrl Pts',(-0.0885984326427958,0.0451124521542337,
-0.935187649208494));
#44662=CARTESIAN_POINT('Ctrl Pts',(-0.0964498235569402,0.022458224021493,
-0.933705620448731));
#44663=CARTESIAN_POINT('Ctrl Pts',(-0.0966191160461945,-8.04235544959989E-5,
-0.932223591688968));
#44664=CARTESIAN_POINT('Origin',(0.,0.,-0.493));
#44665=CARTESIAN_POINT('',(-0.0968293357490093,1.06988599727479E-5,-0.886426408311032));
#44666=CARTESIAN_POINT('',(-0.0968280577919496,1.39804010291189E-5,-0.892223591688968));
#44667=CARTESIAN_POINT('',(-0.096675,-1.1839272930757E-17,-0.493));
#44668=CARTESIAN_POINT('Ctrl Pts',(-0.0968293357490093,1.06988599727479E-5,
-0.886426408311032));
#44669=CARTESIAN_POINT('Ctrl Pts',(-0.0968302582891165,0.00059431625353822,
-0.886465012270798));
#44670=CARTESIAN_POINT('Ctrl Pts',(-0.096825435141126,0.00117791800451826,
-0.886503616230564));
#44671=CARTESIAN_POINT('Ctrl Pts',(-0.0968148197274314,0.00176141437737019,
-0.88654222019033));
#44672=CARTESIAN_POINT('Ctrl Pts',(-0.0962348210277351,0.0336421443489341,
-0.888651440528954));
#44673=CARTESIAN_POINT('Ctrl Pts',(-0.0783634816289883,0.0652082946364147,
-0.890760660867579));
#44674=CARTESIAN_POINT('Ctrl Pts',(-0.0513251420952661,0.0821094183977308,
-0.892869881206202));
#44675=CARTESIAN_POINT('Ctrl Pts',(-0.0242868025615438,0.0990105421590469,
-0.894979101544826));
#44676=CARTESIAN_POINT('Ctrl Pts',(0.0119185371071539,0.101246639394198,
-0.89708832188345));
#44677=CARTESIAN_POINT('Ctrl Pts',(0.0408310098562432,0.0878012164778136,
-0.899197542222074));
#44678=CARTESIAN_POINT('Ctrl Pts',(0.0697434826053325,0.074355793561429,
-0.901306762560698));
#44679=CARTESIAN_POINT('Ctrl Pts',(0.0913630884348138,0.0452288504935087,
-0.903415982899322));
#44680=CARTESIAN_POINT('Ctrl Pts',(0.0958620419187354,0.0136617734053438,
-0.905525203237946));
#44681=CARTESIAN_POINT('Ctrl Pts',(0.100360995402657,-0.017905303682821,
-0.90763442357657));
#44682=CARTESIAN_POINT('Ctrl Pts',(0.087739296541019,-0.0519125147912303,
-0.909743643915194));
#44683=CARTESIAN_POINT('Ctrl Pts',(0.0637334499829788,-0.0728994661690192,
-0.911852864253818));
#44684=CARTESIAN_POINT('Ctrl Pts',(0.0397276034249385,-0.0938864175468081,
-0.913962084592442));
#44685=CARTESIAN_POINT('Ctrl Pts',(0.00433760917049605,-0.101853109193976,
-0.916071304931066));
#44686=CARTESIAN_POINT('Ctrl Pts',(-0.0263449122524892,-0.0931782315159874,
-0.91818052526969));
#44687=CARTESIAN_POINT('Ctrl Pts',(-0.0570274336754744,-0.0845033538379983,
-0.920289745608314));
#44688=CARTESIAN_POINT('Ctrl Pts',(-0.0830024822670023,-0.0591869068348518,
-0.922398965946938));
#44689=CARTESIAN_POINT('Ctrl Pts',(-0.0924668200574101,-0.0287372284785746,
-0.924508186285562));
#44690=CARTESIAN_POINT('Ctrl Pts',(-0.0953359214774314,-0.0195064489622592,
-0.925147593627386));
#44691=CARTESIAN_POINT('Ctrl Pts',(-0.0966877031614718,-0.00980393001962354,
-0.925787000969209));
#44692=CARTESIAN_POINT('Ctrl Pts',(-0.0966111239073705,-8.03799554811163E-5,
-0.926426408311032));
#44693=CARTESIAN_POINT('Ctrl Pts',(-0.0966191160461945,-8.04235544959989E-5,
-0.932223591688968));
#44694=CARTESIAN_POINT('Ctrl Pts',(-0.0966907602858392,-0.00961873370229752,
-0.931596400110107));
#44695=CARTESIAN_POINT('Ctrl Pts',(-0.0953865673460834,-0.0191363437733232,
-0.930969208531246));
#44696=CARTESIAN_POINT('Ctrl Pts',(-0.0926220973441531,-0.0282076709356274,
-0.930342016952384));
#44697=CARTESIAN_POINT('Ctrl Pts',(-0.0833252946603945,-0.0587141834493743,
-0.92823279661376));
#44698=CARTESIAN_POINT('Ctrl Pts',(-0.0575134863026783,-0.0841734587225733,
-0.926123576275137));
#44699=CARTESIAN_POINT('Ctrl Pts',(-0.0268854626848309,-0.0930233302060816,
-0.924014355936513));
#44700=CARTESIAN_POINT('Ctrl Pts',(0.00374256093301658,-0.10187320168959,
-0.921905135597888));
#44701=CARTESIAN_POINT('Ctrl Pts',(0.0391867998109952,-0.0941136693834075,
-0.919795915259264));
#44702=CARTESIAN_POINT('Ctrl Pts',(0.063315182280828,-0.0732660374240845,
-0.91768669492064));
#44703=CARTESIAN_POINT('Ctrl Pts',(0.0874435647506607,-0.0524184054647615,
-0.915577474582016));
#44704=CARTESIAN_POINT('Ctrl Pts',(0.100256090812348,-0.018482673852298,
-0.913468254243393));
#44705=CARTESIAN_POINT('Ctrl Pts',(0.0959378107493762,0.0131101896102531,
-0.911359033904769));
#44706=CARTESIAN_POINT('Ctrl Pts',(0.0916195306864047,0.0447030530728043,
-0.909249813566145));
#44707=CARTESIAN_POINT('Ctrl Pts',(0.0701704444987747,0.0739530483854431,
-0.90714059322752));
#44708=CARTESIAN_POINT('Ctrl Pts',(0.0413364389978215,0.087564466214271,
-0.905031372888896));
#44709=CARTESIAN_POINT('Ctrl Pts',(0.0125024334968684,0.101175884043099,
-0.902922152550272));
#44710=CARTESIAN_POINT('Ctrl Pts',(-0.0237164913174078,0.0991487243881159,
-0.900812932211648));
#44711=CARTESIAN_POINT('Ctrl Pts',(-0.0508519843711625,0.0824036418801622,
-0.898703711873024));
#44712=CARTESIAN_POINT('Ctrl Pts',(-0.0779874774249174,0.0656585593722084,
-0.896594491534401));
#44713=CARTESIAN_POINT('Ctrl Pts',(-0.0960395387181506,0.0341955540112833,
-0.894485271195776));
#44714=CARTESIAN_POINT('Ctrl Pts',(-0.0968028858565612,0.00231863128268832,
-0.892376050857152));
#44715=CARTESIAN_POINT('Ctrl Pts',(-0.0968212780032749,0.00155058616913002,
-0.892325231134424));
#44716=CARTESIAN_POINT('Ctrl Pts',(-0.0968296336248802,0.000782300766327763,
-0.892274411411696));
#44717=CARTESIAN_POINT('Ctrl Pts',(-0.0968280577919496,1.39804010291189E-5,
-0.892223591688968));
#44718=CARTESIAN_POINT('Origin',(0.,0.,-0.493));
#44719=CARTESIAN_POINT('',(-0.0965815334425764,7.1292991562881E-5,-0.846426408311032));
#44720=CARTESIAN_POINT('',(-0.0965773242360877,6.95087071336693E-5,-0.852223591688968));
#44721=CARTESIAN_POINT('',(-0.096675,-1.1839272930757E-17,-0.493));
#44722=CARTESIAN_POINT('Ctrl Pts',(-0.0965815334425764,7.1292991562881E-5,
-0.846426408311032));
#44723=CARTESIAN_POINT('Ctrl Pts',(-0.096656839197146,0.0109770781310021,
-0.847143023572388));
#44724=CARTESIAN_POINT('Ctrl Pts',(-0.0949511484573878,0.0218600075058422,
-0.847859638833743));
#44725=CARTESIAN_POINT('Ctrl Pts',(-0.091361885510168,0.0320815246121575,
-0.848576254095099));
#44726=CARTESIAN_POINT('Ctrl Pts',(-0.080797574620909,0.0621666106197558,
-0.850685474433722));
#44727=CARTESIAN_POINT('Ctrl Pts',(-0.0539157469163047,0.0865218362212725,
-0.852794694772346));
#44728=CARTESIAN_POINT('Ctrl Pts',(-0.0229372507921025,0.0940749760435912,
-0.854903915110971));
#44729=CARTESIAN_POINT('Ctrl Pts',(0.00804124533209912,0.10162811586591,
-0.857013135449595));
#44730=CARTESIAN_POINT('Ctrl Pts',(0.0431164098758985,0.092379169909031,
-0.859122355788219));
#44731=CARTESIAN_POINT('Ctrl Pts',(0.0663425758270414,0.0705328392060976,
-0.861231576126843));
#44732=CARTESIAN_POINT('Ctrl Pts',(0.0895687417781846,0.0486865085031638,
-0.863340796465467));
#44733=CARTESIAN_POINT('Ctrl Pts',(0.100945909136671,0.0142427930541751,
-0.86545001680409));
#44734=CARTESIAN_POINT('Ctrl Pts',(0.0953018761651522,-0.0171397173428181,
-0.867559237142714));
#44735=CARTESIAN_POINT('Ctrl Pts',(0.0896578431936334,-0.0485222277398107,
-0.869668457481338));
#44736=CARTESIAN_POINT('Ctrl Pts',(0.06699260989211,-0.0768435330848077,
-0.871777677819963));
#44737=CARTESIAN_POINT('Ctrl Pts',(0.037610074738181,-0.0892283685032535,
-0.873886898158587));
#44738=CARTESIAN_POINT('Ctrl Pts',(0.00822753958425157,-0.101613203921699,
-0.875996118497211));
#44739=CARTESIAN_POINT('Ctrl Pts',(-0.0278722974220837,-0.0980615694135937,
-0.878105338835835));
#44740=CARTESIAN_POINT('Ctrl Pts',(-0.0542778869249285,-0.0801880973317172,
-0.880214559174458));
#44741=CARTESIAN_POINT('Ctrl Pts',(-0.0802001886952881,-0.0626417540872089,
-0.882285175553316));
#44742=CARTESIAN_POINT('Ctrl Pts',(-0.0967798530879647,-0.0312930259762486,
-0.884355791932174));
#44743=CARTESIAN_POINT('Ctrl Pts',(-0.0968293357490093,1.06988599727479E-5,
-0.886426408311032));
#44744=CARTESIAN_POINT('Ctrl Pts',(-0.0968280577919496,1.39804010291189E-5,
-0.892223591688968));
#44745=CARTESIAN_POINT('Ctrl Pts',(-0.0967642302993774,-0.0311060460027344,
-0.890165191073072));
#44746=CARTESIAN_POINT('Ctrl Pts',(-0.080407139247537,-0.0622834308897126,
-0.888106790457176));
#44747=CARTESIAN_POINT('Ctrl Pts',(-0.0547386896099341,-0.0798742794120905,
-0.886048389841281));
#44748=CARTESIAN_POINT('Ctrl Pts',(-0.028436513241308,-0.0978994272820098,
-0.883939169502657));
#44749=CARTESIAN_POINT('Ctrl Pts',(0.00764247247953262,-0.101658882925584,
-0.881829949164033));
#44750=CARTESIAN_POINT('Ctrl Pts',(0.0370958592149572,-0.0894434105834474,
-0.879720728825409));
#44751=CARTESIAN_POINT('Ctrl Pts',(0.0665492459503818,-0.0772279382413112,
-0.877611508486785));
#44752=CARTESIAN_POINT('Ctrl Pts',(0.0893770337003904,-0.0490375379134651,
-0.87550228814816));
#44753=CARTESIAN_POINT('Ctrl Pts',(0.0952016028206863,-0.0176880291495755,
-0.873393067809536));
#44754=CARTESIAN_POINT('Ctrl Pts',(0.101026171940982,0.0136614796143141,
-0.871283847470913));
#44755=CARTESIAN_POINT('Ctrl Pts',(0.089847522431565,0.0481700968142471,
-0.869174627132289));
#44756=CARTESIAN_POINT('Ctrl Pts',(0.0667475130189973,0.0701497621673904,
-0.867065406793665));
#44757=CARTESIAN_POINT('Ctrl Pts',(0.0436475036064297,0.0921294275205335,
-0.864956186455041));
#44758=CARTESIAN_POINT('Ctrl Pts',(0.00862613429071169,0.101580141026887,
-0.862846966116416));
#44759=CARTESIAN_POINT('Ctrl Pts',(-0.0223953343972411,0.09420545699243,
-0.860737745777792));
#44760=CARTESIAN_POINT('Ctrl Pts',(-0.053416803085194,0.0868307729579728,
-0.858628525439168));
#44761=CARTESIAN_POINT('Ctrl Pts',(-0.0804383711453816,0.0626306913827048,
-0.856519305100545));
#44762=CARTESIAN_POINT('Ctrl Pts',(-0.0911756884108397,0.0326069166667885,
-0.854410084761921));
#44763=CARTESIAN_POINT('Ctrl Pts',(-0.0948859171611054,0.0222323445657248,
-0.853681253737604));
#44764=CARTESIAN_POINT('Ctrl Pts',(-0.0966517818572679,0.0111624147385034,
-0.852952422713286));
#44765=CARTESIAN_POINT('Ctrl Pts',(-0.0965773242360877,6.95087071336693E-5,
-0.852223591688968));
#44766=CARTESIAN_POINT('Origin',(0.,0.,-0.493));
#44767=CARTESIAN_POINT('',(-0.0965822410032082,-7.15798389840372E-5,-0.806426408311033));
#44768=CARTESIAN_POINT('',(-0.0965865764190601,-7.32614358284168E-5,-0.812223591688968));
#44769=CARTESIAN_POINT('',(-0.096675,-1.1839272930757E-17,-0.493));
#44770=CARTESIAN_POINT('Ctrl Pts',(-0.0965822410032082,-7.15798389840372E-5,
-0.806426408311033));
#44771=CARTESIAN_POINT('Ctrl Pts',(-0.0964350243461911,0.021152105978162,
-0.807821034873977));
#44772=CARTESIAN_POINT('Ctrl Pts',(-0.0895412391802931,0.0424627517956176,
-0.809215661436921));
#44773=CARTESIAN_POINT('Ctrl Pts',(-0.0766614365121771,0.0591543965841834,
-0.810610287999866));
#44774=CARTESIAN_POINT('Ctrl Pts',(-0.0571821418630841,0.0843986860653691,
-0.81271950833849));
#44775=CARTESIAN_POINT('Ctrl Pts',(-0.0240108747313753,0.0990778151604882,
-0.814828728677115));
#44776=CARTESIAN_POINT('Ctrl Pts',(0.00777224516368064,0.096518447416171,
-0.816937949015739));
#44777=CARTESIAN_POINT('Ctrl Pts',(0.0395553650587365,0.0939590796718537,
-0.819047169354363));
#44778=CARTESIAN_POINT('Ctrl Pts',(0.0699503377171397,0.0741612150881001,
-0.821156389692986));
#44779=CARTESIAN_POINT('Ctrl Pts',(0.0851391852437711,0.0461252385447729,
-0.82326561003161));
#44780=CARTESIAN_POINT('Ctrl Pts',(0.100328032770402,0.0180892620014455,
-0.825374830370234));
#44781=CARTESIAN_POINT('Ctrl Pts',(0.100310755165262,-0.0181848265014556,
-0.827484050708859));
#44782=CARTESIAN_POINT('Ctrl Pts',(0.0850952074316202,-0.0462063214123137,
-0.829593271047483));
#44783=CARTESIAN_POINT('Ctrl Pts',(0.0698796596979782,-0.0742278163231718,
-0.831702491386107));
#44784=CARTESIAN_POINT('Ctrl Pts',(0.0394658418358345,-0.0939967176419867,
-0.833811711724731));
#44785=CARTESIAN_POINT('Ctrl Pts',(0.00768029815127167,-0.096525807511727,
-0.835920932063354));
#44786=CARTESIAN_POINT('Ctrl Pts',(-0.0241052455332914,-0.0990548973814673,
-0.838030152401978));
#44787=CARTESIAN_POINT('Ctrl Pts',(-0.0572625150402736,-0.0843441758021326,
-0.840139372740602));
#44788=CARTESIAN_POINT('Ctrl Pts',(-0.0767177527568075,-0.0590813418056254,
-0.842248593079227));
#44789=CARTESIAN_POINT('Ctrl Pts',(-0.0895630028842492,-0.0424016473016928,
-0.843641198156495));
#44790=CARTESIAN_POINT('Ctrl Pts',(-0.0964351910719676,-0.0211220203186491,
-0.845033803233764));
#44791=CARTESIAN_POINT('Ctrl Pts',(-0.0965815334425764,7.1292991562881E-5,
-0.846426408311032));
#44792=CARTESIAN_POINT('Ctrl Pts',(-0.0965773242360877,6.95087071336693E-5,
-0.852223591688968));
#44793=CARTESIAN_POINT('Ctrl Pts',(-0.0964363032021079,-0.0209402019657099,
-0.850843202374662));
#44794=CARTESIAN_POINT('Ctrl Pts',(-0.0896937709124859,-0.042032331717466,
-0.849462813060355));
#44795=CARTESIAN_POINT('Ctrl Pts',(-0.0770565847627674,-0.0586387344727256,
-0.848082423746049));
#44796=CARTESIAN_POINT('Ctrl Pts',(-0.0577470973785083,-0.084013143039759,
-0.845973203407424));
#44797=CARTESIAN_POINT('Ctrl Pts',(-0.0246750561392616,-0.0989144923172608,
-0.843863983068801));
#44798=CARTESIAN_POINT('Ctrl Pts',(0.00712452003262372,-0.0965684185823616,
-0.841754762730177));
#44799=CARTESIAN_POINT('Ctrl Pts',(0.0389240962045089,-0.0942223448474623,
-0.839645542391553));
#44800=CARTESIAN_POINT('Ctrl Pts',(0.0694512073090326,-0.0746288481001618,
-0.837536322052929));
#44801=CARTESIAN_POINT('Ctrl Pts',(0.0848278081861491,-0.0466954062534146,
-0.835427101714305));
#44802=CARTESIAN_POINT('Ctrl Pts',(0.100204409063266,-0.0187619644066672,
-0.833317881375681));
#44803=CARTESIAN_POINT('Ctrl Pts',(0.100430499712975,0.0175114225395272,
-0.831208661037057));
#44804=CARTESIAN_POINT('Ctrl Pts',(0.0854032937950573,0.0456343687175503,
-0.829099440698433));
#44805=CARTESIAN_POINT('Ctrl Pts',(0.0703760878771397,0.0737573148955733,
-0.826990220359809));
#44806=CARTESIAN_POINT('Ctrl Pts',(0.0400955853915954,0.0937298203054251,
-0.824881000021185));
#44807=CARTESIAN_POINT('Ctrl Pts',(0.00832772556442014,0.0964721055228851,
-0.822771779682561));
#44808=CARTESIAN_POINT('Ctrl Pts',(-0.023440134262755,0.0992143907403452,
-0.820662559343937));
#44809=CARTESIAN_POINT('Ctrl Pts',(-0.0566953514315609,0.0847264557654135,
-0.818553339005313));
#44810=CARTESIAN_POINT('Ctrl Pts',(-0.0763196419287051,0.0595947177503087,
-0.816444118666689));
#44811=CARTESIAN_POINT('Ctrl Pts',(-0.08940897260778,0.0428319395256663,
-0.815037276340782));
#44812=CARTESIAN_POINT('Ctrl Pts',(-0.0964341198149447,0.0213339018407355,
-0.813630434014875));
#44813=CARTESIAN_POINT('Ctrl Pts',(-0.0965865764190601,-7.32614358284168E-5,
-0.812223591688968));
#44814=CARTESIAN_POINT('Origin',(0.,0.,-0.493));
#44815=CARTESIAN_POINT('',(-0.0968295223683655,-1.01472914774969E-5,-0.766426408311033));
#44816=CARTESIAN_POINT('',(-0.0968302674661193,-6.76949675972993E-6,-0.772223591688968));
#44817=CARTESIAN_POINT('',(-0.096675,-1.1839272930757E-17,-0.493));
#44818=CARTESIAN_POINT('Ctrl Pts',(-0.0968295223683655,-1.01472914774969E-5,
-0.766426408311033));
#44819=CARTESIAN_POINT('Ctrl Pts',(-0.0967824824364324,0.0313240025753763,
-0.768499046175567));
#44820=CARTESIAN_POINT('Ctrl Pts',(-0.0801658005353392,0.0627010190930274,
-0.7705716840401));
#44821=CARTESIAN_POINT('Ctrl Pts',(-0.0542014570286708,0.0802397690797426,
-0.772644321904635));
#44822=CARTESIAN_POINT('Ctrl Pts',(-0.0277788376505428,0.0980880815220773,
-0.774753542243259));
#44823=CARTESIAN_POINT('Ctrl Pts',(0.00832433161131209,0.101605320043514,
-0.776862762581884));
#44824=CARTESIAN_POINT('Ctrl Pts',(0.0376950474149603,0.0891924990478497,
-0.778971982920508));
#44825=CARTESIAN_POINT('Ctrl Pts',(0.067065763218609,0.0767796780521847,
-0.781081203259132));
#44826=CARTESIAN_POINT('Ctrl Pts',(0.0897040255640509,0.0484367975394173,
-0.783190423597755));
#44827=CARTESIAN_POINT('Ctrl Pts',(0.0953181652342701,0.0170489255568315,
-0.785299643936379));
#44828=CARTESIAN_POINT('Ctrl Pts',(0.100932304904489,-0.0143389464257542,
-0.787408864275003));
#44829=CARTESIAN_POINT('Ctrl Pts',(0.0895223218994858,-0.0487718098781582,
-0.789518084613627));
#44830=CARTESIAN_POINT('Ctrl Pts',(0.0662753533412323,-0.0705960057310972,
-0.791627304952251));
#44831=CARTESIAN_POINT('Ctrl Pts',(0.0430283847829787,-0.0924202015840362,
-0.793736525290875));
#44832=CARTESIAN_POINT('Ctrl Pts',(0.007944430671475,-0.10163572983751,
-0.795845745629498));
#44833=CARTESIAN_POINT('Ctrl Pts',(-0.0230268550599761,-0.0940530830543341,
-0.797954965968123));
#44834=CARTESIAN_POINT('Ctrl Pts',(-0.0539981407914274,-0.0864704362711582,
-0.800064186306747));
#44835=CARTESIAN_POINT('Ctrl Pts',(-0.0808567581428261,-0.0620896144513321,
-0.802173406645372));
#44836=CARTESIAN_POINT('Ctrl Pts',(-0.0913924057352866,-0.0319944786077929,
-0.804282626983995));
#44837=CARTESIAN_POINT('Ctrl Pts',(-0.0949618328143147,-0.0217983903384935,
-0.804997220759675));
#44838=CARTESIAN_POINT('Ctrl Pts',(-0.0966576734591616,-0.0109464005149062,
-0.805711814535354));
#44839=CARTESIAN_POINT('Ctrl Pts',(-0.0965822410032082,-7.15798389840372E-5,
-0.806426408311033));
#44840=CARTESIAN_POINT('Ctrl Pts',(-0.0965865764190601,-7.32614358284168E-5,
-0.812223591688968));
#44841=CARTESIAN_POINT('Ctrl Pts',(-0.0966626916770759,-0.0107609700178141,
-0.811521213676251));
#44842=CARTESIAN_POINT('Ctrl Pts',(-0.0950257264917633,-0.0214260273296114,
-0.810818835663534));
#44843=CARTESIAN_POINT('Ctrl Pts',(-0.0915750664262514,-0.0314678465331367,
-0.810116457650817));
#44844=CARTESIAN_POINT('Ctrl Pts',(-0.0812128366011709,-0.0616231317461982,
-0.808007237312193));
#44845=CARTESIAN_POINT('Ctrl Pts',(-0.054495013125528,-0.0861581611170432,
-0.805898016973569));
#44846=CARTESIAN_POINT('Ctrl Pts',(-0.0235678906783709,-0.0939189686756064,
-0.803788796634945));
#44847=CARTESIAN_POINT('Ctrl Pts',(0.00735923176878642,-0.10167977623417,
-0.801679576296321));
#44848=CARTESIAN_POINT('Ctrl Pts',(0.042495653187458,-0.0926663619804508,
-0.799570355957697));
#44849=CARTESIAN_POINT('Ctrl Pts',(0.0658678673583969,-0.0709763495441025,
-0.797461135619073));
#44850=CARTESIAN_POINT('Ctrl Pts',(0.0892400815293357,-0.0492863371077543,
-0.795351915280449));
#44851=CARTESIAN_POINT('Ctrl Pts',(0.100848088452542,-0.0149197264887765,
-0.793242694941826));
#44852=CARTESIAN_POINT('Ctrl Pts',(0.0954147265327156,0.0164999427199751,
-0.791133474603202));
#44853=CARTESIAN_POINT('Ctrl Pts',(0.0899813646128891,0.0479196119287269,
-0.789024254264578));
#44854=CARTESIAN_POINT('Ctrl Pts',(0.0675066338500296,0.0763923397272526,
-0.786915033925953));
#44855=CARTESIAN_POINT('Ctrl Pts',(0.0382078597500414,0.0889740276760835,
-0.784805813587329));
#44856=CARTESIAN_POINT('Ctrl Pts',(0.00890908565005346,0.101555715624914,
-0.782696593248705));
#44857=CARTESIAN_POINT('Ctrl Pts',(-0.0272137317870626,0.0982463637240508,
-0.780587372910081));
#44858=CARTESIAN_POINT('Ctrl Pts',(-0.0537386568974374,0.0805504494224217,
-0.778478152571458));
#44859=CARTESIAN_POINT('Ctrl Pts',(-0.0799571535252079,0.0630589666939328,
-0.776393298943961));
#44860=CARTESIAN_POINT('Ctrl Pts',(-0.0967982356800078,0.0315114022882873,
-0.774308445316464));
#44861=CARTESIAN_POINT('Ctrl Pts',(-0.0968302674661193,-6.76949675972993E-6,
-0.772223591688968));
#44862=CARTESIAN_POINT('Origin',(0.,0.,-0.493));
#44863=CARTESIAN_POINT('',(-0.096609779660466,8.02748517758078E-5,-0.726426408311033));
#44864=CARTESIAN_POINT('',(-0.0966049344323358,7.90599391692882E-5,-0.732223591688968));
#44865=CARTESIAN_POINT('',(-0.096675,-1.1839272930757E-17,-0.493));
#44866=CARTESIAN_POINT('Ctrl Pts',(-0.096609779660466,8.02748517758078E-5,
-0.726426408311033));
#44867=CARTESIAN_POINT('Ctrl Pts',(-0.096687244674842,0.00983463108919295,
-0.727067837138532));
#44868=CARTESIAN_POINT('Ctrl Pts',(-0.0953275566972926,0.0195678958140022,
-0.727709265966032));
#44869=CARTESIAN_POINT('Ctrl Pts',(-0.092440982531473,0.0288250452673198,
-0.728350694793532));
#44870=CARTESIAN_POINT('Ctrl Pts',(-0.0829490160365677,0.0592654730552798,
-0.730459915132156));
#44871=CARTESIAN_POINT('Ctrl Pts',(-0.0569468007063695,0.0845576575314614,
-0.732569135470779));
#44872=CARTESIAN_POINT('Ctrl Pts',(-0.0262553056107718,0.0932034195366821,
-0.734678355809403));
#44873=CARTESIAN_POINT('Ctrl Pts',(0.00443618948482572,0.101849181541903,
-0.736787576148027));
#44874=CARTESIAN_POINT('Ctrl Pts',(0.0398169643458228,0.0938485210761628,
-0.738896796486651));
#44875=CARTESIAN_POINT('Ctrl Pts',(0.0638024261793546,0.072838649765581,
-0.741006016825275));
#44876=CARTESIAN_POINT('Ctrl Pts',(0.0877878880128864,0.0518287784549991,
-0.7431152371639));
#44877=CARTESIAN_POINT('Ctrl Pts',(0.100378036818953,0.0178096962995753,
-0.745224457502523));
#44878=CARTESIAN_POINT('Ctrl Pts',(0.0958492156808683,-0.0137530483680479,
-0.747333677841147));
#44879=CARTESIAN_POINT('Ctrl Pts',(0.0913203945427836,-0.0453157930356709,
-0.749442898179771));
#44880=CARTESIAN_POINT('Ctrl Pts',(0.0696726034605476,-0.0744222002154934,
-0.751552118518395));
#44881=CARTESIAN_POINT('Ctrl Pts',(0.0407472296224764,-0.0878400920089121,
-0.753661338857019));
#44882=CARTESIAN_POINT('Ctrl Pts',(0.0118218557844046,-0.101257983802331,
-0.755770559195643));
#44883=CARTESIAN_POINT('Ctrl Pts',(-0.0243811008095024,-0.0989873602093457,
-0.757879779534267));
#44884=CARTESIAN_POINT('Ctrl Pts',(-0.0514032721051547,-0.082060478324969,
-0.759988999872891));
#44885=CARTESIAN_POINT('Ctrl Pts',(-0.0784254434008066,-0.0651335964405926,
-0.762098220211515));
#44886=CARTESIAN_POINT('Ctrl Pts',(-0.0962668293982039,-0.0335504562648253,
-0.76420744055014));
#44887=CARTESIAN_POINT('Ctrl Pts',(-0.0968164876497021,-0.00166919299532548,
-0.766316660888763));
#44888=CARTESIAN_POINT('Ctrl Pts',(-0.0968260209632092,-0.00111624199909807,
-0.766353243362853));
#44889=CARTESIAN_POINT('Ctrl Pts',(-0.0968303526326005,-0.000563201322402664,
-0.766389825836943));
#44890=CARTESIAN_POINT('Ctrl Pts',(-0.0968295223683655,-1.01472914774969E-5,
-0.766426408311033));
#44891=CARTESIAN_POINT('Ctrl Pts',(-0.0968302674661193,-6.76949675972993E-6,
-0.772223591688968));
#44892=CARTESIAN_POINT('Ctrl Pts',(-0.0968306418373791,-0.00037513789299813,
-0.77219922497784));
#44893=CARTESIAN_POINT('Ctrl Pts',(-0.096828720134703,-0.000743502274278584,
-0.772174858266713));
#44894=CARTESIAN_POINT('Ctrl Pts',(-0.0968244904936179,-0.00111184015339449,
-0.772150491555585));
#44895=CARTESIAN_POINT('Ctrl Pts',(-0.0964583661957905,-0.0329957387251863,
-0.770041271216961));
#44896=CARTESIAN_POINT('Ctrl Pts',(-0.0787990848165025,-0.064681059166375,
-0.767932050878338));
#44897=CARTESIAN_POINT('Ctrl Pts',(-0.0518748015122534,-0.0817632137069352,
-0.765822830539714));
#44898=CARTESIAN_POINT('Ctrl Pts',(-0.0249505182080041,-0.0988453682474956,
-0.76371361020109));
#44899=CARTESIAN_POINT('Ctrl Pts',(0.0112387670212067,-0.101324356887427,
-0.761604389862466));
#44900=CARTESIAN_POINT('Ctrl Pts',(0.0402409013157684,-0.0880731968813481,
-0.759495169523841));
#44901=CARTESIAN_POINT('Ctrl Pts',(0.06924303561033,-0.0748220368752688,
-0.757385949185217));
#44902=CARTESIAN_POINT('Ctrl Pts',(0.0910580189702425,-0.0458407282231786,
-0.755276728846593));
#44903=CARTESIAN_POINT('Ctrl Pts',(0.0957684562693173,-0.0143045772911135,
-0.753167508507969));
#44904=CARTESIAN_POINT('Ctrl Pts',(0.100478893568392,0.0172315736409515,
-0.751058288169346));
#44905=CARTESIAN_POINT('Ctrl Pts',(0.0880847848066293,0.0513225668529911,
-0.748949067830722));
#44906=CARTESIAN_POINT('Ctrl Pts',(0.0642206643679629,0.0724701622447588,
-0.746839847492098));
#44907=CARTESIAN_POINT('Ctrl Pts',(0.0403565439292966,0.0936177576365265,
-0.744730627153474));
#44908=CARTESIAN_POINT('Ctrl Pts',(0.00502241181372707,0.101821955208023,
-0.74262140681485));
#44909=CARTESIAN_POINT('Ctrl Pts',(-0.0257183436275326,0.0933530125314768,
-0.740512186476226));
#44910=CARTESIAN_POINT('Ctrl Pts',(-0.0564590990687925,0.084884069854931,
-0.738402966137602));
#44911=CARTESIAN_POINT('Ctrl Pts',(-0.0826064778357426,0.0597419869303427,
-0.736293745798978));
#44912=CARTESIAN_POINT('Ctrl Pts',(-0.0922735175391629,0.0293567046619034,
-0.734184525460354));
#44913=CARTESIAN_POINT('Ctrl Pts',(-0.0952693203446887,0.0199403459151532,
-0.733530880869892));
#44914=CARTESIAN_POINT('Ctrl Pts',(-0.0966823977057856,0.0100204450398257,
-0.73287723627943));
#44915=CARTESIAN_POINT('Ctrl Pts',(-0.0966049344323358,7.90599391692882E-5,
-0.732223591688968));
#44916=CARTESIAN_POINT('Origin',(0.,0.,-0.493));
#44917=CARTESIAN_POINT('',(-0.09655822028916,-5.94095412307302E-5,-0.686426408311032));
#44918=CARTESIAN_POINT('',(-0.0965617881854164,-6.15864372647569E-5,-0.692223591688968));
#44919=CARTESIAN_POINT('',(-0.096675,-1.1839272930757E-17,-0.493));
#44920=CARTESIAN_POINT('Ctrl Pts',(-0.09655822028916,-5.94095412307302E-5,
-0.686426408311032));
#44921=CARTESIAN_POINT('Ctrl Pts',(-0.096444469996802,0.0200326449855016,
-0.687745848440121));
#44922=CARTESIAN_POINT('Ctrl Pts',(-0.0903271586571913,0.0401881545090195,
-0.689065288569211));
#44923=CARTESIAN_POINT('Ctrl Pts',(-0.0787087709636884,0.0564016653959087,
-0.6903847286983));
#44924=CARTESIAN_POINT('Ctrl Pts',(-0.0601359391353336,0.0823201335167296,
-0.692493949036924));
#44925=CARTESIAN_POINT('Ctrl Pts',(-0.0275054744417361,0.0981650876515461,
-0.694603169375547));
#44926=CARTESIAN_POINT('Ctrl Pts',(0.00434835961377499,0.0967331910706748,
-0.696712389714171));
#44927=CARTESIAN_POINT('Ctrl Pts',(0.0362021936692865,0.0953012944898034,
-0.698821610052795));
#44928=CARTESIAN_POINT('Ctrl Pts',(0.0672793970867115,0.076592547193244,
-0.70093083039142));
#44929=CARTESIAN_POINT('Ctrl Pts',(0.0834518405620545,0.0491122061493044,
-0.703040050730044));
#44930=CARTESIAN_POINT('Ctrl Pts',(0.0996242840373975,0.0216318651053648,
-0.705149271068668));
#44931=CARTESIAN_POINT('Ctrl Pts',(0.100891967570659,-0.0146200696859549,
-0.707258491407292));
#44932=CARTESIAN_POINT('Ctrl Pts',(0.0866785845800015,-0.0431629639998695,
-0.709367711745916));
#44933=CARTESIAN_POINT('Ctrl Pts',(0.0724652015893446,-0.0717058583137836,
-0.71147693208454));
#44934=CARTESIAN_POINT('Ctrl Pts',(0.0427707520747702,-0.0925397121502928,
-0.713586152423164));
#44935=CARTESIAN_POINT('Ctrl Pts',(0.0110947461665166,-0.0961931655241,
-0.715695372761788));
#44936=CARTESIAN_POINT('Ctrl Pts',(-0.0205812597417374,-0.0998466188979071,
-0.717804593100411));
#44937=CARTESIAN_POINT('Ctrl Pts',(-0.0542388220436707,-0.0863196718090117,
-0.719913813439035));
#44938=CARTESIAN_POINT('Ctrl Pts',(-0.0745767443648309,-0.0617618627146946,
-0.722023033777659));
#44939=CARTESIAN_POINT('Ctrl Pts',(-0.0887297606193485,-0.0446722571100165,
-0.723490825288783));
#44940=CARTESIAN_POINT('Ctrl Pts',(-0.0964325152694136,-0.0222407694604564,
-0.724958616799908));
#44941=CARTESIAN_POINT('Ctrl Pts',(-0.096609779660466,8.02748517758078E-5,
-0.726426408311033));
#44942=CARTESIAN_POINT('Ctrl Pts',(-0.0966049344323358,7.90599391692882E-5,
-0.732223591688968));
#44943=CARTESIAN_POINT('Ctrl Pts',(-0.0964324344776936,-0.0220590243757753,
-0.730768015940806));
#44944=CARTESIAN_POINT('Ctrl Pts',(-0.0888684767602903,-0.0443036470435852,
-0.729312440192644));
#44945=CARTESIAN_POINT('Ctrl Pts',(-0.0749310401969944,-0.0613315364445268,
-0.727856864444482));
#44946=CARTESIAN_POINT('Ctrl Pts',(-0.0547348225115145,-0.0860060136702274,
-0.725747644105858));
#44947=CARTESIAN_POINT('Ctrl Pts',(-0.0211556865006636,-0.0997264865093382,
-0.723638423767234));
#44948=CARTESIAN_POINT('Ctrl Pts',(0.0105408251448544,-0.0962554370044433,
-0.72152920342861));
#44949=CARTESIAN_POINT('Ctrl Pts',(0.0422373367903726,-0.0927843874995483,
-0.719419983089986));
#44950=CARTESIAN_POINT('Ctrl Pts',(0.0720512240705579,-0.0721218156506473,
-0.717310762751361));
#44951=CARTESIAN_POINT('Ctrl Pts',(0.0864286787841937,-0.0436612142670213,
-0.715201542412737));
#44952=CARTESIAN_POINT('Ctrl Pts',(0.100806133497829,-0.0152006128833955,
-0.713092322074114));
#44953=CARTESIAN_POINT('Ctrl Pts',(0.0997471556449157,0.0210580180349552,
-0.71098310173549));
#44954=CARTESIAN_POINT('Ctrl Pts',(0.0837331712995902,0.0486310001106758,
-0.708873881396866));
#44955=CARTESIAN_POINT('Ctrl Pts',(0.0677191869542648,0.0762039821863965,
-0.706764661058242));
#44956=CARTESIAN_POINT('Ctrl Pts',(0.0367501961165274,0.0950913154194871,
-0.704655440719617));
#44957=CARTESIAN_POINT('Ctrl Pts',(0.0049051331451982,0.0967065551887728,
-0.702546220380993));
#44958=CARTESIAN_POINT('Ctrl Pts',(-0.0269399298261309,0.0983217949580586,
-0.700437000042369));
#44959=CARTESIAN_POINT('Ctrl Pts',(-0.0596610649310518,0.0826649412635394,
-0.698327779703746));
#44960=CARTESIAN_POINT('Ctrl Pts',(-0.078382788635008,0.056853817756164,
-0.696218559365122));
#44961=CARTESIAN_POINT('Ctrl Pts',(-0.0902027456225251,0.0405579694421437,
-0.694886903473071));
#44962=CARTESIAN_POINT('Ctrl Pts',(-0.0964425008026231,0.0202146027618285,
-0.693555247581019));
#44963=CARTESIAN_POINT('Ctrl Pts',(-0.0965617881854164,-6.15864372647569E-5,
-0.692223591688968));
#44964=CARTESIAN_POINT('Origin',(0.,0.,-0.493));
#44965=CARTESIAN_POINT('',(-0.0968190249341983,-3.03081917537168E-5,-0.646426408311032));
#44966=CARTESIAN_POINT('',(-0.0968213716511174,-2.71350648972155E-5,-0.652223591688967));
#44967=CARTESIAN_POINT('',(-0.096675,-1.1839272930757E-17,-0.493));
#44968=CARTESIAN_POINT('Ctrl Pts',(-0.0968190249341983,-3.03081917537168E-5,
-0.646426408311032));
#44969=CARTESIAN_POINT('Ctrl Pts',(-0.0966942363656106,0.0301759440623484,
-0.648423859741711));
#44970=CARTESIAN_POINT('Ctrl Pts',(-0.0814178221682262,0.0604911215757958,
-0.65042131117239));
#44971=CARTESIAN_POINT('Ctrl Pts',(-0.0570098021767794,0.0782694125556777,
-0.652418762603068));
#44972=CARTESIAN_POINT('Ctrl Pts',(-0.0312360129367518,0.0970425012750384,
-0.654527982941692));
#44973=CARTESIAN_POINT('Ctrl Pts',(0.00471990542191003,0.10183642791609,
-0.656637203280316));
#44974=CARTESIAN_POINT('Ctrl Pts',(0.034511891865597,0.0904718066908345,
-0.65874642361894));
#44975=CARTESIAN_POINT('Ctrl Pts',(0.0643038783092844,0.079107185465579,
-0.660855643957563));
#44976=CARTESIAN_POINT('Ctrl Pts',(0.087931932837997,0.051584016374016,
-0.662964864296188));
#44977=CARTESIAN_POINT('Ctrl Pts',(0.0946544129332718,0.0204147152393576,
-0.665074084634812));
#44978=CARTESIAN_POINT('Ctrl Pts',(0.101376893028546,-0.0107545858953003,
-0.667183304973436));
#44979=CARTESIAN_POINT('Ctrl Pts',(0.0911937986903842,-0.0455700190730532,
-0.66929252531206));
#44980=CARTESIAN_POINT('Ctrl Pts',(0.068734506365305,-0.0682040037004004,
-0.671401745650684));
#44981=CARTESIAN_POINT('Ctrl Pts',(0.0462752140402253,-0.0908379883277482,
-0.673510965989308));
#44982=CARTESIAN_POINT('Ctrl Pts',(0.0115397237282281,-0.101290524404689,
-0.675620186327932));
#44983=CARTESIAN_POINT('Ctrl Pts',(-0.0196807271168537,-0.0948097435193152,
-0.677729406666556));
#44984=CARTESIAN_POINT('Ctrl Pts',(-0.0509011779619347,-0.0883289626339413,
-0.67983862700518));
#44985=CARTESIAN_POINT('Ctrl Pts',(-0.0786065893401007,-0.0649148647862529,
-0.681947847343803));
#44986=CARTESIAN_POINT('Ctrl Pts',(-0.0902016955476279,-0.035211824808996,
-0.684057067682427));
#44987=CARTESIAN_POINT('Ctrl Pts',(-0.0945433877086917,-0.0240897657678029,
-0.684846847891962));
#44988=CARTESIAN_POINT('Ctrl Pts',(-0.0966263080543815,-0.0120859552588177,
-0.685636628101497));
#44989=CARTESIAN_POINT('Ctrl Pts',(-0.09655822028916,-5.94095412307302E-5,
-0.686426408311032));
#44990=CARTESIAN_POINT('Ctrl Pts',(-0.0965617881854164,-6.15864372647569E-5,
-0.692223591688968));
#44991=CARTESIAN_POINT('Ctrl Pts',(-0.0966314410351792,-0.0119010142709122,
-0.691446027242395));
#44992=CARTESIAN_POINT('Ctrl Pts',(-0.0946143296894111,-0.0237175380444123,
-0.690668462795823));
#44993=CARTESIAN_POINT('Ctrl Pts',(-0.0904028966310228,-0.03469199372149,
-0.68989089834925));
#44994=CARTESIAN_POINT('Ctrl Pts',(-0.0789789686200898,-0.0644612883715367,
-0.687781678010626));
#44995=CARTESIAN_POINT('Ctrl Pts',(-0.0514088002952321,-0.0880344843513981,
-0.685672457672002));
#44996=CARTESIAN_POINT('Ctrl Pts',(-0.0202261739853999,-0.0946948786026133,
-0.683563237333378));
#44997=CARTESIAN_POINT('Ctrl Pts',(0.0109564523244319,-0.101355272853828,
-0.681454016994754));
#44998=CARTESIAN_POINT('Ctrl Pts',(0.0457515366192382,-0.091102865376398,
-0.679344796656129));
#44999=CARTESIAN_POINT('Ctrl Pts',(0.0683407491909844,-0.0685985433348721,
-0.677235576317506));
#45000=CARTESIAN_POINT('Ctrl Pts',(0.0909299617627307,-0.046094221293346,
-0.675126355978882));
#45001=CARTESIAN_POINT('Ctrl Pts',(0.101313302611417,-0.0113379846877243,
-0.673017135640258));
#45002=CARTESIAN_POINT('Ctrl Pts',(0.0947703604391765,0.0198694974742666,
-0.670907915301634));
#45003=CARTESIAN_POINT('Ctrl Pts',(0.0882274182669362,0.0510769796362577,
-0.66879869496301));
#45004=CARTESIAN_POINT('Ctrl Pts',(0.0647581930737698,0.0787357073546175,
-0.666689474624386));
#45005=CARTESIAN_POINT('Ctrl Pts',(0.0350321213511129,0.090271637967261,
-0.664580254285762));
#45006=CARTESIAN_POINT('Ctrl Pts',(0.00530604962845649,0.101807568579904,
-0.662471033947138));
#45007=CARTESIAN_POINT('Ctrl Pts',(-0.03067686862369,0.0972207020868314,
-0.660361813608514));
#45008=CARTESIAN_POINT('Ctrl Pts',(-0.0565582978442699,0.0785962918502532,
-0.65825259326989));
#45009=CARTESIAN_POINT('Ctrl Pts',(-0.0812181488217498,0.0608509356311975,
-0.656242926076249));
#45010=CARTESIAN_POINT('Ctrl Pts',(-0.0967075680763441,0.0303618803342572,
-0.654233258882608));
#45011=CARTESIAN_POINT('Ctrl Pts',(-0.0968213716511174,-2.71350648972155E-5,
-0.652223591688967));
#45012=CARTESIAN_POINT('Origin',(0.,0.,-0.493));
#45013=CARTESIAN_POINT('',(-0.0966413181482248,8.54984747835699E-5,-0.606426408311032));
#45014=CARTESIAN_POINT('',(-0.0966360180667763,8.49218538845601E-5,-0.612223591688967));
#45015=CARTESIAN_POINT('',(-0.096675,-1.1839272930757E-17,-0.493));
#45016=CARTESIAN_POINT('Ctrl Pts',(-0.0966413181482248,8.54984747835699E-5,
-0.606426408311032));
#45017=CARTESIAN_POINT('Ctrl Pts',(-0.0967160133304872,0.0086893470084329,
-0.606992650704676));
#45018=CARTESIAN_POINT('Ctrl Pts',(-0.0956611835672563,0.0172751935884665,
-0.60755889309832));
#45019=CARTESIAN_POINT('Ctrl Pts',(-0.0934040461356575,0.0255323843683732,
-0.608125135491964));
#45020=CARTESIAN_POINT('Ctrl Pts',(-0.0849963390631441,0.0562899449614566,
-0.610234355830588));
#45021=CARTESIAN_POINT('Ctrl Pts',(-0.0599063769810964,0.0824873417858737,
-0.612343576169212));
#45022=CARTESIAN_POINT('Ctrl Pts',(-0.0295404059331587,0.0922148735473329,
-0.614452796507836));
#45023=CARTESIAN_POINT('Ctrl Pts',(0.000825565114778395,0.101942405308792,
-0.61656201684646));
#45024=CARTESIAN_POINT('Ctrl Pts',(0.0364675451286056,0.0952000720072934,
-0.618671237185084));
#45025=CARTESIAN_POINT('Ctrl Pts',(0.0611821938166583,0.0750530322227374,
-0.620780457523708));
#45026=CARTESIAN_POINT('Ctrl Pts',(0.0858968425047111,0.0549059924381812,
-0.622889677862332));
#45027=CARTESIAN_POINT('Ctrl Pts',(0.0996841598669897,0.0213542461705674,
-0.624998898200956));
#45028=CARTESIAN_POINT('Ctrl Pts',(0.0962762394952784,-0.010349115647928,
-0.62710811853958));
#45029=CARTESIAN_POINT('Ctrl Pts',(0.0928683191235671,-0.042052477466424,
-0.629217338878204));
#45030=CARTESIAN_POINT('Ctrl Pts',(0.0722651610178653,-0.0719074548358012,
-0.631326559216828));
#45031=CARTESIAN_POINT('Ctrl Pts',(0.0438332476726959,-0.086341559428299,
-0.633435779555452));
#45032=CARTESIAN_POINT('Ctrl Pts',(0.0154013343275267,-0.100775664020797,
-0.635544999894076));
#45033=CARTESIAN_POINT('Ctrl Pts',(-0.0208593342571104,-0.0997888958364151,
-0.6376542202327));
#45034=CARTESIAN_POINT('Ctrl Pts',(-0.0484641533524033,-0.0838298534287226,
-0.639763440571324));
#45035=CARTESIAN_POINT('Ctrl Pts',(-0.0760689724476961,-0.0678708110210303,
-0.641872660909948));
#45036=CARTESIAN_POINT('Ctrl Pts',(-0.0950179420536452,-0.0369394943900277,
-0.643981881248572));
#45037=CARTESIAN_POINT('Ctrl Pts',(-0.0966965967959232,-0.00509771067569107,
-0.646091101587196));
#45038=CARTESIAN_POINT('Ctrl Pts',(-0.0967855497630107,-0.00341039459608733,
-0.646202870495141));
#45039=CARTESIAN_POINT('Ctrl Pts',(-0.0968260075730854,-0.00172052191896296,
-0.646314639403087));
#45040=CARTESIAN_POINT('Ctrl Pts',(-0.0968190249341983,-3.03081917537168E-5,
-0.646426408311032));
#45041=CARTESIAN_POINT('Ctrl Pts',(-0.0968213716511174,-2.71350648972155E-5,
-0.652223591688967));
#45042=CARTESIAN_POINT('Ctrl Pts',(-0.0968270091535929,-0.00153251967061721,
-0.652124038543984));
#45043=CARTESIAN_POINT('Ctrl Pts',(-0.0967949160138212,-0.00303765878570629,
-0.652024485399001));
#45044=CARTESIAN_POINT('Ctrl Pts',(-0.0967243379264574,-0.00454099111866625,
-0.651924932254018));
#45045=CARTESIAN_POINT('Ctrl Pts',(-0.0952290085990514,-0.0363919098709228,
-0.649815711915394));
#45046=CARTESIAN_POINT('Ctrl Pts',(-0.0764584097552263,-0.0674317933953525,
-0.64770649157677));
#45047=CARTESIAN_POINT('Ctrl Pts',(-0.0489459169377222,-0.0835494785308498,
-0.645597271238146));
#45048=CARTESIAN_POINT('Ctrl Pts',(-0.0214334241202177,-0.0996671636663474,
-0.643488050899522));
#45049=CARTESIAN_POINT('Ctrl Pts',(0.0148209626709659,-0.100862650412913,
-0.641378830560898));
#45050=CARTESIAN_POINT('Ctrl Pts',(0.0433354944977714,-0.0865924538530059,
-0.639269610222274));
#45051=CARTESIAN_POINT('Ctrl Pts',(0.0718500263245767,-0.0723222572930992,
-0.63716038988365));
#45052=CARTESIAN_POINT('Ctrl Pts',(0.0926247031870034,-0.0425863774267208,
-0.635051169545026));
#45053=CARTESIAN_POINT('Ctrl Pts',(0.0962150677759835,-0.0109031591987936,
-0.632941949206402));
#45054=CARTESIAN_POINT('Ctrl Pts',(0.0998054323649636,0.0207800590291337,
-0.630832728867778));
#45055=CARTESIAN_POINT('Ctrl Pts',(0.0862114846804966,0.0544106156186099,
-0.628723508529154));
#45056=CARTESIAN_POINT('Ctrl Pts',(0.0616132225833369,0.074699591368009,
-0.62661428819053));
#45057=CARTESIAN_POINT('Ctrl Pts',(0.0370149604861774,0.0949885671174079,
-0.624505067851906));
#45058=CARTESIAN_POINT('Ctrl Pts',(0.00141238397632584,0.10193596202673,
-0.622395847513282));
#45059=CARTESIAN_POINT('Ctrl Pts',(-0.0290090800360038,0.0923833936544662,
-0.620286627174659));
#45060=CARTESIAN_POINT('Ctrl Pts',(-0.0594305440483332,0.0828308252822022,
-0.618177406836035));
#45061=CARTESIAN_POINT('Ctrl Pts',(-0.0846708955631408,0.0567782936283514,
-0.61606818649741));
#45062=CARTESIAN_POINT('Ctrl Pts',(-0.0932555194070551,0.0260696422639763,
-0.613958966158786));
#45063=CARTESIAN_POINT('Ctrl Pts',(-0.0956098707249212,0.0176477294202516,
-0.61338050800218));
#45064=CARTESIAN_POINT('Ctrl Pts',(-0.0967114743576563,0.00887561013077407,
-0.612802049845574));
#45065=CARTESIAN_POINT('Ctrl Pts',(-0.0966360180667763,8.49218538845601E-5,
-0.612223591688967));
#45066=CARTESIAN_POINT('Origin',(0.,0.,-0.493));
#45067=CARTESIAN_POINT('',(-0.0965393946746019,-4.45580922561403E-5,-0.566426408311032));
#45068=CARTESIAN_POINT('',(-0.0965420680789469,-4.71254655582805E-5,-0.572223591688968));
#45069=CARTESIAN_POINT('',(-0.096675,-1.1839272930757E-17,-0.493));
#45070=CARTESIAN_POINT('Ctrl Pts',(-0.0965393946746019,-4.45580922561403E-5,
-0.566426408311032));
#45071=CARTESIAN_POINT('Ctrl Pts',(-0.0964598943699223,0.0189118469550805,
-0.567670662006265));
#45072=CARTESIAN_POINT('Ctrl Pts',(-0.0910651542801533,0.0379100173100681,
-0.568914915701499));
#45073=CARTESIAN_POINT('Ctrl Pts',(-0.0806573094966741,0.0535781383663534,
-0.570159169396732));
#45074=CARTESIAN_POINT('Ctrl Pts',(-0.0630142532753806,0.0801382520526055,
-0.572268389735356));
#45075=CARTESIAN_POINT('Ctrl Pts',(-0.030965549107614,0.097129142518426,
-0.57437761007398));
#45076=CARTESIAN_POINT('Ctrl Pts',(0.00091901593711588,0.0968265144253046,
-0.576486830412604));
#45077=CARTESIAN_POINT('Ctrl Pts',(0.0328035809818462,0.0965238863321833,
-0.578596050751228));
#45078=CARTESIAN_POINT('Ctrl Pts',(0.0645240069035398,0.0789277396801196,
-0.580705271089852));
#45079=CARTESIAN_POINT('Ctrl Pts',(0.0816597464933621,0.0520375276957528,
-0.582814491428476));
#45080=CARTESIAN_POINT('Ctrl Pts',(0.0987954860831841,0.0251473157113864,
-0.5849237117671));
#45081=CARTESIAN_POINT('Ctrl Pts',(0.101346539341135,-0.0110369616052829,
-0.587032932105724));
#45082=CARTESIAN_POINT('Ctrl Pts',(0.0881531619425538,-0.0400654280593166,
-0.589142152444348));
#45083=CARTESIAN_POINT('Ctrl Pts',(0.0749597845439722,-0.0690938945133507,
-0.591251372782972));
#45084=CARTESIAN_POINT('Ctrl Pts',(0.0460219764888577,-0.090966550104749,
-0.593360593121596));
#45085=CARTESIAN_POINT('Ctrl Pts',(0.0144952681666549,-0.0957397811091249,
-0.59546981346022));
#45086=CARTESIAN_POINT('Ctrl Pts',(-0.0170314401555474,-0.100513012113501,
-0.597579033798844));
#45087=CARTESIAN_POINT('Ctrl Pts',(-0.0511470487448379,-0.0881868185308549,
-0.599688254137468));
#45088=CARTESIAN_POINT('Ctrl Pts',(-0.0723421270079938,-0.0643648595586574,
-0.601797474476092));
#45089=CARTESIAN_POINT('Ctrl Pts',(-0.0878471634915268,-0.0469381561331164,
-0.603340452421072));
#45090=CARTESIAN_POINT('Ctrl Pts',(-0.0964377780740077,-0.0233594937730345,
-0.604883430366052));
#45091=CARTESIAN_POINT('Ctrl Pts',(-0.0966413181482248,8.54984747835699E-5,
-0.606426408311032));
#45092=CARTESIAN_POINT('Ctrl Pts',(-0.0966360180667763,8.49218538845601E-5,
-0.612223591688967));
#45093=CARTESIAN_POINT('Ctrl Pts',(-0.0964363396023009,-0.0231776996762786,
-0.610692829506949));
#45094=CARTESIAN_POINT('Ctrl Pts',(-0.0879939491883497,-0.0465703560596884,
-0.609162067324932));
#45095=CARTESIAN_POINT('Ctrl Pts',(-0.0727114440849164,-0.0639473537117637,
-0.607631305142914));
#45096=CARTESIAN_POINT('Ctrl Pts',(-0.0516538487458423,-0.0878909272482276,
-0.60552208480429));
#45097=CARTESIAN_POINT('Ctrl Pts',(-0.0176097618946735,-0.100413303246256,
-0.603412864465667));
#45098=CARTESIAN_POINT('Ctrl Pts',(0.0139439006531827,-0.0958216352512599,
-0.601303644127043));
#45099=CARTESIAN_POINT('Ctrl Pts',(0.0454975632010391,-0.0912299672562642,
-0.599194423788419));
#45100=CARTESIAN_POINT('Ctrl Pts',(0.0745608014455828,-0.0695242552682441,
-0.597085203449794));
#45101=CARTESIAN_POINT('Ctrl Pts',(0.0879210626871216,-0.0405722181254436,
-0.59497598311117));
#45102=CARTESIAN_POINT('Ctrl Pts',(0.10128132392866,-0.0116201809826433,
-0.592866762772546));
#45103=CARTESIAN_POINT('Ctrl Pts',(0.0989386081671945,0.0245781813149372,
-0.590757542433923));
#45104=CARTESIAN_POINT('Ctrl Pts',(0.0819579466011862,0.0515665893439584,
-0.588648322095299));
#45105=CARTESIAN_POINT('Ctrl Pts',(0.0649772850351777,0.0785549973729798,
-0.586539101756675));
#45106=CARTESIAN_POINT('Ctrl Pts',(0.033358677664626,0.0963334511334416,
-0.58442988141805));
#45107=CARTESIAN_POINT('Ctrl Pts',(0.00147638356758545,0.0968196180493019,
-0.582320661079426));
#45108=CARTESIAN_POINT('Ctrl Pts',(-0.0304059105294553,0.0973057849651621,
-0.580211440740802));
#45109=CARTESIAN_POINT('Ctrl Pts',(-0.0625518913529849,0.080499665036421,
-0.578102220402179));
#45110=CARTESIAN_POINT('Ctrl Pts',(-0.0803475485115806,0.0540415543432139,
-0.575993000063555));
#45111=CARTESIAN_POINT('Ctrl Pts',(-0.0909484797176978,0.0382803712184285,
-0.574736530605359));
#45112=CARTESIAN_POINT('Ctrl Pts',(-0.096457020786623,0.0190940595933471,
-0.573480061147164));
#45113=CARTESIAN_POINT('Ctrl Pts',(-0.0965420680789469,-4.71254655582805E-5,
-0.572223591688968));
#45114=CARTESIAN_POINT('Origin',(0.,0.,-0.493));
#45115=CARTESIAN_POINT('',(-0.0967998842052739,-4.85300446802506E-5,-0.526426408311032));
#45116=CARTESIAN_POINT('',(-0.0968034943207674,-4.57450494820897E-5,-0.532223591688968));
#45117=CARTESIAN_POINT('',(-0.096675,-1.1839272930757E-17,-0.493));
#45118=CARTESIAN_POINT('Ctrl Pts',(-0.0967998842052739,-4.85300446802506E-5,
-0.526426408311032));
#45119=CARTESIAN_POINT('Ctrl Pts',(-0.0966204449976918,0.0290359816449859,
-0.528348673307855));
#45120=CARTESIAN_POINT('Ctrl Pts',(-0.0826150578079472,0.058270385292619,
-0.530270938304678));
#45121=CARTESIAN_POINT('Ctrl Pts',(-0.0597465881474668,0.0762008116149912,
-0.5321932033015));
#45122=CARTESIAN_POINT('Ctrl Pts',(-0.034653980520104,0.095875112474578,
-0.534302423640124));
#45123=CARTESIAN_POINT('Ctrl Pts',(0.00110955476683836,0.101939709858917,
-0.536411643978749));
#45124=CARTESIAN_POINT('Ctrl Pts',(0.0312854167023489,0.0916375533709122,
-0.538520864317373));
#45125=CARTESIAN_POINT('Ctrl Pts',(0.0614612786378607,0.0813353968829074,
-0.540630084655997));
#45126=CARTESIAN_POINT('Ctrl Pts',(0.0860494672219405,0.0546664865225578,
-0.54273930499462));
#45127=CARTESIAN_POINT('Ctrl Pts',(0.093871849628384,0.0237548802016017,
-0.544848525333244));
#45128=CARTESIAN_POINT('Ctrl Pts',(0.101694232034827,-0.0071567261193535,
-0.546957745671868));
#45129=CARTESIAN_POINT('Ctrl Pts',(0.0927508082636355,-0.0423110284009153,
-0.549066966010493));
#45130=CARTESIAN_POINT('Ctrl Pts',(0.0711073832639433,-0.0657263914375426,
-0.551176186349117));
#45131=CARTESIAN_POINT('Ctrl Pts',(0.0494639582642506,-0.0891417544741703,
-0.553285406687741));
#45132=CARTESIAN_POINT('Ctrl Pts',(0.0151205320360575,-0.100818178265863,
-0.555394627026364));
#45133=CARTESIAN_POINT('Ctrl Pts',(-0.0163098957572849,-0.0954473980076612,
-0.557503847364988));
#45134=CARTESIAN_POINT('Ctrl Pts',(-0.0477403235506265,-0.0900766177494595,
-0.559613067703612));
#45135=CARTESIAN_POINT('Ctrl Pts',(-0.0762577529091172,-0.0676586334413634,
-0.561722288042237));
#45136=CARTESIAN_POINT('Ctrl Pts',(-0.0888977634509525,-0.0383849728339736,
-0.563831508380861));
#45137=CARTESIAN_POINT('Ctrl Pts',(-0.0940812842479904,-0.0263801862824427,
-0.564696475024251));
#45138=CARTESIAN_POINT('Ctrl Pts',(-0.0965946608248659,-0.0132224639384352,
-0.565561441667642));
#45139=CARTESIAN_POINT('Ctrl Pts',(-0.0965393946746019,-4.45580922561403E-5,
-0.566426408311032));
#45140=CARTESIAN_POINT('Ctrl Pts',(-0.0965420680789469,-4.71254655582805E-5,
-0.572223591688968));
#45141=CARTESIAN_POINT('Ctrl Pts',(-0.0965997886649382,-0.0130380201546043,
-0.571370840808539));
#45142=CARTESIAN_POINT('Ctrl Pts',(-0.0941593528399191,-0.0260081287553386,
-0.570518089928111));
#45143=CARTESIAN_POINT('Ctrl Pts',(-0.0891172524233399,-0.0378725952129777,
-0.569665339047682));
#45144=CARTESIAN_POINT('Ctrl Pts',(-0.076645965682842,-0.0672185326182907,
-0.567556118709058));
#45145=CARTESIAN_POINT('Ctrl Pts',(-0.0482580587081843,-0.0898003059712441,
-0.565446898370435));
#45146=CARTESIAN_POINT('Ctrl Pts',(-0.0168590692023799,-0.0953519267413129,
-0.563337678031811));
#45147=CARTESIAN_POINT('Ctrl Pts',(0.014539920303424,-0.100903547511382,
-0.561228457693187));
#45148=CARTESIAN_POINT('Ctrl Pts',(0.0489499923403744,-0.0894250156985665,
-0.559119237354563));
#45149=CARTESIAN_POINT('Ctrl Pts',(0.0707278491326723,-0.0661346316593453,
-0.557010017015939));
#45150=CARTESIAN_POINT('Ctrl Pts',(0.0925057059249705,-0.0428442476201238,
-0.554900796677315));
#45151=CARTESIAN_POINT('Ctrl Pts',(0.101651347472616,-0.00774201135449594,
-0.552791576338691));
#45152=CARTESIAN_POINT('Ctrl Pts',(0.0940070378101934,0.0232141118676594,
-0.550682356000067));
#45153=CARTESIAN_POINT('Ctrl Pts',(0.0863627281477711,0.0541702350898143,
-0.548573135661443));
#45154=CARTESIAN_POINT('Ctrl Pts',(0.0619284672752818,0.0809802452684969,
-0.546463915322819));
#45155=CARTESIAN_POINT('Ctrl Pts',(0.031812410338389,0.0914559385502838,
-0.544354694984195));
#45156=CARTESIAN_POINT('Ctrl Pts',(0.00169635340149625,0.101931631832071,
-0.542245474645571));
#45157=CARTESIAN_POINT('Ctrl Pts',(-0.0341014995998,0.0960730082169618,
-0.540136254306947));
#45158=CARTESIAN_POINT('Ctrl Pts',(-0.059306946343801,0.0765434795591685,
-0.538027033968323));
#45159=CARTESIAN_POINT('Ctrl Pts',(-0.0824242332745107,0.0586318859980991,
-0.536092553208537));
#45160=CARTESIAN_POINT('Ctrl Pts',(-0.0966314821794818,0.0292207067132771,
-0.534158072448753));
#45161=CARTESIAN_POINT('Ctrl Pts',(-0.0968034943207674,-4.57450494820897E-5,
-0.532223591688968));
#45162=CARTESIAN_POINT('Origin',(0.,0.,-0.493));
#45163=CARTESIAN_POINT('',(-0.0966749003444729,8.66157029079558E-5,-0.486426408311032));
#45164=CARTESIAN_POINT('',(-0.096669360704088,8.67233818675543E-5,-0.492223591688967));
#45165=CARTESIAN_POINT('',(-0.096675,-1.1839272930757E-17,-0.493));
#45166=CARTESIAN_POINT('Ctrl Pts',(-0.0966749003444729,8.66157029079557E-5,
-0.486426408311032));
#45167=CARTESIAN_POINT('Ctrl Pts',(-0.0967425505848559,0.00754142010055274,
-0.48691746427082));
#45168=CARTESIAN_POINT('Ctrl Pts',(-0.0959524121396197,0.0149820405673192,
-0.487408520230609));
#45169=CARTESIAN_POINT('Ctrl Pts',(-0.0942498682055356,0.0222076750085543,
-0.487899576190397));
#45170=CARTESIAN_POINT('Ctrl Pts',(-0.0869369739791434,0.0532437612613018,
-0.490008796529021));
#45171=CARTESIAN_POINT('Ctrl Pts',(-0.0627907582739773,0.0803134872439226,
-0.492118016867645));
#45172=CARTESIAN_POINT('Ctrl Pts',(-0.0327884268927159,0.0911105786829796,
-0.494227237206269));
#45173=CARTESIAN_POINT('Ctrl Pts',(-0.00278609551145491,0.101907670122036,
-0.496336457544893));
#45174=CARTESIAN_POINT('Ctrl Pts',(0.0330723515459016,0.09643212701753,
-0.498445677883517));
#45175=CARTESIAN_POINT('Ctrl Pts',(0.0584851650562304,0.0771732074906303,
-0.500554898222141));
#45176=CARTESIAN_POINT('Ctrl Pts',(0.0838979785665599,0.05791428796373,
-0.502664118560765));
#45177=CARTESIAN_POINT('Ctrl Pts',(0.0988651585298612,0.0248719920144367,
-0.504773338899389));
#45178=CARTESIAN_POINT('Ctrl Pts',(0.0965824165744489,-0.00693219263191769,
-0.506882559238013));
#45179=CARTESIAN_POINT('Ctrl Pts',(0.0942996746190366,-0.0387363772782712,
-0.508991779576637));
#45180=CARTESIAN_POINT('Ctrl Pts',(0.0747670107449108,-0.0693024506216854,
-0.511100999915261));
#45181=CARTESIAN_POINT('Ctrl Pts',(0.0468642458664085,-0.0847346502053275,
-0.513210220253885));
#45182=CARTESIAN_POINT('Ctrl Pts',(0.0189614809879057,-0.10016684978897,
-0.515319440592508));
#45183=CARTESIAN_POINT('Ctrl Pts',(-0.0173113848949743,-0.10046517561284,
-0.517428660931132));
#45184=CARTESIAN_POINT('Ctrl Pts',(-0.0454642019918381,-0.0854940046043682,
-0.519537881269756));
#45185=CARTESIAN_POINT('Ctrl Pts',(-0.0736170190887016,-0.0705228335958964,
-0.52164710160838));
#45186=CARTESIAN_POINT('Ctrl Pts',(-0.0936497873995494,-0.0402821657550826,
-0.523756321947005));
#45187=CARTESIAN_POINT('Ctrl Pts',(-0.0964553315710817,-0.00851982966725782,
-0.525865542285629));
#45188=CARTESIAN_POINT('Ctrl Pts',(-0.0967040070934641,-0.00570450578147726,
-0.52605249762743));
#45189=CARTESIAN_POINT('Ctrl Pts',(-0.0968173360750429,-0.00287722683364963,
-0.526239452969231));
#45190=CARTESIAN_POINT('Ctrl Pts',(-0.0967998842052739,-4.85300446802506E-5,
-0.526426408311032));
#45191=CARTESIAN_POINT('Ctrl Pts',(-0.0968034943207674,-4.57450494820897E-5,
-0.532223591688968));
#45192=CARTESIAN_POINT('Ctrl Pts',(-0.0968190319935881,-0.00268935234785623,
-0.532048852110129));
#45193=CARTESIAN_POINT('Ctrl Pts',(-0.0967200517379734,-0.00533177876867958,
-0.53187411253129));
#45194=CARTESIAN_POINT('Ctrl Pts',(-0.0965027761683216,-0.00796444219378559,
-0.531699372952451));
#45195=CARTESIAN_POINT('Ctrl Pts',(-0.0938801187621351,-0.0397424015884674,
-0.529590152613827));
#45196=CARTESIAN_POINT('Ctrl Pts',(-0.0740217634630564,-0.0700978866773524,
-0.527480932275203));
#45197=CARTESIAN_POINT('Ctrl Pts',(-0.0459555950412053,-0.0852308713557481,
-0.525371711936579));
#45198=CARTESIAN_POINT('Ctrl Pts',(-0.0178894266193546,-0.100363856034144,
-0.523262491597955));
#45199=CARTESIAN_POINT('Ctrl Pts',(0.0183845549252683,-0.10027434030205,
-0.521153271259331));
#45200=CARTESIAN_POINT('Ctrl Pts',(0.046375692606911,-0.0850030192574396,
-0.519044050920707));
#45201=CARTESIAN_POINT('Ctrl Pts',(0.074366830288554,-0.0697316982128287,
-0.516934830582083));
#45202=CARTESIAN_POINT('Ctrl Pts',(0.0940751241072166,-0.0392785718557001,
-0.514825610243459));
#45203=CARTESIAN_POINT('Ctrl Pts',(0.0965409093308046,-0.00748805537056879,
-0.512716389904835));
#45204=CARTESIAN_POINT('Ctrl Pts',(0.0990066945543925,0.0243024611145621,
-0.510607169566211));
#45205=CARTESIAN_POINT('Ctrl Pts',(0.0842299711829063,0.0574303677276956,
-0.508497949227587));
#45206=CARTESIAN_POINT('Ctrl Pts',(0.0589284433700178,0.0768352569439182,
-0.506388728888963));
#45207=CARTESIAN_POINT('Ctrl Pts',(0.0336269155571289,0.096240146160141,
-0.504279508550339));
#45208=CARTESIAN_POINT('Ctrl Pts',(-0.00219941669716259,0.101922017979453,
-0.502170288211715));
#45209=CARTESIAN_POINT('Ctrl Pts',(-0.032263404006282,0.0912978143745992,
-0.500061067873091));
#45210=CARTESIAN_POINT('Ctrl Pts',(-0.0623273913154009,0.080673610769746,
-0.497951847534467));
#45211=CARTESIAN_POINT('Ctrl Pts',(-0.0866290336793479,0.0537433317407283,
-0.495842627195843));
#45212=CARTESIAN_POINT('Ctrl Pts',(-0.0941204661726449,0.0227498570346129,
-0.493733406857219));
#45213=CARTESIAN_POINT('Ctrl Pts',(-0.095907963698499,0.0153546413126034,
-0.493230135134469));
#45214=CARTESIAN_POINT('Ctrl Pts',(-0.0967384119606225,0.00772809722163936,
-0.492726863411718));
#45215=CARTESIAN_POINT('Ctrl Pts',(-0.096669360704088,8.67233818675543E-5,
-0.492223591688967));
#45216=CARTESIAN_POINT('Origin',(0.,0.,-0.493));
#45217=CARTESIAN_POINT('',(-0.096526423484871,-2.77199618692811E-5,-0.446426408311032));
#45218=CARTESIAN_POINT('',(-0.0965281097149038,-3.05597964714245E-5,-0.452223591688967));
#45219=CARTESIAN_POINT('',(-0.096675,-1.1839272930757E-17,-0.493));
#45220=CARTESIAN_POINT('Ctrl Pts',(-0.096526423484871,-2.77199618692811E-5,
-0.446426408311032));
#45221=CARTESIAN_POINT('Ctrl Pts',(-0.0964803188479194,0.017789197404952,
-0.44759547557241));
#45222=CARTESIAN_POINT('Ctrl Pts',(-0.0917559201737887,0.0356288516457462,
-0.448764542833788));
#45223=CARTESIAN_POINT('Ctrl Pts',(-0.0825046063050242,0.0506873596126229,
-0.449933610095166));
#45224=CARTESIAN_POINT('Ctrl Pts',(-0.0658134714014635,0.0778557803890599,
-0.45204283043379));
#45225=CARTESIAN_POINT('Ctrl Pts',(-0.0343867555591216,0.0959712800790841,
-0.454152050772413));
#45226=CARTESIAN_POINT('Ctrl Pts',(-0.00251148129597715,0.0967983003350077,
-0.456261271111037));
#45227=CARTESIAN_POINT('Ctrl Pts',(0.0293637929671665,0.0976253205909313,
-0.458370491449661));
#45228=CARTESIAN_POINT('Ctrl Pts',(0.0616876256511122,0.0811638614127553,
-0.460479711788285));
#45229=CARTESIAN_POINT('Ctrl Pts',(0.0797651524327904,0.0548975313053337,
-0.462588932126909));
#45230=CARTESIAN_POINT('Ctrl Pts',(0.0978426792144691,0.0286312011979114,
-0.464698152465533));
#45231=CARTESIAN_POINT('Ctrl Pts',(0.101673900093879,-0.00743999983875827,
-0.466807372804157));
#45232=CARTESIAN_POINT('Ctrl Pts',(0.0895170887242362,-0.0369176016607743,
-0.468916593142781));
#45233=CARTESIAN_POINT('Ctrl Pts',(0.0773602773545936,-0.0663952034827903,
-0.471025813481405));
#45234=CARTESIAN_POINT('Ctrl Pts',(0.0492154337359004,-0.0892792060901528,
-0.473135033820029));
#45235=CARTESIAN_POINT('Ctrl Pts',(0.0178775955858247,-0.0951662233259054,
-0.475244254158653));
#45236=CARTESIAN_POINT('Ctrl Pts',(-0.0134602425642505,-0.101053240561658,
-0.477353474497277));
#45237=CARTESIAN_POINT('Ctrl Pts',(-0.0479910752457083,-0.0899432724257991,
-0.479462694835901));
#45238=CARTESIAN_POINT('Ctrl Pts',(-0.0700167052126272,-0.0668870650964328,
-0.481571915174525));
#45239=CARTESIAN_POINT('Ctrl Pts',(-0.0869144608340886,-0.0491986649192516,
-0.483190079553361));
#45240=CARTESIAN_POINT('Ctrl Pts',(-0.096451974205353,-0.0244790141138182,
-0.484808243932196));
#45241=CARTESIAN_POINT('Ctrl Pts',(-0.0966749003444729,8.66157029079557E-5,
-0.486426408311032));
#45242=CARTESIAN_POINT('Ctrl Pts',(-0.096669360704088,8.67233818675543E-5,
-0.492223591688967));
#45243=CARTESIAN_POINT('Ctrl Pts',(-0.0964490169715812,-0.0242970303372613,
-0.490617643073094));
#45244=CARTESIAN_POINT('Ctrl Pts',(-0.0870694389706079,-0.0488317892994789,
-0.489011694457221));
#45245=CARTESIAN_POINT('Ctrl Pts',(-0.0704005799644349,-0.0664829037296246,
-0.487405745841347));
#45246=CARTESIAN_POINT('Ctrl Pts',(-0.0485080386402814,-0.0896655194045322,
-0.485296525502723));
#45247=CARTESIAN_POINT('Ctrl Pts',(-0.0140417333693276,-0.100974080371134,
-0.483187305164099));
#45248=CARTESIAN_POINT('Ctrl Pts',(0.017329473661618,-0.0952675573858311,
-0.481078084825475));
#45249=CARTESIAN_POINT('Ctrl Pts',(0.048700680692564,-0.0895610344005279,
-0.478968864486851));
#45250=CARTESIAN_POINT('Ctrl Pts',(0.0769767894835017,-0.0668394274633188,
-0.476859644148227));
#45251=CARTESIAN_POINT('Ctrl Pts',(0.0893030873420965,-0.0374322953987758,
-0.474750423809603));
#45252=CARTESIAN_POINT('Ctrl Pts',(0.101629385200691,-0.00802516333423281,
-0.472641203470979));
#45253=CARTESIAN_POINT('Ctrl Pts',(0.0980058721269431,0.0280674938576442,
-0.470531983132355));
#45254=CARTESIAN_POINT('Ctrl Pts',(0.0800798476076497,0.0544374517661044,
-0.468422762793731));
#45255=CARTESIAN_POINT('Ctrl Pts',(0.0621538230883563,0.0808074096745646,
-0.466313542455107));
#45256=CARTESIAN_POINT('Ctrl Pts',(0.0299252871235178,0.0974546682996081,
-0.464204322116483));
#45257=CARTESIAN_POINT('Ctrl Pts',(-0.00195421917894117,0.0968111521212923,
-0.462095101777859));
#45258=CARTESIAN_POINT('Ctrl Pts',(-0.0338337254813997,0.0961676359429765,
-0.459985881439235));
#45259=CARTESIAN_POINT('Ctrl Pts',(-0.0653642021214785,0.0782333449613021,
-0.457876661100611));
#45260=CARTESIAN_POINT('Ctrl Pts',(-0.0822114554780782,0.0511614575225072,
-0.455767440761987));
#45261=CARTESIAN_POINT('Ctrl Pts',(-0.0916468729318517,0.0359996650427535,
-0.454586157737647));
#45262=CARTESIAN_POINT('Ctrl Pts',(-0.0964766987464544,0.0179717418073378,
-0.453404874713307));
#45263=CARTESIAN_POINT('Ctrl Pts',(-0.0965281097149038,-3.05597964714245E-5,
-0.452223591688967));
#45264=CARTESIAN_POINT('Origin',(0.,0.,-0.493));
#45265=CARTESIAN_POINT('',(-0.0967741445435993,-6.3845289803563E-5,-0.406426408311032));
#45266=CARTESIAN_POINT('',(-0.0967786908216685,-6.15870636970637E-5,-0.412223591688967));
#45267=CARTESIAN_POINT('',(-0.096675,-1.1839272930757E-17,-0.493));
#45268=CARTESIAN_POINT('Ctrl Pts',(-0.0967741445435993,-6.3845289803563E-5,
-0.406426408311032));
#45269=CARTESIAN_POINT('Ctrl Pts',(-0.096560293855864,0.0279026272071614,
-0.408273486873999));
#45270=CARTESIAN_POINT('Ctrl Pts',(-0.0837582806333823,0.0560398774460321,
-0.410120565436966));
#45271=CARTESIAN_POINT('Ctrl Pts',(-0.0624083797045926,0.0740365627828155,
-0.411967643999934));
#45272=CARTESIAN_POINT('Ctrl Pts',(-0.0380284501393496,0.0945873804368201,
-0.414076864338557));
#45273=CARTESIAN_POINT('Ctrl Pts',(-0.00250218861058814,0.10191503623145,
-0.416186084677181));
#45274=CARTESIAN_POINT('Ctrl Pts',(0.0280196718242732,0.0926882758330654,
-0.418295305015805));
#45275=CARTESIAN_POINT('Ctrl Pts',(0.058541532259135,0.0834615154346805,
-0.420404525354429));
#45276=CARTESIAN_POINT('Ctrl Pts',(0.0840589916000967,0.0576803388432805,
-0.422513745693054));
#45277=CARTESIAN_POINT('Ctrl Pts',(0.0929714575983574,0.0270652278409629,
-0.424622966031678));
#45278=CARTESIAN_POINT('Ctrl Pts',(0.101883923596618,-0.00354988316135429,
-0.426732186370302));
#45279=CARTESIAN_POINT('Ctrl Pts',(0.0941913962521782,-0.038998928574589,
-0.428841406708925));
#45280=CARTESIAN_POINT('Ctrl Pts',(0.0733910055846535,-0.0631662788623783,
-0.430950627047549));
#45281=CARTESIAN_POINT('Ctrl Pts',(0.0525906149171285,-0.087333629150168,
-0.433059847386173));
#45282=CARTESIAN_POINT('Ctrl Pts',(0.0186823609265183,-0.100219284312512,
-0.435169067724798));
#45283=CARTESIAN_POINT('Ctrl Pts',(-0.0129185920811288,-0.0959652461294597,
-0.437278288063422));
#45284=CARTESIAN_POINT('Ctrl Pts',(-0.0445195450887755,-0.0917112079464077,
-0.439387508402046));
#45285=CARTESIAN_POINT('Ctrl Pts',(-0.0738131971134591,-0.0703174764179602,
-0.441496728740669));
#45286=CARTESIAN_POINT('Ctrl Pts',(-0.0874822461434114,-0.041509939722312,
-0.443605949079293));
#45287=CARTESIAN_POINT('Ctrl Pts',(-0.0935750180900934,-0.0286694157730852,
-0.444546102156539));
#45288=CARTESIAN_POINT('Ctrl Pts',(-0.0965635004074205,-0.0143559200944416,
-0.445486255233785));
#45289=CARTESIAN_POINT('Ctrl Pts',(-0.096526423484871,-2.77199618692811E-5,
-0.446426408311032));
#45290=CARTESIAN_POINT('Ctrl Pts',(-0.0965281097149038,-3.05597964714245E-5,
-0.452223591688967));
#45291=CARTESIAN_POINT('Ctrl Pts',(-0.0965684947496539,-0.0141719696508128,
-0.451295654374683));
#45292=CARTESIAN_POINT('Ctrl Pts',(-0.0936602978316979,-0.028297569349907,
-0.4503677170604));
#45293=CARTESIAN_POINT('Ctrl Pts',(-0.0877197475004104,-0.0410056587084708,
-0.449439779746116));
#45294=CARTESIAN_POINT('Ctrl Pts',(-0.0742167560930221,-0.0698914036047387,
-0.447330559407492));
#45295=CARTESIAN_POINT('Ctrl Pts',(-0.0450467432051246,-0.0914534095013585,
-0.445221339068867));
#45296=CARTESIAN_POINT('Ctrl Pts',(-0.0134708027757043,-0.0958892883497912,
-0.443112118730243));
#45297=CARTESIAN_POINT('Ctrl Pts',(0.0181051376537155,-0.100325167198224,
-0.441002898391619));
#45298=CARTESIAN_POINT('Ctrl Pts',(0.0520870056246581,-0.0876349189984701,
-0.438893678052996));
#45299=CARTESIAN_POINT('Ctrl Pts',(0.0730261708908248,-0.0635877072449965,
-0.436784457714372));
#45300=CARTESIAN_POINT('Ctrl Pts',(0.0939653361569919,-0.0395404954915226,
-0.434675237375748));
#45301=CARTESIAN_POINT('Ctrl Pts',(0.101861798718383,-0.00413632018432857,
-0.432566017037124));
#45302=CARTESIAN_POINT('Ctrl Pts',(0.0931257167667431,0.0265295877150718,
-0.4304567966985));
#45303=CARTESIAN_POINT('Ctrl Pts',(0.0843896348151035,0.0571954956144718,
-0.428347576359876));
#45304=CARTESIAN_POINT('Ctrl Pts',(0.0590210083504338,0.0831231361060782,
-0.426238356021252));
#45305=CARTESIAN_POINT('Ctrl Pts',(0.0285527681240471,0.092525442879814,
-0.424129135682628));
#45306=CARTESIAN_POINT('Ctrl Pts',(-0.00191547210233993,0.10192774965355,
-0.422019915344004));
#45307=CARTESIAN_POINT('Ctrl Pts',(-0.0374833260904441,0.0948047227094148,
-0.41991069500538));
#45308=CARTESIAN_POINT('Ctrl Pts',(-0.0619811522718143,0.0743945892569446,
-0.417801474666756));
#45309=CARTESIAN_POINT('Ctrl Pts',(-0.0835761788238258,0.0564028960114691,
-0.415942180340826));
#45310=CARTESIAN_POINT('Ctrl Pts',(-0.0965691724858363,0.0280863752955406,
-0.414082886014897));
#45311=CARTESIAN_POINT('Ctrl Pts',(-0.0967786908216685,-6.15870636970637E-5,
-0.412223591688967));
#45312=CARTESIAN_POINT('Origin',(0.,0.,-0.493));
#45313=CARTESIAN_POINT('',(-0.0967091013458909,8.3442749783804E-5,-0.366426408311032));
#45314=CARTESIAN_POINT('',(-0.096703565001884,8.42524377135991E-5,-0.372223591688967));
#45315=CARTESIAN_POINT('',(-0.096675,-1.1839272930757E-17,-0.493));
#45316=CARTESIAN_POINT('Ctrl Pts',(-0.0967091013458909,8.3442749783804E-5,
-0.366426408311032));
#45317=CARTESIAN_POINT('Ctrl Pts',(-0.0967663269514072,0.0063910955402476,
-0.366842277836965));
#45318=CARTESIAN_POINT('Ctrl Pts',(-0.0962015802620651,0.0126885502496758,
-0.367258147362897));
#45319=CARTESIAN_POINT('Ctrl Pts',(-0.0949773870582177,0.0188550903906585,
-0.36767401688883));
#45320=CARTESIAN_POINT('Ctrl Pts',(-0.0887684848835039,0.0501307455498909,
-0.369783237227454));
#45321=CARTESIAN_POINT('Ctrl Pts',(-0.0655963240856761,0.0780388225458823,
-0.371892457566078));
#45322=CARTESIAN_POINT('Ctrl Pts',(-0.0359952915465715,0.0898919210637069,
-0.374001677904702));
#45323=CARTESIAN_POINT('Ctrl Pts',(-0.00639425900746725,0.101745019581531,
-0.376110898243326));
#45324=CARTESIAN_POINT('Ctrl Pts',(0.0296356452729136,0.0975431396211891,
-0.37822011858195));
#45325=CARTESIAN_POINT('Ctrl Pts',(0.0557147252309796,0.0791965143076565,
-0.380329338920574));
#45326=CARTESIAN_POINT('Ctrl Pts',(0.081793805189046,0.0608498889941236,
-0.382438559259198));
#45327=CARTESIAN_POINT('Ctrl Pts',(0.0979220608247974,0.0283585183273998,
-0.384547779597822));
#45328=CARTESIAN_POINT('Ctrl Pts',(0.0967673626023422,-0.00350656827015149,
-0.386656999936446));
#45329=CARTESIAN_POINT('Ctrl Pts',(0.095612664379887,-0.0353716548677019,
-0.38876622027507));
#45330=CARTESIAN_POINT('Ctrl Pts',(0.0771750122992263,-0.0666104573960799,
-0.390875440613694));
#45331=CARTESIAN_POINT('Ctrl Pts',(0.0498364196695632,-0.0830213813458049,
-0.392984660952318));
#45332=CARTESIAN_POINT('Ctrl Pts',(0.0224978270398989,-0.0994323052955306,
-0.395093881290942));
#45333=CARTESIAN_POINT('Ctrl Pts',(-0.0137417061387687,-0.101015350666602,
-0.397203101629565));
#45334=CARTESIAN_POINT('Ctrl Pts',(-0.0424071835874108,-0.0870508429955163,
-0.399312321968189));
#45335=CARTESIAN_POINT('Ctrl Pts',(-0.071072661036052,-0.0730863353244312,
-0.401421542306813));
#45336=CARTESIAN_POINT('Ctrl Pts',(-0.0921640827546683,-0.0435742746111902,
-0.403530762645437));
#45337=CARTESIAN_POINT('Ctrl Pts',(-0.0960929948131144,-0.01193125449788,
-0.405639982984062));
#45338=CARTESIAN_POINT('Ctrl Pts',(-0.0965812946671128,-0.00799854186101098,
-0.405902124759718));
#45339=CARTESIAN_POINT('Ctrl Pts',(-0.0968044947410041,-0.00403291347466469,
-0.406164266535375));
#45340=CARTESIAN_POINT('Ctrl Pts',(-0.0967741445435993,-6.3845289803563E-5,
-0.406426408311032));
#45341=CARTESIAN_POINT('Ctrl Pts',(-0.0967786908216685,-6.15870636970637E-5,
-0.412223591688967));
#45342=CARTESIAN_POINT('Ctrl Pts',(-0.0968068542391171,-0.0038452311591,
-0.411973665676273));
#45343=CARTESIAN_POINT('Ctrl Pts',(-0.0966040370216943,-0.00762582962604524,
-0.411723739663579));
#45344=CARTESIAN_POINT('Ctrl Pts',(-0.0961600833242075,-0.0113778962349287,
-0.411473813650884));
#45345=CARTESIAN_POINT('Ctrl Pts',(-0.0924133898205945,-0.043043008313528,
-0.40936459331226));
#45346=CARTESIAN_POINT('Ctrl Pts',(-0.071492204438732,-0.0726759925099216,
-0.407255372973636));
#45347=CARTESIAN_POINT('Ctrl Pts',(-0.0429075893001909,-0.0868052816831873,
-0.405146152635012));
#45348=CARTESIAN_POINT('Ctrl Pts',(-0.0143229741616502,-0.100934570856453,
-0.403036932296388));
#45349=CARTESIAN_POINT('Ctrl Pts',(0.02192507073357,-0.0995601650065905,
-0.400927711957764));
#45350=CARTESIAN_POINT('Ctrl Pts',(0.0493576795616014,-0.0833068881662591,
-0.39881849161914));
#45351=CARTESIAN_POINT('Ctrl Pts',(0.0767902883896333,-0.0670536113259275,
-0.396709271280516));
#45352=CARTESIAN_POINT('Ctrl Pts',(0.0954074611504771,-0.035921463495128,
-0.394600050941892));
#45353=CARTESIAN_POINT('Ctrl Pts',(0.0967455719345851,-0.00406355247306422,
-0.392490830603268));
#45354=CARTESIAN_POINT('Ctrl Pts',(0.0980836827186931,0.0277943585489991,
-0.390381610264644));
#45355=CARTESIAN_POINT('Ctrl Pts',(0.0821427315260642,0.0603780327623262,
-0.38827238992602));
#45356=CARTESIAN_POINT('Ctrl Pts',(0.0561696966852534,0.0788744782672949,
-0.386163169587396));
#45357=CARTESIAN_POINT('Ctrl Pts',(0.0301966618444426,0.0973709237722636,
-0.384053949248772));
#45358=CARTESIAN_POINT('Ctrl Pts',(-0.00580845664455006,0.101780140568875,
-0.381944728910148));
#45359=CARTESIAN_POINT('Ctrl Pts',(-0.0354772306839452,0.0900976373200178,
-0.379835508571524));
#45360=CARTESIAN_POINT('Ctrl Pts',(-0.0651460047233408,0.0784151340711604,
-0.3777262882329));
#45361=CARTESIAN_POINT('Ctrl Pts',(-0.0884784343131384,0.050640910776834,
-0.375617067894276));
#45362=CARTESIAN_POINT('Ctrl Pts',(-0.0948672721475454,0.01940151599579,
-0.373507847555652));
#45363=CARTESIAN_POINT('Ctrl Pts',(-0.0961639444012508,0.0130611991048246,
-0.373079762266757));
#45364=CARTESIAN_POINT('Ctrl Pts',(-0.0967626700723313,0.00657814361201625,
-0.372651676977862));
#45365=CARTESIAN_POINT('Ctrl Pts',(-0.096703565001884,8.42524377135991E-5,
-0.372223591688967));
#45366=CARTESIAN_POINT('Origin',(0.,0.,-0.493));
#45367=CARTESIAN_POINT('',(-0.0965197516312923,-9.65577020483471E-6,-0.326426408311032));
#45368=CARTESIAN_POINT('',(-0.0965203932006718,-1.26410680933947E-5,-0.332223591688967));
#45369=CARTESIAN_POINT('',(-0.096675,-1.1839272930757E-17,-0.493));
#45370=CARTESIAN_POINT('Ctrl Pts',(-0.0965197516312923,-9.65577020483471E-6,
-0.326426408311032));
#45371=CARTESIAN_POINT('Ctrl Pts',(-0.0965047840234489,0.0166642787646163,
-0.327520289138554));
#45372=CARTESIAN_POINT('Ctrl Pts',(-0.0924001255268703,0.0333451168327119,
-0.328614169966076));
#45373=CARTESIAN_POINT('Ctrl Pts',(-0.0842483426464452,0.0477329576642131,
-0.329708050793598));
#45374=CARTESIAN_POINT('Ctrl Pts',(-0.0685300799117474,0.0754755835034765,
-0.331817271132222));
#45375=CARTESIAN_POINT('Ctrl Pts',(-0.0377647994695152,0.0946929536920675,
-0.333926491470846));
#45376=CARTESIAN_POINT('Ctrl Pts',(-0.00593882609689562,0.0966485842143444,
-0.33603571180947));
#45377=CARTESIAN_POINT('Ctrl Pts',(0.0258871472757249,0.0986042147366213,
-0.338144932148094));
#45378=CARTESIAN_POINT('Ctrl Pts',(0.0587738135787319,0.083298105592584,
-0.340254152486718));
#45379=CARTESIAN_POINT('Ctrl Pts',(0.0777704364905394,0.0576886270777644,
-0.342363372825342));
#45380=CARTESIAN_POINT('Ctrl Pts',(0.0967670594023461,0.0320791485629459,
-0.344472593163966));
#45381=CARTESIAN_POINT('Ctrl Pts',(0.101873638922953,-0.00383369932265502,
-0.34658181350259));
#45382=CARTESIAN_POINT('Ctrl Pts',(0.0907686529128285,-0.0337234359820715,
-0.348691033841214));
#45383=CARTESIAN_POINT('Ctrl Pts',(0.0796636669027034,-0.0636131726414893,
-0.350800254179838));
#45384=CARTESIAN_POINT('Ctrl Pts',(0.0523471153618471,-0.0874797980747228,
-0.352909474518462));
#45385=CARTESIAN_POINT('Ctrl Pts',(0.0212374828985647,-0.0944732121089336,
-0.355018694857086));
#45386=CARTESIAN_POINT('Ctrl Pts',(-0.00987214956471671,-0.101466626143144,
-0.35712791519571));
#45387=CARTESIAN_POINT('Ctrl Pts',(-0.0447748629504247,-0.0915868287783316,
-0.359237135534334));
#45388=CARTESIAN_POINT('Ctrl Pts',(-0.067603397867478,-0.069325313434689,
-0.361346355872958));
#45389=CARTESIAN_POINT('Ctrl Pts',(-0.0859308895223161,-0.0514530435686153,
-0.363039706685649));
#45390=CARTESIAN_POINT('Ctrl Pts',(-0.0964760882983722,-0.0256002592597677,
-0.364733057498341));
#45391=CARTESIAN_POINT('Ctrl Pts',(-0.0967091013458909,8.3442749783804E-5,
-0.366426408311032));
#45392=CARTESIAN_POINT('Ctrl Pts',(-0.096703565001884,8.42524377135991E-5,
-0.372223591688967));
#45393=CARTESIAN_POINT('Ctrl Pts',(-0.0964714532986248,-0.0254179274910308,
-0.370542456639238));
#45394=CARTESIAN_POINT('Ctrl Pts',(-0.0860941848055461,-0.0510872168002652,
-0.368861321589509));
#45395=CARTESIAN_POINT('Ctrl Pts',(-0.0680013484513945,-0.0689350038546699,
-0.36718018653978));
#45396=CARTESIAN_POINT('Ctrl Pts',(-0.0453013408418207,-0.0913275626563238,
-0.365070966201156));
#45397=CARTESIAN_POINT('Ctrl Pts',(-0.0104560795436565,-0.101408113991871,
-0.362961745862532));
#45398=CARTESIAN_POINT('Ctrl Pts',(0.0206932945708154,-0.0945938988912964,
-0.360852525523908));
#45399=CARTESIAN_POINT('Ctrl Pts',(0.0518426686852874,-0.0877796837907218,
-0.358743305185284));
#45400=CARTESIAN_POINT('Ctrl Pts',(0.0792961556160677,-0.0640707022540251,
-0.35663408484666));
#45401=CARTESIAN_POINT('Ctrl Pts',(0.090573018020292,-0.0342453873440962,
-0.354524864508036));
#45402=CARTESIAN_POINT('Ctrl Pts',(0.101849880424517,-0.00442007243416647,
-0.352415644169412));
#45403=CARTESIAN_POINT('Ctrl Pts',(0.096950118302185,0.0315215758489951,
-0.350306423830788));
#45404=CARTESIAN_POINT('Ctrl Pts',(0.0781012317244362,0.0572399838467591,
-0.348197203492164));
#45405=CARTESIAN_POINT('Ctrl Pts',(0.059252345146688,0.0829583918445225,
-0.34608798315354));
#45406=CARTESIAN_POINT('Ctrl Pts',(0.026454334113523,0.098453559556888,
-0.343978762814916));
#45407=CARTESIAN_POINT('Ctrl Pts',(-0.00538236897332435,0.0966811680312477,
-0.341869542476292));
#45408=CARTESIAN_POINT('Ctrl Pts',(-0.0372190720601721,0.0949087765056073,
-0.339760322137668));
#45409=CARTESIAN_POINT('Ctrl Pts',(-0.0680944672007028,0.0758688257419608,
-0.337651101799044));
#45410=CARTESIAN_POINT('Ctrl Pts',(-0.083972169942999,0.0482171424154877,
-0.33554188146042));
#45411=CARTESIAN_POINT('Ctrl Pts',(-0.0922985986931762,0.0337163185383023,
-0.334435784869936));
#45412=CARTESIAN_POINT('Ctrl Pts',(-0.0965005716954632,0.0168472163336972,
-0.333329688279452));
#45413=CARTESIAN_POINT('Ctrl Pts',(-0.0965203932006718,-1.26410680933947E-5,
-0.332223591688967));
#45414=CARTESIAN_POINT('Origin',(0.,0.,-0.493));
#45415=CARTESIAN_POINT('',(-0.0967437690459326,-7.5552805846299E-5,-0.286426408311032));
#45416=CARTESIAN_POINT('',(-0.0967489390155672,-7.39178419271937E-5,-0.292223591688967));
#45417=CARTESIAN_POINT('',(-0.096675,-1.1839272930757E-17,-0.493));
#45418=CARTESIAN_POINT('Ctrl Pts',(-0.0967437690459326,-7.5552805846299E-5,
-0.286426408311032));
#45419=CARTESIAN_POINT('Ctrl Pts',(-0.0965129181057634,0.0267745038977835,
-0.288198300440143));
#45420=CARTESIAN_POINT('Ctrl Pts',(-0.0848482692534772,0.05380059796138,
-0.289970192569255));
#45421=CARTESIAN_POINT('Ctrl Pts',(-0.0649918357452926,0.0717793826422552,
-0.291742084698366));
#45422=CARTESIAN_POINT('Ctrl Pts',(-0.0413551861322041,0.0931809215337106,
-0.29385130503699));
#45423=CARTESIAN_POINT('Ctrl Pts',(-0.00611079122009462,0.101762438004232,
-0.295960525375614));
#45424=CARTESIAN_POINT('Ctrl Pts',(0.024718756421455,0.0936226552017361,
-0.298069745714238));
#45425=CARTESIAN_POINT('Ctrl Pts',(0.0555483040630038,0.0854828723992403,
-0.300178966052862));
#45426=CARTESIAN_POINT('Ctrl Pts',(0.0819630044339925,0.0606217903237279,
-0.302288186391486));
#45427=CARTESIAN_POINT('Ctrl Pts',(0.0919543670227436,0.0303416029815987,
-0.30439740673011));
#45428=CARTESIAN_POINT('Ctrl Pts',(0.101945729611495,6.14156394686538E-5,
-0.306506627068734));
#45429=CARTESIAN_POINT('Ctrl Pts',(0.0955137544180066,-0.0356378769692795,
-0.308615847407358));
#45430=CARTESIAN_POINT('Ctrl Pts',(0.0755825069057357,-0.0605268794494711,
-0.310725067745982));
#45431=CARTESIAN_POINT('Ctrl Pts',(0.055651259393465,-0.0854158819296624,
-0.312834288084606));
#45432=CARTESIAN_POINT('Ctrl Pts',(0.0222207395624123,-0.0994945942812985,
-0.31494350842323));
#45433=CARTESIAN_POINT('Ctrl Pts',(-0.00951107288091885,-0.0963626378774484,
-0.317052728761854));
#45434=CARTESIAN_POINT('Ctrl Pts',(-0.0412428853242505,-0.0932306814735982,
-0.319161949100478));
#45435=CARTESIAN_POINT('Ctrl Pts',(-0.0712759903798599,-0.0728880563142611,
-0.321271169439102));
#45436=CARTESIAN_POINT('Ctrl Pts',(-0.0859569203940831,-0.0445828029896242,
-0.323380389777726));
#45437=CARTESIAN_POINT('Ctrl Pts',(-0.093024047535901,-0.0309571795561787,
-0.324395729288828));
#45438=CARTESIAN_POINT('Ctrl Pts',(-0.0965336445556838,-0.0154863915468829,
-0.32541106879993));
#45439=CARTESIAN_POINT('Ctrl Pts',(-0.0965197516312923,-9.65577020483471E-6,
-0.326426408311032));
#45440=CARTESIAN_POINT('Ctrl Pts',(-0.0965203932006718,-1.26410680933947E-5,
-0.332223591688967));
#45441=CARTESIAN_POINT('Ctrl Pts',(-0.0965383694088707,-0.0153029181519232,
-0.331220467940828));
#45442=CARTESIAN_POINT('Ctrl Pts',(-0.0931166288935622,-0.0305855916128645,
-0.330217344192688));
#45443=CARTESIAN_POINT('Ctrl Pts',(-0.0862121360220177,-0.0440872515606547,
-0.329214220444548));
#45444=CARTESIAN_POINT('Ctrl Pts',(-0.0716943890146783,-0.072476546321024,
-0.327105000105924));
#45445=CARTESIAN_POINT('Ctrl Pts',(-0.0417788846559379,-0.0929917199524636,
-0.3249957797673));
#45446=CARTESIAN_POINT('Ctrl Pts',(-0.0100656276855269,-0.0963062889272953,
-0.322886559428676));
#45447=CARTESIAN_POINT('Ctrl Pts',(0.0216476292848846,-0.0996208579021272,
-0.320777339090052));
#45448=CARTESIAN_POINT('Ctrl Pts',(0.0551586388669668,-0.0857348222203507,
-0.318668118751428));
#45449=CARTESIAN_POINT('Ctrl Pts',(0.0752328295928874,-0.0609609670124983,
-0.316558898412804));
#45450=CARTESIAN_POINT('Ctrl Pts',(0.0953070203188076,-0.0361871118046462,
-0.31444967807418));
#45451=CARTESIAN_POINT('Ctrl Pts',(0.101944392188567,-0.000525437070718525,
-0.312340457735557));
#45452=CARTESIAN_POINT('Ctrl Pts',(0.0921275035503174,0.02981176340369,
-0.310231237396933));
#45453=CARTESIAN_POINT('Ctrl Pts',(0.0823106149120679,0.0601489638780991,
-0.308122017058309));
#45454=CARTESIAN_POINT('Ctrl Pts',(0.0560394657658096,0.0851616900929888,
-0.306012796719685));
#45455=CARTESIAN_POINT('Ctrl Pts',(0.0252572862380605,0.0934788085051367,
-0.30390357638106));
#45456=CARTESIAN_POINT('Ctrl Pts',(-0.00552489328968782,0.101795926917284,
-0.301794356042436));
#45457=CARTESIAN_POINT('Ctrl Pts',(-0.0408181031989268,0.0934174375266914,
-0.299685135703812));
#45458=CARTESIAN_POINT('Ctrl Pts',(-0.0645775589428199,0.0721523182485355,
-0.297575915365188));
#45459=CARTESIAN_POINT('Ctrl Pts',(-0.0846747634538068,0.0541649764638451,
-0.295791807473115));
#45460=CARTESIAN_POINT('Ctrl Pts',(-0.0965197817739755,0.0269574911179326,
-0.294007699581041));
#45461=CARTESIAN_POINT('Ctrl Pts',(-0.0967489390155672,-7.39178419271937E-5,
-0.292223591688967));
#45462=CARTESIAN_POINT('Origin',(0.,0.,-0.493));
#45463=CARTESIAN_POINT('',(-0.0967423356012983,7.59830402560519E-5,-0.246426408311031));
#45464=CARTESIAN_POINT('',(-0.0967370704137262,7.74805285259637E-5,-0.252223591688967));
#45465=CARTESIAN_POINT('',(-0.096675,-1.1839272930757E-17,-0.493));
#45466=CARTESIAN_POINT('Ctrl Pts',(-0.0967423356012983,7.59830402560519E-5,
-0.246426408311031));
#45467=CARTESIAN_POINT('Ctrl Pts',(-0.0967868821729931,0.00523866323318436,
-0.246767091403108));
#45468=CARTESIAN_POINT('Ctrl Pts',(-0.096408980193914,0.0103948133764852,
-0.247107774495185));
#45469=CARTESIAN_POINT('Ctrl Pts',(-0.0955856895060027,0.0154788387067367,
-0.247448457587262));
#45470=CARTESIAN_POINT('Ctrl Pts',(-0.0904885728485377,0.046954805310395,
-0.249557677925886));
#45471=CARTESIAN_POINT('Ctrl Pts',(-0.0683195528466901,0.0756662028697691,
-0.251666898264511));
#45472=CARTESIAN_POINT('Ctrl Pts',(-0.0391569746115824,0.0885604303586767,
-0.253776118603135));
#45473=CARTESIAN_POINT('Ctrl Pts',(-0.00999439637647477,0.101454657847584,
-0.255885338941759));
#45474=CARTESIAN_POINT('Ctrl Pts',(0.0261617400918925,0.0985317152660251,
-0.257994559280382));
#45475=CARTESIAN_POINT('Ctrl Pts',(0.0528743518199786,0.0811204130022984,
-0.260103779619006));
#45476=CARTESIAN_POINT('Ctrl Pts',(0.0795869635480646,0.0637091107385717,
-0.26221299995763));
#45477=CARTESIAN_POINT('Ctrl Pts',(0.0968560505358691,0.0318094487926776,
-0.264322220296255));
#45478=CARTESIAN_POINT('Ctrl Pts',(0.0968308454331686,-7.65424347751696E-5,
-0.266431440634879));
#45479=CARTESIAN_POINT('Ctrl Pts',(0.0968056403304681,-0.031962533662227,
-0.268540660973503));
#45480=CARTESIAN_POINT('Ctrl Pts',(0.0794861431372628,-0.0638348541712385,
-0.270649881312126));
#45481=CARTESIAN_POINT('Ctrl Pts',(0.0527460383849185,-0.0812039033590322,
-0.27275910165075));
#45482=CARTESIAN_POINT('Ctrl Pts',(0.0260059336325734,-0.0985729525468265,
-0.274868321989374));
#45483=CARTESIAN_POINT('Ctrl Pts',(-0.0101547786789113,-0.101438730413403,
-0.276977542327999));
#45484=CARTESIAN_POINT('Ctrl Pts',(-0.0392969353340071,-0.0884984144456908,
-0.279086762666623));
#45485=CARTESIAN_POINT('Ctrl Pts',(-0.0684390919891021,-0.0755580984779786,
-0.281195983005247));
#45486=CARTESIAN_POINT('Ctrl Pts',(-0.0905626929878082,-0.0468116886759782,
-0.28330520334387));
#45487=CARTESIAN_POINT('Ctrl Pts',(-0.0956100413301282,-0.015327703118784,
-0.285414423682494));
#45488=CARTESIAN_POINT('Ctrl Pts',(-0.0964172651881209,-0.0102924603412303,
-0.285751751892007));
#45489=CARTESIAN_POINT('Ctrl Pts',(-0.0967877178467835,-0.00518719668322276,
-0.286089080101519));
#45490=CARTESIAN_POINT('Ctrl Pts',(-0.0967437690459326,-7.5552805846299E-5,
-0.286426408311032));
#45491=CARTESIAN_POINT('Ctrl Pts',(-0.0967489390155672,-7.39178419271937E-5,
-0.292223591688967));
#45492=CARTESIAN_POINT('Ctrl Pts',(-0.0967906976288156,-0.00499976764040804,
-0.291898479242417));
#45493=CARTESIAN_POINT('Ctrl Pts',(-0.0964467324983444,-0.00991977053332167,
-0.291573366795867));
#45494=CARTESIAN_POINT('Ctrl Pts',(-0.0956966895450183,-0.0147770686462416,
-0.291248254349317));
#45495=CARTESIAN_POINT('Ctrl Pts',(-0.0908306628247752,-0.0462895870971385,
-0.289139034010693));
#45496=CARTESIAN_POINT('Ctrl Pts',(-0.0688729078057432,-0.0751628748332125,
-0.287029813672068));
#45497=CARTESIAN_POINT('Ctrl Pts',(-0.0398057255967931,-0.0882707333002516,
-0.284920593333444));
#45498=CARTESIAN_POINT('Ctrl Pts',(-0.0107385433878433,-0.101378591767291,
-0.28281137299482));
#45499=CARTESIAN_POINT('Ctrl Pts',(0.0254380660110247,-0.0987210209652953,
-0.280702152656197));
#45500=CARTESIAN_POINT('Ctrl Pts',(0.0522777123470515,-0.0815061895772969,
-0.278592932317573));
#45501=CARTESIAN_POINT('Ctrl Pts',(0.0791173586830794,-0.0642913581892978,
-0.276483711978949));
#45502=CARTESIAN_POINT('Ctrl Pts',(0.0966200419562655,-0.0325192662152939,
-0.274374491640325));
#45503=CARTESIAN_POINT('Ctrl Pts',(0.0968287986931256,-0.000633948970751547,
-0.272265271301701));
#45504=CARTESIAN_POINT('Ctrl Pts',(0.0970375554299856,0.0312513682737899,
-0.270156050963076));
#45505=CARTESIAN_POINT('Ctrl Pts',(0.0799523856305208,0.0632499107888704,
-0.268046830624453));
#45506=CARTESIAN_POINT('Ctrl Pts',(0.0533404453307932,0.0808146956905983,
-0.265937610285829));
#45507=CARTESIAN_POINT('Ctrl Pts',(0.0267285050310652,0.0983794805923265,
-0.263828389947205));
#45508=CARTESIAN_POINT('Ctrl Pts',(-0.00941020576892441,0.101510507880702,
-0.261719169608581));
#45509=CARTESIAN_POINT('Ctrl Pts',(-0.0386465260470608,0.0887843689629269,
-0.259609949269957));
#45510=CARTESIAN_POINT('Ctrl Pts',(-0.0678828463251972,0.076058230045152,
-0.257500728931333));
#45511=CARTESIAN_POINT('Ctrl Pts',(-0.0902167760814793,0.0474749249212259,
-0.255391508592709));
#45512=CARTESIAN_POINT('Ctrl Pts',(-0.0954949999346953,0.016028822012986,
-0.253282288254085));
#45513=CARTESIAN_POINT('Ctrl Pts',(-0.0963781125807907,0.0107674970065134,
-0.252929389399046));
#45514=CARTESIAN_POINT('Ctrl Pts',(-0.0967837769872234,0.00542603238163979,
-0.252576490544006));
#45515=CARTESIAN_POINT('Ctrl Pts',(-0.0967370704137262,7.74805285259636E-5,
-0.252223591688967));
#45516=CARTESIAN_POINT('Origin',(0.,0.,-0.493));
#45517=CARTESIAN_POINT('',(-0.096519605166994,8.83378289982806E-6,-0.206426408311032));
#45518=CARTESIAN_POINT('',(-0.0965191803594238,5.8347464585056E-6,-0.212223591688967));
#45519=CARTESIAN_POINT('',(-0.096675,-1.1839272930757E-17,-0.493));
#45520=CARTESIAN_POINT('Ctrl Pts',(-0.096519605166994,8.83378289982806E-6,
-0.206426408311032));
#45521=CARTESIAN_POINT('Ctrl Pts',(-0.0965323562986513,0.0155367666085817,
-0.207445102704698));
#45522=CARTESIAN_POINT('Ctrl Pts',(-0.0929984118487813,0.0310592225023218,
-0.208463797098364));
#45523=CARTESIAN_POINT('Ctrl Pts',(-0.085886329768773,0.0447186409110356,
-0.209482491492031));
#45524=CARTESIAN_POINT('Ctrl Pts',(-0.0711606688969908,0.0730006490388526,
-0.211591711830655));
#45525=CARTESIAN_POINT('Ctrl Pts',(-0.0410954406900119,0.0932957679232711,
-0.213700932169279));
#45526=CARTESIAN_POINT('Ctrl Pts',(-0.00935871643388856,0.0963775539882049,
-0.215810152507903));
#45527=CARTESIAN_POINT('Ctrl Pts',(0.0223780078222335,0.0994593400531385,
-0.217919372846527));
#45528=CARTESIAN_POINT('Ctrl Pts',(0.0557862281274994,0.0853277932985902,
-0.220028593185151));
#45529=CARTESIAN_POINT('Ctrl Pts',(0.0756781024505724,0.0604073116064739,
-0.222137813523775));
#45530=CARTESIAN_POINT('Ctrl Pts',(0.0955699767736457,0.0354868299143573,
-0.224247033862399));
#45531=CARTESIAN_POINT('Ctrl Pts',(0.101945505114525,-0.000222586715327797,
-0.226356254201023));
#45532=CARTESIAN_POINT('Ctrl Pts',(0.0919062835345921,-0.0304869403665019,
-0.228465474539647));
#45533=CARTESIAN_POINT('Ctrl Pts',(0.081867061954659,-0.0607512940176778,
-0.230574694878271));
#45534=CARTESIAN_POINT('Ctrl Pts',(0.0554130904539123,-0.0855705846903427,
-0.232683915216895));
#45535=CARTESIAN_POINT('Ctrl Pts',(0.0245707127464045,-0.0936616173316404,
-0.234793135555519));
#45536=CARTESIAN_POINT('Ctrl Pts',(-0.00627166496110106,-0.101752649972938,
-0.236902355894143));
#45537=CARTESIAN_POINT('Ctrl Pts',(-0.0415024488753662,-0.0931154245828709,
-0.239011576232767));
#45538=CARTESIAN_POINT('Ctrl Pts',(-0.065105234175958,-0.0716765440638671,
-0.241120796571391));
#45539=CARTESIAN_POINT('Ctrl Pts',(-0.084895677195098,-0.0537004900557472,
-0.242889333817938));
#45540=CARTESIAN_POINT('Ctrl Pts',(-0.0965110876377789,-0.0267242674727368,
-0.244657871064485));
#45541=CARTESIAN_POINT('Ctrl Pts',(-0.0967423356012983,7.59830402560519E-5,
-0.246426408311031));
#45542=CARTESIAN_POINT('Ctrl Pts',(-0.0967370704137262,7.74805285259636E-5,
-0.252223591688967));
#45543=CARTESIAN_POINT('Ctrl Pts',(-0.0965046192247059,-0.0265414115181691,
-0.250467270205382));
#45544=CARTESIAN_POINT('Ctrl Pts',(-0.08506741559802,-0.0533358467394369,
-0.248710948721798));
#45545=CARTESIAN_POINT('Ctrl Pts',(-0.065516761081115,-0.0713005761904585,
-0.246954627238213));
#45546=CARTESIAN_POINT('Ctrl Pts',(-0.0420377804241679,-0.0928749707931102,
-0.244845406899589));
#45547=CARTESIAN_POINT('Ctrl Pts',(-0.00685730116012349,-0.101714859305859,
-0.242736186560965));
#45548=CARTESIAN_POINT('Ctrl Pts',(0.0240311410848332,-0.0938015053493915,
-0.240626966222341));
#45549=CARTESIAN_POINT('Ctrl Pts',(0.0549195833297894,-0.0858881513929241,
-0.238517745883717));
#45550=CARTESIAN_POINT('Ctrl Pts',(0.0815159885556585,-0.0612215549672399,
-0.236408525545093));
#45551=CARTESIAN_POINT('Ctrl Pts',(0.0917292606941796,-0.0310154941948588,
-0.234299305206469));
#45552=CARTESIAN_POINT('Ctrl Pts',(0.101942532832701,-0.000809433422477208,
-0.232190084867845));
#45553=CARTESIAN_POINT('Ctrl Pts',(0.0957726718838747,0.0349360916966021,
-0.230080864529221));
#45554=CARTESIAN_POINT('Ctrl Pts',(0.0760245825266243,0.0599706678243891,
-0.227971644190597));
#45555=CARTESIAN_POINT('Ctrl Pts',(0.0562764931693742,0.0850052439521758,
-0.225862423851973));
#45556=CARTESIAN_POINT('Ctrl Pts',(0.0229501754037008,0.0993288710886704,
-0.223753203513349));
#45557=CARTESIAN_POINT('Ctrl Pts',(-0.00880376277346886,0.0964298289362705,
-0.221643983174725));
#45558=CARTESIAN_POINT('Ctrl Pts',(-0.0405577009506385,0.0935307867838707,
-0.219534762836101));
#45559=CARTESIAN_POINT('Ctrl Pts',(-0.0707392595393038,0.0734090753425766,
-0.217425542497477));
#45560=CARTESIAN_POINT('Ctrl Pts',(-0.0856274818429496,0.0452123047509388,
-0.215316322158853));
#45561=CARTESIAN_POINT('Ctrl Pts',(-0.0929043031905888,0.0314307492373925,
-0.214285412002224));
#45562=CARTESIAN_POINT('Ctrl Pts',(-0.0965277014070608,0.0157201438856951,
-0.213254501845596));
#45563=CARTESIAN_POINT('Ctrl Pts',(-0.0965191803594238,5.8347464585056E-6,
-0.212223591688967));
#45564=CARTESIAN_POINT('Origin',(0.,0.,-0.493));
#45565=CARTESIAN_POINT('',(-0.0967106172141971,-8.32004823464877E-5,-0.166426408311032));
#45566=CARTESIAN_POINT('',(-0.0967161166967018,-8.22460629427947E-5,-0.172223591688967));
#45567=CARTESIAN_POINT('',(-0.096675,-1.1839272930757E-17,-0.493));
#45568=CARTESIAN_POINT('Ctrl Pts',(-0.0967106172141971,-8.32004823464877E-5,
-0.166426408311032));
#45569=CARTESIAN_POINT('Ctrl Pts',(-0.0964774108677986,0.025650346436811,
-0.168123114006287));
#45570=CARTESIAN_POINT('Ctrl Pts',(-0.0858858039544249,0.0515534804917154,
-0.169819819701543));
#45571=CARTESIAN_POINT('Ctrl Pts',(-0.0674937135020625,0.0694321044270534,
-0.171516525396799));
#45572=CARTESIAN_POINT('Ctrl Pts',(-0.0446300127669237,0.0916575011687899,
-0.173625745735423));
#45573=CARTESIAN_POINT('Ctrl Pts',(-0.00971172351316946,0.101482106719653,
-0.175734966074047));
#45574=CARTESIAN_POINT('Ctrl Pts',(0.0213868138345207,0.0944395186348712,
-0.177844186412671));
#45575=CARTESIAN_POINT('Ctrl Pts',(0.0524853511822118,0.0873969305500895,
-0.179953406751295));
#45576=CARTESIAN_POINT('Ctrl Pts',(0.079764136623838,0.0634871488296626,
-0.182062627089919));
#45577=CARTESIAN_POINT('Ctrl Pts',(0.0908218545598657,0.0335798930909097,
-0.184171847428543));
#45578=CARTESIAN_POINT('Ctrl Pts',(0.101879572495893,0.00367263735215799,
-0.186281067767167));
#45579=CARTESIAN_POINT('Ctrl Pts',(0.0967162229263223,-0.0322320924049201,
-0.188390288105791));
#45580=CARTESIAN_POINT('Ctrl Pts',(0.0776791364377021,-0.0578115061952451,
-0.190499508444415));
#45581=CARTESIAN_POINT('Ctrl Pts',(0.0586420499490815,-0.0833909199855704,
-0.192608728783039));
#45582=CARTESIAN_POINT('Ctrl Pts',(0.0257312265414111,-0.0986450178091434,
-0.194717949121663));
#45583=CARTESIAN_POINT('Ctrl Pts',(-0.00609161530366864,-0.0966390744420128,
-0.196827169460287));
#45584=CARTESIAN_POINT('Ctrl Pts',(-0.0379144571487484,-0.0946331310748821,
-0.198936389798911));
#45585=CARTESIAN_POINT('Ctrl Pts',(-0.0686493174312371,-0.0753671465170478,
-0.201045610137535));
#45586=CARTESIAN_POINT('Ctrl Pts',(-0.0843237008041889,-0.0475997055525231,
-0.203154830476159));
#45587=CARTESIAN_POINT('Ctrl Pts',(-0.0924277956805772,-0.0332431614578228,
-0.204245356421116));
#45588=CARTESIAN_POINT('Ctrl Pts',(-0.0965059549103652,-0.0166140255586733,
-0.205335882366074));
#45589=CARTESIAN_POINT('Ctrl Pts',(-0.096519605166994,8.83378289982806E-6,
-0.206426408311032));
#45590=CARTESIAN_POINT('Ctrl Pts',(-0.0965191803594238,5.8347464585056E-6,
-0.212223591688967));
#45591=CARTESIAN_POINT('Ctrl Pts',(-0.0965102675241303,-0.0164309996749581,
-0.211145281506972));
#45592=CARTESIAN_POINT('Ctrl Pts',(-0.0925277746875275,-0.0328718863054202,
-0.210066971324976));
#45593=CARTESIAN_POINT('Ctrl Pts',(-0.0845963103545643,-0.0471135057286142,
-0.208988661142981));
#45594=CARTESIAN_POINT('Ctrl Pts',(-0.0690820305439074,-0.0749707158745457,
-0.206879440804357));
#45595=CARTESIAN_POINT('Ctrl Pts',(-0.0384585849039681,-0.0944133064244279,
-0.204770220465733));
#45596=CARTESIAN_POINT('Ctrl Pts',(-0.00664781813597963,-0.096602405051195,
-0.202661000127109));
#45597=CARTESIAN_POINT('Ctrl Pts',(0.0251629486320089,-0.0987915036779621,
-0.200551779788485));
#45598=CARTESIAN_POINT('Ctrl Pts',(0.0581610365280471,-0.083727110381614,
-0.198442559449861));
#45599=CARTESIAN_POINT('Ctrl Pts',(0.0773450554226922,-0.0582577080680854,
-0.196333339111237));
#45600=CARTESIAN_POINT('Ctrl Pts',(0.096529074317338,-0.0327883057545557,
-0.194224118772613));
#45601=CARTESIAN_POINT('Ctrl Pts',(0.10189902421059,0.00308610557615446,
-0.192114898433989));
#45602=CARTESIAN_POINT('Ctrl Pts',(0.0910136511261294,0.0330565191194918,
-0.190005678095365));
#45603=CARTESIAN_POINT('Ctrl Pts',(0.0801282780416693,0.063026932662828,
-0.187896457756741));
#45604=CARTESIAN_POINT('Ctrl Pts',(0.0529875819794976,0.087093348418791,
-0.185787237418117));
#45605=CARTESIAN_POINT('Ctrl Pts',(0.0219301011972353,0.0943148387535103,
-0.183678017079493));
#45606=CARTESIAN_POINT('Ctrl Pts',(-0.00912737958502692,0.10153632908823,
-0.181568796740869));
#45607=CARTESIAN_POINT('Ctrl Pts',(-0.0441016450873802,0.0919128940017052,
-0.179459576402245));
#45608=CARTESIAN_POINT('Ctrl Pts',(-0.0670929073267039,0.0698194810516787,
-0.177350356063621));
#45609=CARTESIAN_POINT('Ctrl Pts',(-0.08572076742876,0.0519190716993752,
-0.175641434605403));
#45610=CARTESIAN_POINT('Ctrl Pts',(-0.0964824094446633,0.0258327707762626,
-0.173932513147185));
#45611=CARTESIAN_POINT('Ctrl Pts',(-0.0967161166967018,-8.22460629427947E-5,
-0.172223591688967));
#45612=CARTESIAN_POINT('Origin',(0.,0.,-0.493));
#45613=CARTESIAN_POINT('',(-0.0967728733759203,6.44486977623322E-5,-0.126426408311032));
#45614=CARTESIAN_POINT('',(-0.0967681696808917,6.65845257773007E-5,-0.132223591688967));
#45615=CARTESIAN_POINT('',(-0.096675,-1.1839272930757E-17,-0.493));
#45616=CARTESIAN_POINT('Ctrl Pts',(-0.0967728733759203,6.44486977623322E-5,
-0.126426408311032));
#45617=CARTESIAN_POINT('Ctrl Pts',(-0.0968038274783861,0.0040844511009329,
-0.126691904969253));
#45618=CARTESIAN_POINT('Ctrl Pts',(-0.0965748568526,0.00810090112065628,
-0.126957401627474));
#45619=CARTESIAN_POINT('Ctrl Pts',(-0.0960740112983165,0.0120831576363327,
-0.127222898285695));
#45620=CARTESIAN_POINT('Ctrl Pts',(-0.0920950774891978,0.0437199265989198,
-0.129332118624319));
#45621=CARTESIAN_POINT('Ctrl Pts',(-0.0709570263862882,0.0731986063626649,
-0.131441338962943));
#45622=CARTESIAN_POINT('Ctrl Pts',(-0.0422695078882135,0.0871177779818565,
-0.133550559301567));
#45623=CARTESIAN_POINT('Ctrl Pts',(-0.0135819893901388,0.101036949601048,
-0.135659779640191));
#45624=CARTESIAN_POINT('Ctrl Pts',(0.0226549965031015,0.0993966130756864,
-0.137768999978815));
#45625=CARTESIAN_POINT('Ctrl Pts',(0.0499676102792677,0.0829424886199023,
-0.139878220317439));
#45626=CARTESIAN_POINT('Ctrl Pts',(0.0772802240554347,0.0664883641641178,
-0.141987440656063));
#45627=CARTESIAN_POINT('Ctrl Pts',(0.0956684657145276,0.0352204517779098,
-0.144096660994687));
#45628=CARTESIAN_POINT('Ctrl Pts',(0.0967727852795511,0.00335357950948155,
-0.146205881333311));
#45629=CARTESIAN_POINT('Ctrl Pts',(0.0978771048445746,-0.0285132927589462,
-0.148315101671935));
#45630=CARTESIAN_POINT('Ctrl Pts',(0.0816975023155301,-0.0609791249095938,
-0.150424322010559));
#45631=CARTESIAN_POINT('Ctrl Pts',(0.0555894498893144,-0.0792844975754325,
-0.152533542349183));
#45632=CARTESIAN_POINT('Ctrl Pts',(0.0294813974630983,-0.0975898702412715,
-0.154642762687807));
#45633=CARTESIAN_POINT('Ctrl Pts',(-0.00655510486028936,-0.1017347834223,
-0.156751983026431));
#45634=CARTESIAN_POINT('Ctrl Pts',(-0.0361373612697451,-0.0898349019422432,
-0.158861203365055));
#45635=CARTESIAN_POINT('Ctrl Pts',(-0.0657196176792,-0.0779350204621864,
-0.160970423703679));
#45636=CARTESIAN_POINT('Ctrl Pts',(-0.0888476281747239,-0.0499903443210447,
-0.163079644042303));
#45637=CARTESIAN_POINT('Ctrl Pts',(-0.0950070773142242,-0.0187049122841689,
-0.165188864380927));
#45638=CARTESIAN_POINT('Ctrl Pts',(-0.096211722897522,-0.0125862064273259,
-0.165601379024295));
#45639=CARTESIAN_POINT('Ctrl Pts',(-0.0967673159292923,-0.00633971565739204,
-0.166013893667664));
#45640=CARTESIAN_POINT('Ctrl Pts',(-0.0967106172141971,-8.32004823464877E-5,
-0.166426408311032));
#45641=CARTESIAN_POINT('Ctrl Pts',(-0.0967161166967018,-8.22460629427947E-5,
-0.172223591688967));
#45642=CARTESIAN_POINT('Ctrl Pts',(-0.0967708604363183,-0.00615259656181894,
-0.171823292808561));
#45643=CARTESIAN_POINT('Ctrl Pts',(-0.0962479502491979,-0.0122135489284046,
-0.171422993928155));
#45644=CARTESIAN_POINT('Ctrl Pts',(-0.0951131764843987,-0.0181576927593301,
-0.171022695047749));
#45645=CARTESIAN_POINT('Ctrl Pts',(-0.0891339244264755,-0.0494780628067843,
-0.168913474709125));
#45646=CARTESIAN_POINT('Ctrl Pts',(-0.066167161334334,-0.0775554120881626,
-0.166804254370501));
#45647=CARTESIAN_POINT('Ctrl Pts',(-0.0366538974200273,-0.0896253867579126,
-0.164695034031877));
#45648=CARTESIAN_POINT('Ctrl Pts',(-0.00714063350572054,-0.101695361427663,
-0.162585813693253));
#45649=CARTESIAN_POINT('Ctrl Pts',(0.0289191312307513,-0.0977579614857844,
-0.160476593354629));
#45650=CARTESIAN_POINT('Ctrl Pts',(0.0551321257213364,-0.0796031837461425,
-0.158367373016005));
#45651=CARTESIAN_POINT('Ctrl Pts',(0.0813451202119191,-0.0614484060065022,
-0.156258152677381));
#45652=CARTESIAN_POINT('Ctrl Pts',(0.097711344456617,-0.0290762504691009,
-0.154148932338757));
#45653=CARTESIAN_POINT('Ctrl Pts',(0.0967904851253458,0.00279645027672639,
-0.152039712000134));
#45654=CARTESIAN_POINT('Ctrl Pts',(0.0958696257940746,0.0346691510225565,
-0.14993049166151));
#45655=CARTESIAN_POINT('Ctrl Pts',(0.0776616828868309,0.0660423969768126,
-0.147821271322886));
#45656=CARTESIAN_POINT('Ctrl Pts',(0.0504442406332896,0.0826534738232335,
-0.145712050984262));
#45657=CARTESIAN_POINT('Ctrl Pts',(0.0232267983797483,0.0992645506696545,
-0.143602830645638));
#45658=CARTESIAN_POINT('Ctrl Pts',(-0.0130001432200904,0.10111345840824,
-0.141493610307013));
#45659=CARTESIAN_POINT('Ctrl Pts',(-0.0417673120207193,0.0873596577544192,
-0.139384389968389));
#45660=CARTESIAN_POINT('Ctrl Pts',(-0.0705344808213482,0.073605857100598,
-0.137275169629765));
#45661=CARTESIAN_POINT('Ctrl Pts',(-0.0918418768227671,0.0442493480543698,
-0.135165949291141));
#45662=CARTESIAN_POINT('Ctrl Pts',(-0.0960028615083386,0.0126360084708544,
-0.133056728952517));
#45663=CARTESIAN_POINT('Ctrl Pts',(-0.0965507213551153,0.00847360925790264,
-0.132779016531334));
#45664=CARTESIAN_POINT('Ctrl Pts',(-0.0968013325140246,0.0042720858280176,
-0.132501304110151));
#45665=CARTESIAN_POINT('Ctrl Pts',(-0.0967681696808917,6.65845257773007E-5,
-0.132223591688967));
#45666=CARTESIAN_POINT('Origin',(0.,0.,-0.493));
#45667=CARTESIAN_POINT('',(-0.0965260258856889,2.69457101370538E-5,-0.0864264083110318));
#45668=CARTESIAN_POINT('',(-0.0965245173086395,2.40562356700919E-5,-0.0922235916889671));
#45669=CARTESIAN_POINT('',(-0.096675,-1.1839272930757E-17,-0.493));
#45670=CARTESIAN_POINT('Ctrl Pts',(-0.0965260258856889,2.69457101370538E-5,
-0.0864264083110318));
#45671=CARTESIAN_POINT('Ctrl Pts',(-0.0965621452892423,0.0144064289818037,
-0.0873699162708424));
#45672=CARTESIAN_POINT('Ctrl Pts',(-0.0935513702939852,0.028771524918513,
-0.0883134242306529));
#45673=CARTESIAN_POINT('Ctrl Pts',(-0.0874164788557378,0.0416481827205965,
-0.0892569321904635));
#45674=CARTESIAN_POINT('Ctrl Pts',(-0.0737018751131272,0.0704340644370663,
-0.0913661525290875));
#45675=CARTESIAN_POINT('Ctrl Pts',(-0.0443745008367193,0.0917814772380087,
-0.0934753728677115));
#45676=CARTESIAN_POINT('Ctrl Pts',(-0.0127668769250902,0.0959855552481512,
-0.0955845932063354));
#45677=CARTESIAN_POINT('Ctrl Pts',(0.0188407469865399,0.100189633258294,
-0.0976938135449594));
#45678=CARTESIAN_POINT('Ctrl Pts',(0.0527286205333904,0.0872503764776352,
-0.0998030338835834));
#45679=CARTESIAN_POINT('Ctrl Pts',(0.0734907857447863,0.0630501695333001,
-0.101912254222207));
#45680=CARTESIAN_POINT('Ctrl Pts',(0.0942529509561815,0.0388499625889657,
-0.104021474560832));
#45681=CARTESIAN_POINT('Ctrl Pts',(0.101889407832122,0.00338880548095356,
-0.106130694899456));
#45682=CARTESIAN_POINT('Ctrl Pts',(0.0929285478197121,-0.027212175791531,
-0.10823991523808));
#45683=CARTESIAN_POINT('Ctrl Pts',(0.0839676878073023,-0.0578131570640146,
-0.110349135576704));
#45684=CARTESIAN_POINT('Ctrl Pts',(0.0584095109065445,-0.0835539625009726,
-0.112458355915327));
#45685=CARTESIAN_POINT('Ctrl Pts',(0.0278731037655201,-0.0927324585046492,
-0.114567576253951));
#45686=CARTESIAN_POINT('Ctrl Pts',(-0.00266330337550607,-0.101910954508326,
-0.116676796592575));
#45687=CARTESIAN_POINT('Ctrl Pts',(-0.0381779407567985,-0.0945271410787201,
-0.118786016931199));
#45688=CARTESIAN_POINT('Ctrl Pts',(-0.0625253511897811,-0.0739378052832015,
-0.120895237269823));
#45689=CARTESIAN_POINT('Ctrl Pts',(-0.0838080480942971,-0.0559401379580672,
-0.122738960950226));
#45690=CARTESIAN_POINT('Ctrl Pts',(-0.0965579146939385,-0.0278521875253081,
-0.124582684630629));
#45691=CARTESIAN_POINT('Ctrl Pts',(-0.0967728733759203,6.44486977623322E-5,
-0.126426408311032));
#45692=CARTESIAN_POINT('Ctrl Pts',(-0.0967681696808917,6.65845257773007E-5,
-0.132223591688967));
#45693=CARTESIAN_POINT('Ctrl Pts',(-0.096549461453191,-0.0276686132699799,
-0.130392083771527));
#45694=CARTESIAN_POINT('Ctrl Pts',(-0.0839883542531326,-0.0555768237062418,
-0.128560575854086));
#45695=CARTESIAN_POINT('Ctrl Pts',(-0.0629499367115576,-0.0735766513583343,
-0.126729067936645));
#45696=CARTESIAN_POINT('Ctrl Pts',(-0.0387214538594795,-0.094305801483208,
-0.124619847598021));
#45697=CARTESIAN_POINT('Ctrl Pts',(-0.00324991478559811,-0.101893931612153,
-0.122510627259397));
#45698=CARTESIAN_POINT('Ctrl Pts',(0.0273388238586198,-0.0928913715547443,
-0.120401406920773));
#45699=CARTESIAN_POINT('Ctrl Pts',(0.0579275625028361,-0.0838888114973365,
-0.118292186582149));
#45700=CARTESIAN_POINT('Ctrl Pts',(0.0836335007173896,-0.058295561253578,
-0.116182966243526));
#45701=CARTESIAN_POINT('Ctrl Pts',(0.0927703633790611,-0.0277466698065643,
-0.114073745904902));
#45702=CARTESIAN_POINT('Ctrl Pts',(0.101907226040733,0.00280222164045035,
-0.111964525566278));
#45703=CARTESIAN_POINT('Ctrl Pts',(0.0944750131495218,0.0383067542907205,
-0.109855305227654));
#45704=CARTESIAN_POINT('Ctrl Pts',(0.0738525078919995,0.0626260754898117,
-0.10774608488903));
#45705=CARTESIAN_POINT('Ctrl Pts',(0.0532300026344766,0.0869453966889036,
-0.105636864550406));
#45706=CARTESIAN_POINT('Ctrl Pts',(0.0194172050106418,0.100079506436816,
-0.103527644211782));
#45707=CARTESIAN_POINT('Ctrl Pts',(-0.0122141083892025,0.0960574515179389,
-0.101418423873158));
#45708=CARTESIAN_POINT('Ctrl Pts',(-0.043845421789046,0.0920353965990621,
-0.0993092035345336));
#45709=CARTESIAN_POINT('Ctrl Pts',(-0.073295250964899,0.0708571770133972,
-0.0971999831959097));
#45710=CARTESIAN_POINT('Ctrl Pts',(-0.0871753089182591,0.0421507139525716,
-0.0950907628572857));
#45711=CARTESIAN_POINT('Ctrl Pts',(-0.0934645999973232,0.0291433257524216,
-0.0941350391345129));
#45712=CARTESIAN_POINT('Ctrl Pts',(-0.0965571823799272,0.014590275702639,
-0.09317931541174));
#45713=CARTESIAN_POINT('Ctrl Pts',(-0.0965245173086395,2.40562356700919E-5,
-0.0922235916889671));
#45714=CARTESIAN_POINT('Origin',(0.,0.,-0.493));
#45715=CARTESIAN_POINT('',(-0.0966799176497682,-8.54770466914428E-5,-0.0464264083110319));
#45716=CARTESIAN_POINT('',(-0.0966824608565994,-8.60709826375376E-5,-0.0522235916889671));
#45717=CARTESIAN_POINT('',(-0.096675,-1.1839272930757E-17,-0.493));
#45718=CARTESIAN_POINT('Ctrl Pts',(-0.0966799176497682,-8.54770466914428E-5,
-0.0464264083110319));
#45719=CARTESIAN_POINT('Ctrl Pts',(-0.0964558808207423,0.0245299519874446,
-0.0480479275724319));
#45720=CARTESIAN_POINT('Ctrl Pts',(-0.0868711565580783,0.0492992357821797,
-0.0496694468338319));
#45721=CARTESIAN_POINT('Ctrl Pts',(-0.0699093451673916,0.066997198228178,
-0.051290966095232));
#45722=CARTESIAN_POINT('Ctrl Pts',(-0.0478459639811275,0.0900181411376509,
-0.0534001864338559));
#45723=CARTESIAN_POINT('Ctrl Pts',(-0.0133005709610127,0.101074427099992,
-0.05550940677248));
#45724=CARTESIAN_POINT('Ctrl Pts',(0.018027220984719,0.0951380919169941,
-0.0576186271111039));
#45725=CARTESIAN_POINT('Ctrl Pts',(0.0493550129304515,0.0892017567339961,
-0.0597278474497278));
#45726=CARTESIAN_POINT('Ctrl Pts',(0.0774652038018009,0.0662728004056583,
-0.0618370677883516));
#45727=CARTESIAN_POINT('Ctrl Pts',(0.0895757663479387,0.0367759010445744,
-0.0639462881269756));
#45728=CARTESIAN_POINT('Ctrl Pts',(0.101686328894077,0.00727900168348961,
-0.0660555084655996));
#45729=CARTESIAN_POINT('Ctrl Pts',(0.0977972631150027,-0.0287858407103417,
-0.0681647288042237));
#45730=CARTESIAN_POINT('Ctrl Pts',(0.0796780386229298,-0.0550234976588298,
-0.0702739491428478));
#45731=CARTESIAN_POINT('Ctrl Pts',(0.0615588141308575,-0.0812611546073171,
-0.0723831694814718));
#45732=CARTESIAN_POINT('Ctrl Pts',(0.0292094309257873,-0.0976716261104618,
-0.0744923898200957));
#45733=CARTESIAN_POINT('Ctrl Pts',(-0.00266439346619636,-0.0967942456364108,
-0.0766016101587197));
#45734=CARTESIAN_POINT('Ctrl Pts',(-0.0345382178581791,-0.0959168651623598,
-0.0787108304973436));
#45735=CARTESIAN_POINT('Ctrl Pts',(-0.0659364834370753,-0.0777516327111142,
-0.0808200508359675));
#45736=CARTESIAN_POINT('Ctrl Pts',(-0.0825846996221178,-0.0505568411694939,
-0.0829292711745914));
#45737=CARTESIAN_POINT('Ctrl Pts',(-0.0917857448314237,-0.0355269722843872,
-0.0840949835534049));
#45738=CARTESIAN_POINT('Ctrl Pts',(-0.0964814000450697,-0.0177390322834002,
-0.0852606959322183));
#45739=CARTESIAN_POINT('Ctrl Pts',(-0.0965260258856889,2.69457101370538E-5,
-0.0864264083110318));
#45740=CARTESIAN_POINT('Ctrl Pts',(-0.0965245173086395,2.40562356700919E-5,
-0.0922235916889671));
#45741=CARTESIAN_POINT('Ctrl Pts',(-0.0964850926838353,-0.0175564269735832,
-0.091070095073116));
#45742=CARTESIAN_POINT('Ctrl Pts',(-0.0918931431861939,-0.0351560939755392,
-0.0899165984572649));
#45743=CARTESIAN_POINT('Ctrl Pts',(-0.0828743072279342,-0.0500806183209312,
-0.0887631018414138));
#45744=CARTESIAN_POINT('Ctrl Pts',(-0.066382960853382,-0.0773707809976222,
-0.0866538815027898));
#45745=CARTESIAN_POINT('Ctrl Pts',(-0.0350899813734107,-0.0957163998150173,
-0.0845446611641659));
#45746=CARTESIAN_POINT('Ctrl Pts',(-0.00322164800733973,-0.0967772732126683,
-0.0824354408255419));
#45747=CARTESIAN_POINT('Ctrl Pts',(0.0286466853587313,-0.0978381466103194,
-0.080326220486918));
#45748=CARTESIAN_POINT('Ctrl Pts',(0.0610903726109036,-0.0816142745882247,
-0.0782170001482938));
#45749=CARTESIAN_POINT('Ctrl Pts',(0.079360166403506,-0.0554813080526386,
-0.0761077798096698));
#45750=CARTESIAN_POINT('Ctrl Pts',(0.0976299601961084,-0.0293483415170525,
-0.0739985594710458));
#45751=CARTESIAN_POINT('Ctrl Pts',(0.101725860529144,0.0066937195320257,
-0.0718893391324219));
#45752=CARTESIAN_POINT('Ctrl Pts',(0.0897856158264645,0.0362597525964753,
-0.0697801187937979));
#45753=CARTESIAN_POINT('Ctrl Pts',(0.0778453711237855,0.0658257856609249,
-0.0676708984551739));
#45754=CARTESIAN_POINT('Ctrl Pts',(0.0498689813853927,0.088915790740745,
-0.0655616781165499));
#45755=CARTESIAN_POINT('Ctrl Pts',(0.0185752788956987,0.0950325400363498,
-0.063452457777926));
#45756=CARTESIAN_POINT('Ctrl Pts',(-0.0127184235939963,0.101149289331955,
-0.0613432374393019));
#45757=CARTESIAN_POINT('Ctrl Pts',(-0.0473294388349918,0.090292782843343,
-0.0592340171006779));
#45758=CARTESIAN_POINT('Ctrl Pts',(-0.069523830713283,0.0673989000216935,
-0.0571247967620539));
#45759=CARTESIAN_POINT('Ctrl Pts',(-0.0867149011254147,0.0496660261609312,
-0.0554910617376916));
#45760=CARTESIAN_POINT('Ctrl Pts',(-0.0964565449248585,0.0247112571856237,
-0.0538573267133294));
#45761=CARTESIAN_POINT('Ctrl Pts',(-0.0966824608565994,-8.60709826375376E-5,
-0.0522235916889671));
#45762=CARTESIAN_POINT('Origin',(0.,0.,-1.05327725593024));
#45763=CARTESIAN_POINT('',(-0.0739037591343974,-6.53400956822213E-5,-0.0332772559302386));
#45764=CARTESIAN_POINT('',(-0.0740000552263865,4.36537410774818E-5,-0.0253727440697612));
#45765=CARTESIAN_POINT('',(-0.0739,6.54188504088864E-16,-1.05327725593024));
#45766=CARTESIAN_POINT('',(0.0740154662741573,-0.000526981588894721,-0.0133250000000002));
#45767=CARTESIAN_POINT('Ctrl Pts',(-0.0739037591343974,-6.53400956822266E-5,
-0.0332772559302386));
#45768=CARTESIAN_POINT('Ctrl Pts',(-0.0739552679160763,-0.00572472549920979,
-0.0327895548530145));
#45769=CARTESIAN_POINT('Ctrl Pts',(-0.0707828206579678,-0.0358032940414331,
-0.0301926334371664));
#45770=CARTESIAN_POINT('Ctrl Pts',(-0.0296542637309572,-0.082043730023256,
-0.0254864916826941));
#45771=CARTESIAN_POINT('Ctrl Pts',(0.0504128653233092,-0.0699260839861745,
-0.0193234407831724));
#45772=CARTESIAN_POINT('Ctrl Pts',(0.0737279762021362,-0.0230151521843795,
-0.0152696102222742));
#45773=CARTESIAN_POINT('Ctrl Pts',(0.0740154662741573,-0.000526981588894725,
-0.0133250000000001));
#45774=CARTESIAN_POINT('',(0.0233628051714152,-0.0701098376443883,-0.013325));
#45775=CARTESIAN_POINT('Origin',(0.,0.,-0.013325));
#45776=CARTESIAN_POINT('Ctrl Pts',(-0.0740000552263865,4.36537410774818E-5,
-0.0253727440697612));
#45777=CARTESIAN_POINT('Ctrl Pts',(-0.073837658281225,-0.022021592300188,
-0.0234660497184648));
#45778=CARTESIAN_POINT('Ctrl Pts',(-0.0516098552235117,-0.0687718438380149,
-0.0194501350285445));
#45779=CARTESIAN_POINT('Ctrl Pts',(0.00013432532901024,-0.0778502984302035,
-0.015434220338624));
#45780=CARTESIAN_POINT('Ctrl Pts',(0.0233628051714152,-0.0701098376443883,
-0.013325));
#45781=CARTESIAN_POINT('Origin',(0.,0.,-1.05327725593024));
#45782=CARTESIAN_POINT('',(-0.0737861216752254,2.05977551544039E-5,-0.0732772559302385));
#45783=CARTESIAN_POINT('',(-0.0739057032045792,-6.57941103356097E-5,-0.0653727440697609));
#45784=CARTESIAN_POINT('',(-0.0739,6.54188504088864E-16,-1.05327725593024));
#45785=CARTESIAN_POINT('Ctrl Pts',(-0.0737861216752254,2.05977551544058E-5,
-0.0732772559302385));
#45786=CARTESIAN_POINT('Ctrl Pts',(-0.0737520089302376,-0.0135600153684295,
-0.072111543551425));
#45787=CARTESIAN_POINT('Ctrl Pts',(-0.0636679022392886,-0.0517603253615703,
-0.0688366108339875));
#45788=CARTESIAN_POINT('Ctrl Pts',(-0.00240023246381204,-0.0872062789102198,
-0.0634524577779261));
#45789=CARTESIAN_POINT('Ctrl Pts',(0.071785009393588,-0.0495729555872598,
-0.057124796762054));
#45790=CARTESIAN_POINT('Ctrl Pts',(0.0807036117542888,0.033132765216591,
-0.050797135746182));
#45791=CARTESIAN_POINT('Ctrl Pts',(0.0162399001827532,0.0857146076576825,
-0.0444694747303104));
#45792=CARTESIAN_POINT('Ctrl Pts',(-0.0568754076960062,0.0623139836826857,
-0.0386295147916622));
#45793=CARTESIAN_POINT('Ctrl Pts',(-0.0737325016048901,0.0187511088892927,
-0.0348987751916385));
#45794=CARTESIAN_POINT('Ctrl Pts',(-0.0739037591343974,-6.53400956822266E-5,
-0.0332772559302386));
#45795=CARTESIAN_POINT('Ctrl Pts',(-0.0739057032045792,-6.57941103356053E-5,
-0.0653727440697609));
#45796=CARTESIAN_POINT('Ctrl Pts',(-0.0739559643758101,-0.00558263724541527,
-0.0648972587554992));
#45797=CARTESIAN_POINT('Ctrl Pts',(-0.070879856117806,-0.0355164036035382,
-0.0623125531026135));
#45798=CARTESIAN_POINT('Ctrl Pts',(-0.0301398485007547,-0.0818676840127184,
-0.0576186271111039));
#45799=CARTESIAN_POINT('Ctrl Pts',(0.0521761247033908,-0.0699113944796167,
-0.0512909660952318));
#45800=CARTESIAN_POINT('Ctrl Pts',(0.0870667295313287,0.00560289368117736,
-0.04496330507936));
#45801=CARTESIAN_POINT('Ctrl Pts',(0.0427661024466595,0.0760368969037317,
-0.0386356440634878));
#45802=CARTESIAN_POINT('Ctrl Pts',(-0.0403659317628278,0.0773093583706435,
-0.032307983047616));
#45803=CARTESIAN_POINT('Ctrl Pts',(-0.0728760131951745,0.0291232266081595,
-0.0278870163830404));
#45804=CARTESIAN_POINT('Ctrl Pts',(-0.074017304767004,0.00238738845508473,
-0.0255752700570888));
#45805=CARTESIAN_POINT('Ctrl Pts',(-0.0740000552263865,4.36537410774818E-5,
-0.0253727440697612));
#45806=CARTESIAN_POINT('Origin',(0.,0.,-1.05327725593024));
#45807=CARTESIAN_POINT('',(-0.0739748160587588,4.92656712164654E-5,-0.113277255930238));
#45808=CARTESIAN_POINT('',(-0.0737849684934933,1.83889921493083E-5,-0.105372744069761));
#45809=CARTESIAN_POINT('',(-0.0739,6.54188504088864E-16,-1.05327725593024));
#45810=CARTESIAN_POINT('Ctrl Pts',(-0.0739748160587588,4.92656712164654E-5,
-0.113277255930238));
#45811=CARTESIAN_POINT('Ctrl Pts',(-0.0738104980179169,-0.0212906817493676,
-0.111433532249835));
#45812=CARTESIAN_POINT('Ctrl Pts',(-0.0529146149777968,-0.0673243027675011,
-0.107480588230809));
#45813=CARTESIAN_POINT('Ctrl Pts',(0.0251121136077328,-0.0835467633888102,
-0.101418423873158));
#45814=CARTESIAN_POINT('Ctrl Pts',(0.0837234176563311,-0.0245166463433077,
-0.0950907628572859));
#45815=CARTESIAN_POINT('Ctrl Pts',(0.0662111084823356,0.0568046728275819,
-0.0887631018414139));
#45816=CARTESIAN_POINT('Ctrl Pts',(-0.0115022772465146,0.0864776309684878,
-0.0824354408255419));
#45817=CARTESIAN_POINT('Ctrl Pts',(-0.0663672499855129,0.0465413853866943,
-0.0772734921884835));
#45818=CARTESIAN_POINT('Ctrl Pts',(-0.0738137319562963,0.0110125172149529,
-0.074220763890049));
#45819=CARTESIAN_POINT('Ctrl Pts',(-0.0737861216752254,2.05977551544058E-5,
-0.0732772559302385));
#45820=CARTESIAN_POINT('Ctrl Pts',(-0.0737849684934933,1.83889921493057E-5,
-0.105372744069761));
#45821=CARTESIAN_POINT('Ctrl Pts',(-0.0737548316455695,-0.0134204287907709,
-0.10421924745391));
#45822=CARTESIAN_POINT('Ctrl Pts',(-0.0638261762896611,-0.0514742070674987,
-0.100956530499435));
#45823=CARTESIAN_POINT('Ctrl Pts',(-0.00290249226713311,-0.0871909301984517,
-0.0955845932063355));
#45824=CARTESIAN_POINT('Ctrl Pts',(0.0714990124011491,-0.0499855262439841,
-0.0892569321904637));
#45825=CARTESIAN_POINT('Ctrl Pts',(0.0808919382230671,0.032667951227759,
-0.0829292711745915));
#45826=CARTESIAN_POINT('Ctrl Pts',(0.0167350661775352,0.0856191188118938,
-0.0766016101587197));
#45827=CARTESIAN_POINT('Ctrl Pts',(-0.0566723609033016,0.0625932640986974,
-0.0707494344571094));
#45828=CARTESIAN_POINT('Ctrl Pts',(-0.0737330092572742,0.0188897016396973,
-0.0670064790941231));
#45829=CARTESIAN_POINT('Ctrl Pts',(-0.0739057032045792,-6.57941103356053E-5,
-0.0653727440697609));
#45830=CARTESIAN_POINT('Origin',(0.,0.,-1.05327725593024));
#45831=CARTESIAN_POINT('',(-0.0739272263990603,-6.35998515147437E-5,-0.153277255930238));
#45832=CARTESIAN_POINT('',(-0.0739712204749718,5.0898334158311E-5,-0.145372744069761));
#45833=CARTESIAN_POINT('',(-0.0739,6.54188504088864E-16,-1.05327725593024));
#45834=CARTESIAN_POINT('Ctrl Pts',(-0.0739272263990603,-6.35998515147395E-5,
-0.153277255930238));
#45835=CARTESIAN_POINT('Ctrl Pts',(-0.0739705678528545,-0.00484618554001679,
-0.15286474128687));
#45836=CARTESIAN_POINT('Ctrl Pts',(-0.0713743141958555,-0.0340356706082163,
-0.150343006304878));
#45837=CARTESIAN_POINT('Ctrl Pts',(-0.0325577426519127,-0.0809362252804344,
-0.145712050984262));
#45838=CARTESIAN_POINT('Ctrl Pts',(0.0500829872689032,-0.0714309007163379,
-0.139384389968389));
#45839=CARTESIAN_POINT('Ctrl Pts',(0.0871868701826791,0.00302138775326442,
-0.133056728952518));
#45840=CARTESIAN_POINT('Ctrl Pts',(0.0450180242988335,0.0747265460260562,
-0.126729067936645));
#45841=CARTESIAN_POINT('Ctrl Pts',(-0.0380824646851997,0.0784882487172661,
-0.120401406920774));
#45842=CARTESIAN_POINT('Ctrl Pts',(-0.0724329427199956,0.0305837973187204,
-0.115917469585305));
#45843=CARTESIAN_POINT('Ctrl Pts',(-0.0739984778965888,0.00312222328791404,
-0.113542752588459));
#45844=CARTESIAN_POINT('Ctrl Pts',(-0.0739748160587588,4.92656712164654E-5,
-0.113277255930238));
#45845=CARTESIAN_POINT('Ctrl Pts',(-0.0739712204749718,5.08983341583136E-5,
-0.145372744069761));
#45846=CARTESIAN_POINT('Ctrl Pts',(-0.0738040362181614,-0.0211503544934227,
-0.14354123615232));
#45847=CARTESIAN_POINT('Ctrl Pts',(-0.0531442479111094,-0.067052177514178,
-0.139600507896256));
#45848=CARTESIAN_POINT('Ctrl Pts',(0.0246307528823777,-0.083689933929838,
-0.133550559301567));
#45849=CARTESIAN_POINT('Ctrl Pts',(0.0835809106498128,-0.0249981979169972,
-0.127222898285695));
#45850=CARTESIAN_POINT('Ctrl Pts',(0.0665369841126368,0.0564225922414199,
-0.120895237269823));
#45851=CARTESIAN_POINT('Ctrl Pts',(-0.0110042337120753,0.0865423970628537,
-0.114567576253952));
#45852=CARTESIAN_POINT('Ctrl Pts',(-0.0662286724539735,0.0468289140681891,
-0.10939341185393));
#45853=CARTESIAN_POINT('Ctrl Pts',(-0.0738099382247387,0.0111530527481255,
-0.106328467792534));
#45854=CARTESIAN_POINT('Ctrl Pts',(-0.0737849684934933,1.83889921493057E-5,
-0.105372744069761));
#45855=CARTESIAN_POINT('Origin',(0.,0.,-1.05327725593024));
#45856=CARTESIAN_POINT('',(-0.0737812135695977,6.75269259391766E-6,-0.193277255930238));
#45857=CARTESIAN_POINT('',(-0.0739314302962117,-6.28702772325351E-5,-0.185372744069761));
#45858=CARTESIAN_POINT('',(-0.0739,6.54188504088864E-16,-1.05327725593024));
#45859=CARTESIAN_POINT('Ctrl Pts',(-0.0737812135695977,6.75269259391761E-6,
-0.193277255930238));
#45860=CARTESIAN_POINT('Ctrl Pts',(-0.0737707790832793,-0.0127000412597446,
-0.192186729985281));
#45861=CARTESIAN_POINT('Ctrl Pts',(-0.0646238781142857,-0.0499975205142205,
-0.188986983701699));
#45862=CARTESIAN_POINT('Ctrl Pts',(-0.00548820489699097,-0.0870664043988389,
-0.183678017079493));
#45863=CARTESIAN_POINT('Ctrl Pts',(0.0699845600316936,-0.0520849356893883,
-0.177350356063621));
#45864=CARTESIAN_POINT('Ctrl Pts',(0.0818254144363875,0.0302536067170679,
-0.17102269504775));
#45865=CARTESIAN_POINT('Ctrl Pts',(0.0192683238503164,0.0850847275592565,
-0.164695034031877));
#45866=CARTESIAN_POINT('Ctrl Pts',(-0.05558770111295,0.064023245622808,
-0.158779887659374));
#45867=CARTESIAN_POINT('Ctrl Pts',(-0.0737489595358703,0.0196075572969276,
-0.154973961625494));
#45868=CARTESIAN_POINT('Ctrl Pts',(-0.0739272263990603,-6.35998515147395E-5,
-0.153277255930238));
#45869=CARTESIAN_POINT('Ctrl Pts',(-0.0739314302962117,-6.2870277232539E-5,
-0.185372744069761));
#45870=CARTESIAN_POINT('Ctrl Pts',(-0.0739732773337877,-0.00470314854841896,
-0.184972445189355));
#45871=CARTESIAN_POINT('Ctrl Pts',(-0.0714673786331718,-0.0337485430234499,
-0.182462925970325));
#45872=CARTESIAN_POINT('Ctrl Pts',(-0.0330231128016351,-0.0807474638242463,
-0.177844186412671));
#45873=CARTESIAN_POINT('Ctrl Pts',(0.0496709636615209,-0.0717180191165734,
-0.171516525396799));
#45874=CARTESIAN_POINT('Ctrl Pts',(0.0872028169333057,0.00251944540519899,
-0.165188864380927));
#45875=CARTESIAN_POINT('Ctrl Pts',(0.0454474412670434,0.0744661599442045,
-0.158861203365055));
#45876=CARTESIAN_POINT('Ctrl Pts',(-0.0376300136353005,0.078706168691497,
-0.152533542349183));
#45877=CARTESIAN_POINT('Ctrl Pts',(-0.0723500183551033,0.030870284260848,
-0.148037389250752));
#45878=CARTESIAN_POINT('Ctrl Pts',(-0.0739965707037644,0.00326565443693249,
-0.145650456490944));
#45879=CARTESIAN_POINT('Ctrl Pts',(-0.0739712204749718,5.08983341583136E-5,
-0.145372744069761));
#45880=CARTESIAN_POINT('Origin',(0.,0.,-1.05327725593024));
#45881=CARTESIAN_POINT('',(-0.0739514724689521,5.80827170926923E-5,-0.233277255930238));
#45882=CARTESIAN_POINT('',(-0.0737808888395284,4.46017856624292E-6,-0.22537274406976));
#45883=CARTESIAN_POINT('',(-0.0739,6.54188504088864E-16,-1.05327725593024));
#45884=CARTESIAN_POINT('Ctrl Pts',(-0.0739514724689521,5.808271709269E-5,
-0.233277255930238));
#45885=CARTESIAN_POINT('Ctrl Pts',(-0.0737747026266549,-0.0204284806437574,
-0.231508718683691));
#45886=CARTESIAN_POINT('Ctrl Pts',(-0.0543062576718298,-0.0656429917484751,
-0.22763096109852));
#45887=CARTESIAN_POINT('Ctrl Pts',(0.0221368387963713,-0.0843838819687206,
-0.221643983174725));
#45888=CARTESIAN_POINT('Ctrl Pts',(0.0828024243326025,-0.0274670291926198,
-0.215316322158853));
#45889=CARTESIAN_POINT('Ctrl Pts',(0.0681817402553036,0.0544236112708011,
-0.208988661142981));
#45890=CARTESIAN_POINT('Ctrl Pts',(-0.00843168039820402,0.0868307890880593,
-0.202661000127109));
#45891=CARTESIAN_POINT('Ctrl Pts',(-0.0654962553541143,0.048310132439586,
-0.197423865056195));
#45892=CARTESIAN_POINT('Ctrl Pts',(-0.0737909607496282,0.0118765663550488,
-0.194295950323905));
#45893=CARTESIAN_POINT('Ctrl Pts',(-0.0737812135695977,6.75269259391761E-6,
-0.193277255930238));
#45894=CARTESIAN_POINT('Ctrl Pts',(-0.0737808888395284,4.46017856623859E-6,
-0.22537274406976));
#45895=CARTESIAN_POINT('Ctrl Pts',(-0.0737740757179536,-0.0125601331883079,
-0.224294433887765));
#45896=CARTESIAN_POINT('Ctrl Pts',(-0.0647750414269508,-0.0497107593494358,
-0.221106903367146));
#45897=CARTESIAN_POINT('Ctrl Pts',(-0.00598931255869429,-0.0870333673276597,
-0.215810152507903));
#45898=CARTESIAN_POINT('Ctrl Pts',(0.0696835717087142,-0.0524869386356467,
-0.209482491492031));
#45899=CARTESIAN_POINT('Ctrl Pts',(0.0819982124259003,0.0297820760219009,
-0.203154830476159));
#45900=CARTESIAN_POINT('Ctrl Pts',(0.0197577953896086,0.0849723979572207,
-0.196827169460287));
#45901=CARTESIAN_POINT('Ctrl Pts',(-0.0553730665477232,0.0642995700232107,
-0.190899807324821));
#45902=CARTESIAN_POINT('Ctrl Pts',(-0.0737527805323053,0.0197470055377898,
-0.187081665527979));
#45903=CARTESIAN_POINT('Ctrl Pts',(-0.0739314302962117,-6.2870277232539E-5,
-0.185372744069761));
#45904=CARTESIAN_POINT('Origin',(0.,0.,-1.05327725593024));
#45905=CARTESIAN_POINT('',(-0.0739525682181994,-5.77538386566367E-5,-0.273277255930238));
#45906=CARTESIAN_POINT('',(-0.0739474476707976,5.92274223705867E-5,-0.265372744069761));
#45907=CARTESIAN_POINT('',(-0.0739,6.54188504088864E-16,-1.05327725593024));
#45908=CARTESIAN_POINT('Ctrl Pts',(-0.0739525682181994,-5.77538386566322E-5,
-0.273277255930238));
#45909=CARTESIAN_POINT('Ctrl Pts',(-0.0739861634225736,-0.0039651806039843,
-0.272939927720726));
#45910=CARTESIAN_POINT('Ctrl Pts',(-0.0719323350430627,-0.0322692975822643,
-0.270493379172589));
#45911=CARTESIAN_POINT('Ctrl Pts',(-0.0354043422207423,-0.0797321247674219,
-0.265937610285828));
#45912=CARTESIAN_POINT('Ctrl Pts',(0.0475212323275497,-0.0731601780074524,
-0.259609949269957));
#45913=CARTESIAN_POINT('Ctrl Pts',(0.0872391793431545,-6.89604553678452E-5,
-0.253282288254085));
#45914=CARTESIAN_POINT('Ctrl Pts',(0.0476368355604161,0.0730849578627569,
-0.246954627238213));
#45915=CARTESIAN_POINT('Ctrl Pts',(-0.035278245432985,0.0797879976386212,
-0.240626966222341));
#45916=CARTESIAN_POINT('Ctrl Pts',(-0.0719081835391686,0.0323480695112505,
-0.236067842453016));
#45917=CARTESIAN_POINT('Ctrl Pts',(-0.0739855246194383,0.00400452250253258,
-0.233617939022315));
#45918=CARTESIAN_POINT('Ctrl Pts',(-0.0739514724689521,5.808271709269E-5,
-0.233277255930238));
#45919=CARTESIAN_POINT('Ctrl Pts',(-0.0739474476707976,5.92274223705815E-5,
-0.265372744069761));
#45920=CARTESIAN_POINT('Ctrl Pts',(-0.0737697580626393,-0.0202887024690249,
-0.263616422586176));
#45921=CARTESIAN_POINT('Ctrl Pts',(-0.0545274805569218,-0.0653684243106095,
-0.259750880763967));
#45922=CARTESIAN_POINT('Ctrl Pts',(0.0216507148888523,-0.0845099132536343,
-0.253776118603134));
#45923=CARTESIAN_POINT('Ctrl Pts',(0.0826429366480972,-0.0279432266482656,
-0.247448457587263));
#45924=CARTESIAN_POINT('Ctrl Pts',(0.0684938994372912,0.0540302196294675,
-0.241120796571391));
#45925=CARTESIAN_POINT('Ctrl Pts',(-0.00793169816963801,0.0868778858943854,
-0.234793135555519));
#45926=CARTESIAN_POINT('Ctrl Pts',(-0.065350690899438,0.0485972782324374,
-0.229543784721642));
#45927=CARTESIAN_POINT('Ctrl Pts',(-0.073787402472013,0.0120167430375237,
-0.226403654226389));
#45928=CARTESIAN_POINT('Ctrl Pts',(-0.0737808888395284,4.46017856623859E-6,
-0.22537274406976));
#45929=CARTESIAN_POINT('Origin',(0.,0.,-1.05327725593024));
#45930=CARTESIAN_POINT('',(-0.0737813255293768,-7.38103354979496E-6,-0.313277255930238));
#45931=CARTESIAN_POINT('',(-0.0739565202301569,-5.65040446714252E-5,-0.305372744069761));
#45932=CARTESIAN_POINT('',(-0.0739,6.54188504088864E-16,-1.05327725593024));
#45933=CARTESIAN_POINT('Ctrl Pts',(-0.0737813255293768,-7.38103354979737E-6,
-0.313277255930238));
#45934=CARTESIAN_POINT('Ctrl Pts',(-0.0737919455150245,-0.011838058808532,
-0.312261916419136));
#45935=CARTESIAN_POINT('Ctrl Pts',(-0.0655360332068969,-0.0482312596297118,
-0.30913735656941));
#45936=CARTESIAN_POINT('Ctrl Pts',(-0.00856894504114455,-0.0868173505060656,
-0.303903576381061));
#45937=CARTESIAN_POINT('Ctrl Pts',(0.0680956140128458,-0.0545313352140282,
-0.297575915365189));
#45938=CARTESIAN_POINT('Ctrl Pts',(0.0828457448677347,0.0273360883324843,
-0.291248254349316));
#45939=CARTESIAN_POINT('Ctrl Pts',(0.0222702178726658,0.0843487792674867,
-0.284920593333445));
#45940=CARTESIAN_POINT('Ctrl Pts',(-0.0542452639373956,0.0657183312475859,
-0.278930260527085));
#45941=CARTESIAN_POINT('Ctrl Pts',(-0.0737761018672454,0.0204668822140799,
-0.27504914805935));
#45942=CARTESIAN_POINT('Ctrl Pts',(-0.0739525682181994,-5.77538386566322E-5,
-0.273277255930238));
#45943=CARTESIAN_POINT('Ctrl Pts',(-0.0739565202301568,-5.6504044671423E-5,
-0.305372744069761));
#45944=CARTESIAN_POINT('Ctrl Pts',(-0.0739884412181998,-0.00382190668348843,
-0.305047631623211));
#45945=CARTESIAN_POINT('Ctrl Pts',(-0.0720196891488213,-0.0319825108223484,
-0.302613298838036));
#45946=CARTESIAN_POINT('Ctrl Pts',(-0.0358627338085138,-0.0795269967816936,
-0.298069745714238));
#45947=CARTESIAN_POINT('Ctrl Pts',(0.0470992967446723,-0.0734325209937202,
-0.291742084698366));
#45948=CARTESIAN_POINT('Ctrl Pts',(0.0872373353447779,-0.000571152587860333,
-0.285414423682494));
#45949=CARTESIAN_POINT('Ctrl Pts',(0.0480567597612106,0.0728095236530848,
-0.279086762666623));
#45950=CARTESIAN_POINT('Ctrl Pts',(-0.0348183598080465,0.0799897538039288,
-0.27275910165075));
#45951=CARTESIAN_POINT('Ctrl Pts',(-0.0718196555148094,0.032634929251857,
-0.268187762118463));
#45952=CARTESIAN_POINT('Ctrl Pts',(-0.0739831509630807,0.00414775063876829,
-0.2657256429248));
#45953=CARTESIAN_POINT('Ctrl Pts',(-0.0739474476707976,5.92274223705815E-5,
-0.265372744069761));
#45954=CARTESIAN_POINT('Origin',(0.,0.,-1.05327725593024));
#45955=CARTESIAN_POINT('',(-0.0739260676437687,6.37850448278505E-5,-0.353277255930238));
#45956=CARTESIAN_POINT('',(-0.0737818159558278,-9.66304559187059E-6,-0.345372744069761));
#45957=CARTESIAN_POINT('',(-0.0739,6.54188504088864E-16,-1.05327725593024));
#45958=CARTESIAN_POINT('Ctrl Pts',(-0.0739260676437687,6.37850448278517E-5,
-0.353277255930238));
#45959=CARTESIAN_POINT('Ctrl Pts',(-0.0737479485415012,-0.0195692698142952,
-0.351583905117547));
#45960=CARTESIAN_POINT('Ctrl Pts',(-0.0556464121921038,-0.0639472967095582,
-0.347781333966231));
#45961=CARTESIAN_POINT('Ctrl Pts',(0.019133785015476,-0.0851150834987123,
-0.341869542476292));
#45962=CARTESIAN_POINT('Ctrl Pts',(0.0817774827305826,-0.030382930837239,
-0.33554188146042));
#45963=CARTESIAN_POINT('Ctrl Pts',(0.0700668162737063,0.0519742284721753,
-0.329214220444548));
#45964=CARTESIAN_POINT('Ctrl Pts',(-0.00535055036065351,0.0870749721725439,
-0.322886559428676));
#45965=CARTESIAN_POINT('Ctrl Pts',(-0.0645821602000743,0.0500762594422092,
-0.317574237923906));
#45966=CARTESIAN_POINT('Ctrl Pts',(-0.0737698840375787,0.012738455657667,
-0.31437113675776));
#45967=CARTESIAN_POINT('Ctrl Pts',(-0.0737813255293768,-7.38103354979737E-6,
-0.313277255930238));
#45968=CARTESIAN_POINT('Ctrl Pts',(-0.0737818159558278,-9.6630455918784E-6,
-0.345372744069761));
#45969=CARTESIAN_POINT('Ctrl Pts',(-0.0737955572724641,-0.0116978086519519,
-0.344369620321621));
#45970=CARTESIAN_POINT('Ctrl Pts',(-0.0656801480854143,-0.0479440254684255,
-0.341257276234857));
#45971=CARTESIAN_POINT('Ctrl Pts',(-0.00906856792307098,-0.086766583251621,
-0.33603571180947));
#45972=CARTESIAN_POINT('Ctrl Pts',(0.0677805742992985,-0.0549224238448479,
-0.329708050793598));
#45973=CARTESIAN_POINT('Ctrl Pts',(0.0830017312015545,0.0268587324883495,
-0.323380389777726));
#45974=CARTESIAN_POINT('Ctrl Pts',(0.0227554031361251,0.0842191814342093,
-0.317052728761854));
#45975=CARTESIAN_POINT('Ctrl Pts',(-0.0540223059082473,0.0659924114034696,
-0.311050180192533));
#45976=CARTESIAN_POINT('Ctrl Pts',(-0.0737813485709526,0.0206067607304377,
-0.307156851961835));
#45977=CARTESIAN_POINT('Ctrl Pts',(-0.0739565202301568,-5.6504044671423E-5,
-0.305372744069761));
#45978=CARTESIAN_POINT('Origin',(0.,0.,-1.05327725593024));
#45979=CARTESIAN_POINT('',(-0.0739757877607653,-4.88044159986755E-5,-0.393277255930238));
#45980=CARTESIAN_POINT('',(-0.0739218355690636,6.44039839332328E-5,-0.385372744069761));
#45981=CARTESIAN_POINT('',(-0.0739,6.54188504088864E-16,-1.05327725593024));
#45982=CARTESIAN_POINT('Ctrl Pts',(-0.0739757877607652,-4.88044159986777E-5,
-0.393277255930238));
#45983=CARTESIAN_POINT('Ctrl Pts',(-0.0739989879633844,-0.00308282705743824,
-0.393015114154581));
#45984=CARTESIAN_POINT('Ctrl Pts',(-0.0724555604706598,-0.0305051292578985,
-0.390643752040301));
#45985=CARTESIAN_POINT('Ctrl Pts',(-0.0382065020487046,-0.0784279438032996,
-0.386163169587396));
#45986=CARTESIAN_POINT('Ctrl Pts',(0.0448998284991146,-0.0747976240850022,
-0.379835508571524));
#45987=CARTESIAN_POINT('Ctrl Pts',(0.0871819848609725,-0.00315922201061306,
-0.373507847555652));
#45988=CARTESIAN_POINT('Ctrl Pts',(0.0501958532401191,0.0713516326758373,
-0.36718018653978));
#45989=CARTESIAN_POINT('Ctrl Pts',(-0.0324297457147349,0.0809875963397409,
-0.360852525523908));
#45990=CARTESIAN_POINT('Ctrl Pts',(-0.0713485905353685,0.0341145348533431,
-0.356218215320728));
#45991=CARTESIAN_POINT('Ctrl Pts',(-0.0739698118614845,0.00488546118876761,
-0.353693125456171));
#45992=CARTESIAN_POINT('Ctrl Pts',(-0.0739260676437687,6.37850448278517E-5,
-0.353277255930238));
#45993=CARTESIAN_POINT('Ctrl Pts',(-0.0739218355690636,6.44039839332311E-5,
-0.385372744069761));
#45994=CARTESIAN_POINT('Ctrl Pts',(-0.0737444054695453,-0.019429892336047,
-0.383691609020032));
#45995=CARTESIAN_POINT('Ctrl Pts',(-0.0558593356375793,-0.0636705354435064,
-0.379901253631678));
#45996=CARTESIAN_POINT('Ctrl Pts',(0.0186435017497599,-0.0852238155437934,
-0.374001677904702));
#45997=CARTESIAN_POINT('Ctrl Pts',(0.0816012266274847,-0.0308531798397786,
-0.367674016888829));
#45998=CARTESIAN_POINT('Ctrl Pts',(0.0703648442895387,0.0515700259981008,
-0.361346355872959));
#45999=CARTESIAN_POINT('Ctrl Pts',(-0.0048492135956714,0.0871043283702904,
-0.355018694857085));
#46000=CARTESIAN_POINT('Ctrl Pts',(-0.0644295159300822,0.0503629031102395,
-0.349694157589354));
#46001=CARTESIAN_POINT('Ctrl Pts',(-0.0737666640630444,0.0128782962199111,
-0.346478840660245));
#46002=CARTESIAN_POINT('Ctrl Pts',(-0.0737818159558278,-9.6630455918784E-6,
-0.345372744069761));
#46003=CARTESIAN_POINT('Origin',(0.,0.,-1.05327725593024));
#46004=CARTESIAN_POINT('',(-0.0737864256067439,-2.11896062283324E-5,-0.433277255930238));
#46005=CARTESIAN_POINT('',(-0.0739792630123745,-4.70781898877851E-5,-0.425372744069761));
#46006=CARTESIAN_POINT('',(-0.0739,6.54188504088864E-16,-1.05327725593024));
#46007=CARTESIAN_POINT('Ctrl Pts',(-0.0737864256067439,-2.11896062283414E-5,
-0.433277255930238));
#46008=CARTESIAN_POINT('Ctrl Pts',(-0.0738147678314805,-0.0109739073698394,
-0.432337102852992));
#46009=CARTESIAN_POINT('Ctrl Pts',(-0.0664051981588223,-0.0464624370744622,
-0.429287729437122));
#46010=CARTESIAN_POINT('Ctrl Pts',(-0.0116389293761198,-0.0864593227534712,
-0.424129135682628));
#46011=CARTESIAN_POINT('Ctrl Pts',(0.0661211938172418,-0.0569092865549545,
-0.417801474666756));
#46012=CARTESIAN_POINT('Ctrl Pts',(0.0837620866257479,0.0243842574648459,
-0.411473813650883));
#46013=CARTESIAN_POINT('Ctrl Pts',(0.0252441581448469,0.0835069556837582,
-0.405146152635012));
#46014=CARTESIAN_POINT('Ctrl Pts',(-0.0528513042080767,0.0673989656330345,
-0.399080633394796));
#46015=CARTESIAN_POINT('Ctrl Pts',(-0.0738123166894069,0.0213292386926207,
-0.395124334493205));
#46016=CARTESIAN_POINT('Ctrl Pts',(-0.0739757877607652,-4.88044159986777E-5,
-0.393277255930238));
#46017=CARTESIAN_POINT('Ctrl Pts',(-0.0739792630123745,-4.70781898877872E-5,
-0.425372744069761));
#46018=CARTESIAN_POINT('Ctrl Pts',(-0.0740007916035247,-0.00293935953098124,
-0.425122818057066));
#46019=CARTESIAN_POINT('Ctrl Pts',(-0.0725373395423451,-0.0302187231335646,
-0.422763671705748));
#46020=CARTESIAN_POINT('Ctrl Pts',(-0.0386573396255769,-0.078206706786622,
-0.418295305015806));
#46021=CARTESIAN_POINT('Ctrl Pts',(0.0444685104211786,-0.0750548497717326,
-0.411967643999933));
#46022=CARTESIAN_POINT('Ctrl Pts',(0.0871623526873201,-0.00366103364462123,
-0.405639982984062));
#46023=CARTESIAN_POINT('Ctrl Pts',(0.0506057570896398,0.0710614962037825,
-0.399312321968189));
#46024=CARTESIAN_POINT('Ctrl Pts',(-0.0319630018346919,0.081172935188099,
-0.392984660952318));
#46025=CARTESIAN_POINT('Ctrl Pts',(-0.0712543236721827,0.03440172595574,
-0.388338134986175));
#46026=CARTESIAN_POINT('Ctrl Pts',(-0.0739670164814616,0.00502844388857318,
-0.385800829358656));
#46027=CARTESIAN_POINT('Ctrl Pts',(-0.0739218355690636,6.44039839332311E-5,
-0.385372744069761));
#46028=CARTESIAN_POINT('Origin',(0.,0.,-1.05327725593024));
#46029=CARTESIAN_POINT('',(-0.0738999238216348,6.62105036960088E-5,-0.473277255930238));
#46030=CARTESIAN_POINT('',(-0.0737877145894119,-2.33604236806045E-5,-0.465372744069761));
#46031=CARTESIAN_POINT('',(-0.0739,6.54188504088864E-16,-1.05327725593024));
#46032=CARTESIAN_POINT('Ctrl Pts',(-0.0738999238216348,6.6210503696003E-5,
-0.473277255930238));
#46033=CARTESIAN_POINT('Ctrl Pts',(-0.0737295153222194,-0.0187121711198471,
-0.471659091551403));
#46034=CARTESIAN_POINT('Ctrl Pts',(-0.0569357917229669,-0.0622387138293177,
-0.467931706833943));
#46035=CARTESIAN_POINT('Ctrl Pts',(0.0161067143487094,-0.0857394478691125,
-0.46209510177786));
#46036=CARTESIAN_POINT('Ctrl Pts',(0.0806498933532556,-0.0332606955748025,
-0.455767440761988));
#46037=CARTESIAN_POINT('Ctrl Pts',(0.0718639438423683,0.049459607190435,
-0.449439779746115));
#46038=CARTESIAN_POINT('Ctrl Pts',(-0.00226270426759789,0.0872098580288294,
-0.443112118730244));
#46039=CARTESIAN_POINT('Ctrl Pts',(-0.0636240999221545,0.0518389223721709,
-0.437724610791618));
#46040=CARTESIAN_POINT('Ctrl Pts',(-0.0737511824449055,0.0135983624331623,
-0.434446323191616));
#46041=CARTESIAN_POINT('Ctrl Pts',(-0.0737864256067439,-2.11896062283414E-5,
-0.433277255930238));
#46042=CARTESIAN_POINT('Ctrl Pts',(-0.0737877145894119,-2.33604236806097E-5,
-0.465372744069761));
#46043=CARTESIAN_POINT('Ctrl Pts',(-0.0738185855908912,-0.0108332925492125,
-0.464444806755477));
#46044=CARTESIAN_POINT('Ctrl Pts',(-0.0665424168125231,-0.046174863428295,
-0.461407649102569));
#46045=CARTESIAN_POINT('Ctrl Pts',(-0.0121364403459336,-0.0863908890396749,
-0.456261271111038));
#46046=CARTESIAN_POINT('Ctrl Pts',(0.0657924981506585,-0.0572889699718141,
-0.449933610095165));
#46047=CARTESIAN_POINT('Ctrl Pts',(0.0839010655140964,0.0239016756511994,
-0.443605949079294));
#46048=CARTESIAN_POINT('Ctrl Pts',(0.0257244481133483,0.0833602522944807,
-0.437278288063421));
#46049=CARTESIAN_POINT('Ctrl Pts',(-0.0526199106140298,0.0676705517485118,
-0.431200553060244));
#46050=CARTESIAN_POINT('Ctrl Pts',(-0.0738191036638569,0.0214696988294836,
-0.42723203839569));
#46051=CARTESIAN_POINT('Ctrl Pts',(-0.0739792630123745,-4.70781898877872E-5,
-0.425372744069761));
#46052=CARTESIAN_POINT('Origin',(0.,0.,-1.05327725593024));
#46053=CARTESIAN_POINT('',(-0.0739954635921359,-3.70971844019372E-5,-0.513277255930238));
#46054=CARTESIAN_POINT('',(-0.0738956892271228,6.62928153061619E-5,-0.505372744069761));
#46055=CARTESIAN_POINT('',(-0.0739,6.54188504088864E-16,-1.05327725593024));
#46056=CARTESIAN_POINT('Ctrl Pts',(-0.0739954635921359,-3.70971844019397E-5,
-0.513277255930238));
#46057=CARTESIAN_POINT('Ctrl Pts',(-0.0740088040956365,-0.00219940070345826,
-0.513090300588437));
#46058=CARTESIAN_POINT('Ctrl Pts',(-0.0729448118129387,-0.0287433874190867,
-0.510794124908012));
#46059=CARTESIAN_POINT('Ctrl Pts',(-0.0409607047580388,-0.077025319432872,
-0.506388728888963));
#46060=CARTESIAN_POINT('Ctrl Pts',(0.0422220660331108,-0.0763411835637019,
-0.500061067873091));
#46061=CARTESIAN_POINT('Ctrl Pts',(0.0870153588274602,-0.00624551808415768,
-0.49373340685722));
#46062=CARTESIAN_POINT('Ctrl Pts',(0.0526918646680198,0.0695287463271004,
-0.487405745841347));
#46063=CARTESIAN_POINT('Ctrl Pts',(-0.0295405399103716,0.082085538737435,
-0.481078084825476));
#46064=CARTESIAN_POINT('Ctrl Pts',(-0.0707533164497064,0.0358829129709433,
-0.476368588188439));
#46065=CARTESIAN_POINT('Ctrl Pts',(-0.0739516368060083,0.00576478867784635,
-0.473768311890027));
#46066=CARTESIAN_POINT('Ctrl Pts',(-0.0738999238216348,6.6210503696003E-5,
-0.473277255930238));
#46067=CARTESIAN_POINT('Ctrl Pts',(-0.0738956892271229,6.62928153061619E-5,
-0.505372744069761));
#46068=CARTESIAN_POINT('Ctrl Pts',(-0.073727254762863,-0.0185730596526899,
-0.503766795453888));
#46069=CARTESIAN_POINT('Ctrl Pts',(-0.0571405360190808,-0.0619599952174389,
-0.50005162649939));
#46070=CARTESIAN_POINT('Ctrl Pts',(0.015612887132456,-0.0858307441930048,
-0.494227237206269));
#46071=CARTESIAN_POINT('Ctrl Pts',(0.0804570900696259,-0.0337244058637655,
-0.487899576190397));
#46072=CARTESIAN_POINT('Ctrl Pts',(0.0721474666049248,0.0490451012418884,
-0.481571915174525));
#46073=CARTESIAN_POINT('Ctrl Pts',(-0.00176064224849756,0.087221436769917,
-0.475244254158653));
#46074=CARTESIAN_POINT('Ctrl Pts',(-0.0634642249304729,0.052124916693094,
-0.469844530457065));
#46075=CARTESIAN_POINT('Ctrl Pts',(-0.0737484151783087,0.0137379024521563,
-0.466554027094101));
#46076=CARTESIAN_POINT('Ctrl Pts',(-0.0737877145894119,-2.33604236806097E-5,
-0.465372744069761));
#46077=CARTESIAN_POINT('Origin',(0.,0.,-1.05327725593024));
#46078=CARTESIAN_POINT('',(-0.0737963410028765,-3.40609569993907E-5,-0.553277255930238));
#46079=CARTESIAN_POINT('',(-0.073998223225288,-3.49682871188597E-5,-0.545372744069761));
#46080=CARTESIAN_POINT('',(-0.0739,6.54188504088864E-16,-1.05327725593024));
#46081=CARTESIAN_POINT('Ctrl Pts',(-0.0737963410028765,-3.40609569993884E-5,
-0.553277255930238));
#46082=CARTESIAN_POINT('Ctrl Pts',(-0.0738385873799593,-0.0101074743734211,
-0.552412289286847));
#46083=CARTESIAN_POINT('Ctrl Pts',(-0.0672323111377545,-0.0446918455824485,
-0.549438102304832));
#46084=CARTESIAN_POINT('Ctrl Pts',(-0.0146943044302958,-0.0859927705410227,
-0.544354694984196));
#46085=CARTESIAN_POINT('Ctrl Pts',(0.0640637777501068,-0.0592158048868383,
-0.538027033968322));
#46086=CARTESIAN_POINT('Ctrl Pts',(0.0845732895170916,0.0214018192747577,
-0.531699372952452));
#46087=CARTESIAN_POINT('Ctrl Pts',(0.0281864117401041,0.0825603134758373,
-0.525371711936578));
#46088=CARTESIAN_POINT('Ctrl Pts',(-0.0514051510485292,0.0690635833670669,
-0.519231006262509));
#46089=CARTESIAN_POINT('Ctrl Pts',(-0.0738582972364053,0.0221955939339471,
-0.515199520927061));
#46090=CARTESIAN_POINT('Ctrl Pts',(-0.0739954635921359,-3.70971844019397E-5,
-0.513277255930238));
#46091=CARTESIAN_POINT('Ctrl Pts',(-0.073998223225288,-3.49682871188433E-5,
-0.545372744069761));
#46092=CARTESIAN_POINT('Ctrl Pts',(-0.0740101004843667,-0.00205578627884039,
-0.545198004490922));
#46093=CARTESIAN_POINT('Ctrl Pts',(-0.0730211466423457,-0.0284573927901487,
-0.542914044573459));
#46094=CARTESIAN_POINT('Ctrl Pts',(-0.0414034224289421,-0.076788251083785,
-0.538520864317373));
#46095=CARTESIAN_POINT('Ctrl Pts',(0.0417819068541502,-0.0765829690790775,
-0.532193203301501));
#46096=CARTESIAN_POINT('Ctrl Pts',(0.0869779631209978,-0.00674631934155149,
-0.525865542285629));
#46097=CARTESIAN_POINT('Ctrl Pts',(0.0530912336515535,0.0692242717743709,
-0.519537881269757));
#46098=CARTESIAN_POINT('Ctrl Pts',(-0.0290675236360216,0.0822542276299836,
-0.513210220253885));
#46099=CARTESIAN_POINT('Ctrl Pts',(-0.070653170669016,0.0361703843477604,
-0.508488507853886));
#46100=CARTESIAN_POINT('Ctrl Pts',(-0.0739484731718648,0.00590748781669472,
-0.505876015792512));
#46101=CARTESIAN_POINT('Ctrl Pts',(-0.0738956892271229,6.62928153061619E-5,
-0.505372744069761));
#46102=CARTESIAN_POINT('Origin',(0.,0.,-1.05327725593024));
#46103=CARTESIAN_POINT('',(-0.0738742530246062,6.53564756795162E-5,-0.593277255930239));
#46104=CARTESIAN_POINT('',(-0.073798384598233,-3.60235004422046E-5,-0.585372744069761));
#46105=CARTESIAN_POINT('',(-0.0739,6.54188504088864E-16,-1.05327725593024));
#46106=CARTESIAN_POINT('Ctrl Pts',(-0.0738742530246063,6.53564756795157E-5,
-0.593277255930239));
#46107=CARTESIAN_POINT('Ctrl Pts',(-0.0737186635600633,-0.0178563908955508,
-0.591734277985259));
#46108=CARTESIAN_POINT('Ctrl Pts',(-0.0581751526568177,-0.0605186698232157,
-0.588082079701655));
#46109=CARTESIAN_POINT('Ctrl Pts',(0.013059426400348,-0.0862561913725913,
-0.582320661079426));
#46110=CARTESIAN_POINT('Ctrl Pts',(0.0794210715600979,-0.0360967112110921,
-0.575993000063554));
#46111=CARTESIAN_POINT('Ctrl Pts',(0.0735708671919806,0.046882903799052,
-0.569665339047683));
#46112=CARTESIAN_POINT('Ctrl Pts',(0.000827981990642192,0.087235277347151,
-0.56333767803181));
#46113=CARTESIAN_POINT('Ctrl Pts',(-0.0626211499353113,0.0535971856145833,
-0.55787498365933));
#46114=CARTESIAN_POINT('Ctrl Pts',(-0.0737355696295557,0.0144565346778415,
-0.554521509625472));
#46115=CARTESIAN_POINT('Ctrl Pts',(-0.0737963410028765,-3.40609569993884E-5,
-0.553277255930238));
#46116=CARTESIAN_POINT('Ctrl Pts',(-0.073798384598233,-3.60235004422177E-5,
-0.585372744069761));
#46117=CARTESIAN_POINT('Ctrl Pts',(-0.0738425071873687,-0.00996648243522716,
-0.584519993189332));
#46118=CARTESIAN_POINT('Ctrl Pts',(-0.0673627861806156,-0.0444040547321228,
-0.58155802197028));
#46119=CARTESIAN_POINT('Ctrl Pts',(-0.0151890790080958,-0.0859067562664407,
-0.576486830412606));
#46120=CARTESIAN_POINT('Ctrl Pts',(0.0637218387120179,-0.0595836065079599,
-0.570159169396731));
#46121=CARTESIAN_POINT('Ctrl Pts',(0.0846950865125139,0.0209146172322998,
-0.563831508380862));
#46122=CARTESIAN_POINT('Ctrl Pts',(0.0286612035496907,0.0823966886738722,
-0.557503847364987));
#46123=CARTESIAN_POINT('Ctrl Pts',(-0.0511652173028116,0.0693324148388138,
-0.551350925927956));
#46124=CARTESIAN_POINT('Ctrl Pts',(-0.0738667342442603,0.0223368008907248,
-0.547307224829546));
#46125=CARTESIAN_POINT('Ctrl Pts',(-0.073998223225288,-3.49682871188433E-5,
-0.545372744069761));
#46126=CARTESIAN_POINT('Origin',(0.,0.,-1.05327725593024));
#46127=CARTESIAN_POINT('',(-0.0740100950880502,-2.31680927942999E-5,-0.633277255930238));
#46128=CARTESIAN_POINT('',(-0.0738702015529844,6.49156969421381E-5,-0.625372744069761));
#46129=CARTESIAN_POINT('',(-0.0739,6.54188504088864E-16,-1.05327725593024));
#46130=CARTESIAN_POINT('Ctrl Pts',(-0.0740100950880502,-2.31680927943018E-5,
-0.633277255930238));
#46131=CARTESIAN_POINT('Ctrl Pts',(-0.0740154327349471,-0.00131519596391571,
-0.633165487022293));
#46132=CARTESIAN_POINT('Ctrl Pts',(-0.0734008815262698,-0.0269842396990781,
-0.630944497775723));
#46133=CARTESIAN_POINT('Ctrl Pts',(-0.0436634932506345,-0.0755260122418957,
-0.62661428819053));
#46134=CARTESIAN_POINT('Ctrl Pts',(0.0394913060792223,-0.0777889189548767,
-0.620286627174658));
#46135=CARTESIAN_POINT('Ctrl Pts',(0.0867395103929965,-0.00932397473154213,
-0.613958966158786));
#46136=CARTESIAN_POINT('Ctrl Pts',(0.0551217368298506,0.0676185869186267,
-0.607631305142914));
#46137=CARTESIAN_POINT('Ctrl Pts',(-0.0266142545750163,0.0830804466852906,
-0.601303644127043));
#46138=CARTESIAN_POINT('Ctrl Pts',(-0.0701214900469694,0.0376528645843343,
-0.59651896105615));
#46139=CARTESIAN_POINT('Ctrl Pts',(-0.0739313512813346,0.00664228336098339,
-0.593843498323883));
#46140=CARTESIAN_POINT('Ctrl Pts',(-0.0738742530246063,6.53564756795157E-5,
-0.593277255930239));
#46141=CARTESIAN_POINT('Ctrl Pts',(-0.0738702015529844,6.49156969421468E-5,
-0.625372744069761));
#46142=CARTESIAN_POINT('Ctrl Pts',(-0.0737175639680371,-0.0177174244228303,
-0.623841981887743));
#46143=CARTESIAN_POINT('Ctrl Pts',(-0.0583718441882899,-0.0602382191459097,
-0.620201999367102));
#46144=CARTESIAN_POINT('Ctrl Pts',(0.012562675089579,-0.0863299373793905,
-0.614452796507836));
#46145=CARTESIAN_POINT('Ctrl Pts',(0.0792119631042182,-0.0365533007334742,
-0.608125135491964));
#46146=CARTESIAN_POINT('Ctrl Pts',(0.0738395288211365,0.0464586146673402,
-0.601797474476092));
#46147=CARTESIAN_POINT('Ctrl Pts',(0.00133013907144687,0.0872290640978479,
-0.59546981346022));
#46148=CARTESIAN_POINT('Ctrl Pts',(-0.062453895076773,0.053882371915127,
-0.589994903324777));
#46149=CARTESIAN_POINT('Ctrl Pts',(-0.0737333730140319,0.0145958210907477,
-0.586629213527957));
#46150=CARTESIAN_POINT('Ctrl Pts',(-0.073798384598233,-3.60235004422177E-5,
-0.585372744069761));
#46151=CARTESIAN_POINT('Origin',(0.,0.,-1.05327725593024));
#46152=CARTESIAN_POINT('',(-0.0738107316200561,-4.54136549985855E-5,-0.673277255930238));
#46153=CARTESIAN_POINT('',(-0.0740118889580303,-2.07425011237994E-5,-0.665372744069761));
#46154=CARTESIAN_POINT('',(-0.0739,6.54188504088864E-16,-1.05327725593024));
#46155=CARTESIAN_POINT('Ctrl Pts',(-0.0738107316200561,-4.54136549985842E-5,
-0.673277255930238));
#46156=CARTESIAN_POINT('Ctrl Pts',(-0.073862779055793,-0.00923870797648464,
-0.672487475720703));
#46157=CARTESIAN_POINT('Ctrl Pts',(-0.0680183112542861,-0.0429202091247773,
-0.669588475172544));
#46158=CARTESIAN_POINT('Ctrl Pts',(-0.0177312350715336,-0.0854182794889314,
-0.664580254285763));
#46159=CARTESIAN_POINT('Ctrl Pts',(0.0619259482971724,-0.0614479950487169,
-0.65825259326989));
#46160=CARTESIAN_POINT('Ctrl Pts',(0.0852783353131607,0.0183925173434011,
-0.651924932254018));
#46161=CARTESIAN_POINT('Ctrl Pts',(0.0310932855172931,0.0815100408768839,
-0.645597271238146));
#46162=CARTESIAN_POINT('Ctrl Pts',(-0.049906181360674,0.0707105530622803,
-0.63938137913022));
#46163=CARTESIAN_POINT('Ctrl Pts',(-0.0739147046022107,0.0230670004262463,
-0.635274707360917));
#46164=CARTESIAN_POINT('Ctrl Pts',(-0.0740100950880502,-2.31680927943018E-5,
-0.633277255930238));
#46165=CARTESIAN_POINT('Ctrl Pts',(-0.0740118889580303,-2.07425011238048E-5,
-0.665372744069761));
#46166=CARTESIAN_POINT('Ctrl Pts',(-0.0740161983599743,-0.00117148387544626,
-0.665273190924778));
#46167=CARTESIAN_POINT('Ctrl Pts',(-0.0734718979508283,-0.0266986788458054,
-0.663064417441171));
#46168=CARTESIAN_POINT('Ctrl Pts',(-0.044097535312672,-0.0752734101305599,
-0.65874642361894));
#46169=CARTESIAN_POINT('Ctrl Pts',(0.0390428582906939,-0.0780149608077107,
-0.652418762603067));
#46170=CARTESIAN_POINT('Ctrl Pts',(0.0866843980931254,-0.00982313700242362,
-0.646091101587197));
#46171=CARTESIAN_POINT('Ctrl Pts',(0.0555100696561328,0.0673001564642097,
-0.639763440571324));
#46172=CARTESIAN_POINT('Ctrl Pts',(-0.0261355596403159,0.0832322738823306,
-0.633435779555452));
#46173=CARTESIAN_POINT('Ctrl Pts',(-0.0700153218516501,0.0379405554487119,
-0.628638880721598));
#46174=CARTESIAN_POINT('Ctrl Pts',(-0.0739278816139727,0.00678466603221187,
-0.625951202226367));
#46175=CARTESIAN_POINT('Ctrl Pts',(-0.0738702015529844,6.49156969421468E-5,
-0.625372744069761));
#46176=CARTESIAN_POINT('Origin',(0.,0.,-1.05327725593024));
#46177=CARTESIAN_POINT('',(-0.0738501444728052,6.13634501804807E-5,-0.713277255930238));
#46178=CARTESIAN_POINT('',(-0.0738134589801114,-4.70777110323853E-5,-0.705372744069761));
#46179=CARTESIAN_POINT('',(-0.0739,6.54188504088864E-16,-1.05327725593024));
#46180=CARTESIAN_POINT('Ctrl Pts',(-0.0738501444728051,6.13634501804728E-5,
-0.713277255930238));
#46181=CARTESIAN_POINT('Ctrl Pts',(-0.0737146405834979,-0.0170012191686346,
-0.711809464419114));
#46182=CARTESIAN_POINT('Ctrl Pts',(-0.0593652872484897,-0.0587885221188445,
-0.708232452569367));
#46183=CARTESIAN_POINT('Ctrl Pts',(0.00999574615152227,-0.0866646653884117,
-0.702546220380994));
#46184=CARTESIAN_POINT('Ctrl Pts',(0.0780925597784293,-0.0388874179557339,
-0.696218559365122));
#46185=CARTESIAN_POINT('Ctrl Pts',(0.0751854437781816,0.0442473525975172,
-0.68989089834925));
#46186=CARTESIAN_POINT('Ctrl Pts',(0.00391762895901338,0.0871511982209692,
-0.683563237333377));
#46187=CARTESIAN_POINT('Ctrl Pts',(-0.0615723981039191,0.0553500429250213,
-0.678025356527042));
#46188=CARTESIAN_POINT('Ctrl Pts',(-0.0737237789786778,0.0153132915896411,
-0.674596696059328));
#46189=CARTESIAN_POINT('Ctrl Pts',(-0.0738107316200561,-4.54136549985842E-5,
-0.673277255930238));
#46190=CARTESIAN_POINT('Ctrl Pts',(-0.0738134589801114,-4.70777110323862E-5,
-0.705372744069761));
#46191=CARTESIAN_POINT('Ctrl Pts',(-0.0738667027928598,-0.00909733596711184,
-0.704595179623188));
#46192=CARTESIAN_POINT('Ctrl Pts',(-0.068142195106051,-0.0426323122661008,
-0.701708394837992));
#46193=CARTESIAN_POINT('Ctrl Pts',(-0.0182226522121619,-0.0853147926193951,
-0.696712389714172));
#46194=CARTESIAN_POINT('Ctrl Pts',(0.0615711950922978,-0.0618034532064518,
-0.690384728698299));
#46195=CARTESIAN_POINT('Ctrl Pts',(0.0853827975350567,0.0179013066121811,
-0.684057067682429));
#46196=CARTESIAN_POINT('Ctrl Pts',(0.0315619832053435,0.0813297000454412,
-0.677729406666555));
#46197=CARTESIAN_POINT('Ctrl Pts',(-0.0496576109998276,0.0709763587008032,
-0.671501298795667));
#46198=CARTESIAN_POINT('Ctrl Pts',(-0.0739248955866761,0.0232091332474935,
-0.667382411263402));
#46199=CARTESIAN_POINT('Ctrl Pts',(-0.0740118889580303,-2.07425011238048E-5,
-0.665372744069761));
#46200=CARTESIAN_POINT('Origin',(0.,0.,-1.05327725593024));
#46201=CARTESIAN_POINT('',(-0.0740181195037208,-7.75676069538861E-6,-0.753277255930239));
#46202=CARTESIAN_POINT('',(-0.0738464406987289,6.04347504972284E-5,-0.745372744069761));
#46203=CARTESIAN_POINT('',(-0.0739,6.54188504088864E-16,-1.05327725593024));
#46204=CARTESIAN_POINT('Ctrl Pts',(-0.0740181195037208,-7.75676069538801E-6,
-0.753277255930239));
#46205=CARTESIAN_POINT('Ctrl Pts',(-0.0740187541717008,-0.000430520586765759,
-0.753240673456149));
#46206=CARTESIAN_POINT('Ctrl Pts',(-0.07382453043895,-0.0252278019321763,
-0.751094870643435));
#46207=CARTESIAN_POINT('Ctrl Pts',(-0.0463114749636612,-0.0739319041732507,
-0.746839847492097));
#46208=CARTESIAN_POINT('Ctrl Pts',(0.0367109763098753,-0.0791390130490189,
-0.740512186476226));
#46209=CARTESIAN_POINT('Ctrl Pts',(0.0863547858049027,-0.0123907278484321,
-0.734184525460353));
#46210=CARTESIAN_POINT('Ctrl Pts',(0.0574824197298575,0.0656235520983735,
-0.727856864444481));
#46211=CARTESIAN_POINT('Ctrl Pts',(-0.0236545628063002,0.0839710713665869,
-0.72152920342861));
#46212=CARTESIAN_POINT('Ctrl Pts',(-0.069452220378256,0.0394239899284276,
-0.716669333923862));
#46213=CARTESIAN_POINT('Ctrl Pts',(-0.073909360035902,0.00751775782251194,
-0.713918684757738));
#46214=CARTESIAN_POINT('Ctrl Pts',(-0.0738501444728051,6.13634501804728E-5,
-0.713277255930238));
#46215=CARTESIAN_POINT('Ctrl Pts',(-0.0738464406987288,6.04347504972241E-5,
-0.745372744069761));
#46216=CARTESIAN_POINT('Ctrl Pts',(-0.0737145788249443,-0.0168622901615721,
-0.743917168321599));
#46217=CARTESIAN_POINT('Ctrl Pts',(-0.0595540578546233,-0.0585065533281464,
-0.740352372234814));
#46218=CARTESIAN_POINT('Ctrl Pts',(0.00949669427259201,-0.0867207685115116,
-0.734678355809403));
#46219=CARTESIAN_POINT('Ctrl Pts',(0.0778674086249794,-0.0393363135965772,
-0.728350694793532));
#46220=CARTESIAN_POINT('Ctrl Pts',(0.0754389070476233,0.0438138128538845,
-0.722023033777659));
#46221=CARTESIAN_POINT('Ctrl Pts',(0.00441925078978631,0.0871272007801963,
-0.715695372761787));
#46222=CARTESIAN_POINT('Ctrl Pts',(-0.0613976166205516,0.0556342510285772,
-0.710145276192489));
#46223=CARTESIAN_POINT('Ctrl Pts',(-0.0737222736934459,0.0154523831817844,
-0.706704399961813));
#46224=CARTESIAN_POINT('Ctrl Pts',(-0.0738134589801114,-4.70777110323862E-5,
-0.705372744069761));
#46225=CARTESIAN_POINT('Origin',(0.,0.,-1.05327725593024));
#46226=CARTESIAN_POINT('',(-0.0738290934588786,-5.47168357983042E-5,-0.793277255930239));
#46227=CARTESIAN_POINT('',(-0.0740186890690066,-5.17471746349502E-6,-0.785372744069761));
#46228=CARTESIAN_POINT('',(-0.0739,6.54188504088864E-16,-1.05327725593024));
#46229=CARTESIAN_POINT('Ctrl Pts',(-0.0738290934588786,-5.47168357983097E-5,
-0.793277255930239));
#46230=CARTESIAN_POINT('Ctrl Pts',(-0.0738867553000471,-0.0083676131166434,
-0.79256266215456));
#46231=CARTESIAN_POINT('Ctrl Pts',(-0.0687641349176097,-0.0411481838791359,
-0.789738848040257));
#46232=CARTESIAN_POINT('Ctrl Pts',(-0.0207459093066268,-0.0847365707051847,
-0.784805813587329));
#46233=CARTESIAN_POINT('Ctrl Pts',(0.0597103888730514,-0.0636030551758837,
-0.778478152571458));
#46234=CARTESIAN_POINT('Ctrl Pts',(0.0858763390381331,0.0153601289709793,
-0.772150491555585));
#46235=CARTESIAN_POINT('Ctrl Pts',(0.0339611307424576,0.0803574561980857,
-0.765822830539714));
#46236=CARTESIAN_POINT('Ctrl Pts',(-0.0483538236456822,0.0723381788220632,
-0.75953175199793));
#46237=CARTESIAN_POINT('Ctrl Pts',(-0.0739821613866291,0.0239445957105796,
-0.755349893794773));
#46238=CARTESIAN_POINT('Ctrl Pts',(-0.0740181195037208,-7.75676069538801E-6,
-0.753277255930239));
#46239=CARTESIAN_POINT('Ctrl Pts',(-0.0740186890690066,-5.17471746348515E-6,
-0.785372744069761));
#46240=CARTESIAN_POINT('Ctrl Pts',(-0.0740189752447098,-0.000286761730465124,
-0.785348377358633));
#46241=CARTESIAN_POINT('Ctrl Pts',(-0.0738903489069693,-0.0249426889494393,
-0.783214790308882));
#46242=CARTESIAN_POINT('Ctrl Pts',(-0.0467362966021223,-0.0736640853684918,
-0.778971982920508));
#46243=CARTESIAN_POINT('Ctrl Pts',(0.0362548028063699,-0.0793490275094065,
-0.772644321904634));
#46244=CARTESIAN_POINT('Ctrl Pts',(0.0862820260894591,-0.0128876245803302,
-0.766316660888764));
#46245=CARTESIAN_POINT('Ctrl Pts',(0.0578592289600791,0.0652915654389009,
-0.759988999872889));
#46246=CARTESIAN_POINT('Ctrl Pts',(-0.0231707900729891,0.0841058462933171,
-0.753661338857021));
#46247=CARTESIAN_POINT('Ctrl Pts',(-0.0693398833707779,0.0397118294936949,
-0.748789253589309));
#46248=CARTESIAN_POINT('Ctrl Pts',(-0.0739056549310326,0.00765979713931138,
-0.746026388660223));
#46249=CARTESIAN_POINT('Ctrl Pts',(-0.0738464406987288,6.04347504972241E-5,
-0.745372744069761));
#46250=CARTESIAN_POINT('Origin',(0.,0.,-1.05327725593024));
#46251=CARTESIAN_POINT('',(-0.0738285525876018,5.44975647950647E-5,-0.833277255930239));
#46252=CARTESIAN_POINT('',(-0.0738324075238535,-5.60022767805285E-5,-0.825372744069761));
#46253=CARTESIAN_POINT('',(-0.0739,6.54188504088864E-16,-1.05327725593024));
#46254=CARTESIAN_POINT('Ctrl Pts',(-0.0738285525876017,5.44975647950637E-5,
-0.833277255930239));
#46255=CARTESIAN_POINT('Ctrl Pts',(-0.0737166860120861,-0.0161460284618373,
-0.83188465085297));
#46256=CARTESIAN_POINT('Ctrl Pts',(-0.0605070205977865,-0.0570495580085797,
-0.828382825437078));
#46257=CARTESIAN_POINT('Ctrl Pts',(0.00691951974818428,-0.0869643572919913,
-0.82277177968256));
#46258=CARTESIAN_POINT('Ctrl Pts',(0.0766660252567158,-0.0416293128401549,
-0.81644411866669));
#46259=CARTESIAN_POINT('Ctrl Pts',(0.0767056471347569,0.0415562617250705,
-0.810116457650816));
#46260=CARTESIAN_POINT('Ctrl Pts',(0.00700235840066891,0.0869577262010798,
-0.803788796634946));
#46261=CARTESIAN_POINT('Ctrl Pts',(-0.0604769485808272,0.0570964171803072,
-0.798175729394752));
#46262=CARTESIAN_POINT('Ctrl Pts',(-0.073716558564091,0.0161690264472331,
-0.794671882493184));
#46263=CARTESIAN_POINT('Ctrl Pts',(-0.0738290934588786,-5.47168357983097E-5,
-0.793277255930239));
#46264=CARTESIAN_POINT('Ctrl Pts',(-0.0738324075238535,-5.60022767805354E-5,
-0.825372744069761));
#46265=CARTESIAN_POINT('Ctrl Pts',(-0.0738905913104309,-0.00822586691819469,
-0.824670366057044));
#46266=CARTESIAN_POINT('Ctrl Pts',(-0.0688815793035972,-0.0408602812647409,
-0.821858767705704));
#46267=CARTESIAN_POINT('Ctrl Pts',(-0.0212333521088858,-0.0846157411642612,
-0.816937949015739));
#46268=CARTESIAN_POINT('Ctrl Pts',(0.0593432667534829,-0.0639457236824982,
-0.810610287999866));
#46269=CARTESIAN_POINT('Ctrl Pts',(0.0859633353842028,0.014865526115561,
-0.804282626983996));
#46270=CARTESIAN_POINT('Ctrl Pts',(0.0344231459854351,0.0801606257062834,
-0.797954965968122));
#46271=CARTESIAN_POINT('Ctrl Pts',(-0.0480965289443807,0.072600677106953,
-0.79165167166338));
#46272=CARTESIAN_POINT('Ctrl Pts',(-0.0739942034316283,0.0240878472108019,
-0.787457597697257));
#46273=CARTESIAN_POINT('Ctrl Pts',(-0.0740186890690066,-5.17471746348515E-6,
-0.785372744069761));
#46274=CARTESIAN_POINT('Origin',(0.,0.,-1.05327725593024));
#46275=CARTESIAN_POINT('',(-0.0740179768487384,8.17838895347943E-6,-0.873277255930239));
#46276=CARTESIAN_POINT('',(-0.0738253349991919,5.31336276900878E-5,-0.865372744069761));
#46277=CARTESIAN_POINT('',(-0.0739,6.54188504088864E-16,-1.05327725593024));
#46278=CARTESIAN_POINT('Ctrl Pts',(-0.0740179768487384,8.17838895347957E-6,
-0.873277255930238));
#46279=CARTESIAN_POINT('Ctrl Pts',(-0.0739801514683282,-0.0239209166759214,
-0.871206639551381));
#46280=CARTESIAN_POINT('Ctrl Pts',(-0.0483963153428398,-0.0722946776724089,
-0.8670268028339));
#46281=CARTESIAN_POINT('Ctrl Pts',(0.0338845940526951,-0.0803897756396443,
-0.860737745777792));
#46282=CARTESIAN_POINT('Ctrl Pts',(0.0858616535090988,-0.0154419256785799,
-0.854410084761921));
#46283=CARTESIAN_POINT('Ctrl Pts',(0.0597709578444863,0.0635461448157645,
-0.848082423746049));
#46284=CARTESIAN_POINT('Ctrl Pts',(-0.0206651836539401,0.0847562955128429,
-0.841754762730177));
#46285=CARTESIAN_POINT('Ctrl Pts',(-0.0687445992449014,0.0411958268432829,
-0.836819706791573));
#46286=CARTESIAN_POINT('Ctrl Pts',(-0.0738861175760961,0.00839106360363198,
-0.833993871191594));
#46287=CARTESIAN_POINT('Ctrl Pts',(-0.0738285525876017,5.44975647950637E-5,
-0.833277255930239));
#46288=CARTESIAN_POINT('Ctrl Pts',(-0.0738253349991919,5.31336276900912E-5,
-0.865372744069761));
#46289=CARTESIAN_POINT('Ctrl Pts',(-0.0737175361431159,-0.0160070434472833,
-0.863992354755455));
#46290=CARTESIAN_POINT('Ctrl Pts',(-0.0606880120450771,-0.0567662717423334,
-0.860502745102525));
#46291=CARTESIAN_POINT('Ctrl Pts',(0.00641879698876544,-0.0870027483201755,
-0.85490391511097));
#46292=CARTESIAN_POINT('Ctrl Pts',(0.076425112291304,-0.0420699505040234,
-0.8485762540951));
#46293=CARTESIAN_POINT('Ctrl Pts',(0.0769435948053001,0.0411140152158757,
-0.842248593079225));
#46294=CARTESIAN_POINT('Ctrl Pts',(0.0075028148617241,0.0869159748679489,
-0.835920932063356));
#46295=CARTESIAN_POINT('Ctrl Pts',(-0.0602944965619087,0.0573794653213463,
-0.830295649060199));
#46296=CARTESIAN_POINT('Ctrl Pts',(-0.0737158671251557,0.0163079942697733,
-0.826779586395668));
#46297=CARTESIAN_POINT('Ctrl Pts',(-0.0738324075238535,-5.60022767805354E-5,
-0.825372744069761));
#46298=CARTESIAN_POINT('Origin',(0.,0.,-1.05327725593024));
#46299=CARTESIAN_POINT('',(-0.0738511720378038,-6.144379322435E-5,-0.913277255930239));
#46300=CARTESIAN_POINT('',(-0.0740169999568149,1.06868542633972E-5,-0.905372744069761));
#46301=CARTESIAN_POINT('',(-0.0739,6.54188504088864E-16,-1.05327725593024));
#46302=CARTESIAN_POINT('Ctrl Pts',(-0.0738511720378038,-6.14437932243417E-5,
-0.913277255930239));
#46303=CARTESIAN_POINT('Ctrl Pts',(-0.0739097105108123,-0.00749428940729366,
-0.912637848588415));
#46304=CARTESIAN_POINT('Ctrl Pts',(-0.0694677457128137,-0.0393768397509905,
-0.909889220907968));
#46305=CARTESIAN_POINT('Ctrl Pts',(-0.0237369667204929,-0.0839481073924034,
-0.905031372888896));
#46306=CARTESIAN_POINT('Ctrl Pts',(0.0574211581950477,-0.0656784871371439,
-0.898703711873025));
#46307=CARTESIAN_POINT('Ctrl Pts',(0.0863658764533893,0.0123085695241889,
-0.892376050857153));
#46308=CARTESIAN_POINT('Ctrl Pts',(0.0367867028056418,0.0791039486621042,
-0.88604838984128));
#46309=CARTESIAN_POINT('Ctrl Pts',(-0.0462412134555447,0.0739760173765286,
-0.879720728825409));
#46310=CARTESIAN_POINT('Ctrl Pts',(-0.0738135527330108,0.0252749890993244,
-0.875463684188394));
#46311=CARTESIAN_POINT('Ctrl Pts',(-0.074018682053951,0.000454305364743116,
-0.873315859890004));
#46312=CARTESIAN_POINT('Ctrl Pts',(-0.0740179768487384,8.17838895347957E-6,
-0.873277255930238));
#46313=CARTESIAN_POINT('Ctrl Pts',(-0.0740169999568149,1.06868542633994E-5,
-0.905372744069761));
#46314=CARTESIAN_POINT('Ctrl Pts',(-0.0739682091453213,-0.0237779860315713,
-0.903314343453865));
#46315=CARTESIAN_POINT('Ctrl Pts',(-0.0486522352802609,-0.0720314229341465,
-0.899146722499347));
#46316=CARTESIAN_POINT('Ctrl Pts',(0.0334214198190593,-0.0805835554203335,
-0.892869881206202));
#46317=CARTESIAN_POINT('Ctrl Pts',(0.0857712573590327,-0.0159359034660176,
-0.88654222019033));
#46318=CARTESIAN_POINT('Ctrl Pts',(0.0601358128673054,0.0632010030064432,
-0.880214559174458));
#46319=CARTESIAN_POINT('Ctrl Pts',(-0.0201769626930229,0.084873857253752,
-0.873886898158586));
#46320=CARTESIAN_POINT('Ctrl Pts',(-0.0686259403155307,0.0414837324433979,
-0.868939626457021));
#46321=CARTESIAN_POINT('Ctrl Pts',(-0.0738822516602237,0.00853273803129299,
-0.866101575094079));
#46322=CARTESIAN_POINT('Ctrl Pts',(-0.0738253349991919,5.31336276900912E-5,
-0.865372744069761));
#46323=CARTESIAN_POINT('Origin',(0.,0.,-1.05327725593024));
#46324=CARTESIAN_POINT('',(-0.0739,6.54188504088864E-16,-0.949325));
#46325=CARTESIAN_POINT('',(-0.0738572813634733,-6.14771210490569E-5,-0.945372744069761));
#46326=CARTESIAN_POINT('',(-0.0739,6.54188504088864E-16,-1.05327725593024));
#46327=CARTESIAN_POINT('',(-0.0601104350279399,-0.0429877377952343,-0.949325));
#46328=CARTESIAN_POINT('Origin',(0.,0.,-0.949325));
#46329=CARTESIAN_POINT('Ctrl Pts',(-0.0601104350279403,-0.0429877377952337,
-0.949325));
#46330=CARTESIAN_POINT('Ctrl Pts',(-0.0458679287777906,-0.0629032599997909,
-0.947215779661376));
#46331=CARTESIAN_POINT('Ctrl Pts',(0.00371043826886423,-0.0871365202941097,
-0.942997338984126));
#46332=CARTESIAN_POINT('Ctrl Pts',(0.0752041131369929,-0.0443285976848148,
-0.936669677968258));
#46333=CARTESIAN_POINT('Ctrl Pts',(0.0780980364899326,0.0388180903923549,
-0.930342016952383));
#46334=CARTESIAN_POINT('Ctrl Pts',(0.0100948570851079,0.0866524255516566,
-0.924014355936512));
#46335=CARTESIAN_POINT('Ctrl Pts',(-0.0593400932047787,0.0588361590846621,
-0.918326102262464));
#46336=CARTESIAN_POINT('Ctrl Pts',(-0.0737166089778999,0.0170245237460521,
-0.914747068927039));
#46337=CARTESIAN_POINT('Ctrl Pts',(-0.0738511720378038,-6.14437932243417E-5,
-0.913277255930239));
#46338=CARTESIAN_POINT('Ctrl Pts',(-0.0738572813634733,-6.14771210490526E-5,
-0.945372744069761));
#46339=CARTESIAN_POINT('Ctrl Pts',(-0.0739120474282235,-0.0073527222198075,
-0.9447455524909));
#46340=CARTESIAN_POINT('Ctrl Pts',(-0.0695624069951655,-0.0390950973922719,
-0.942009140573414));
#46341=CARTESIAN_POINT('Ctrl Pts',(-0.0242332971309306,-0.0838051103417385,
-0.937163508317307));
#46342=CARTESIAN_POINT('Ctrl Pts',(0.0570492242990965,-0.06601055836573,
-0.930835847301434));
#46343=CARTESIAN_POINT('Ctrl Pts',(0.0864315571449822,0.0118125778999351,
-0.924508186285562));
#46344=CARTESIAN_POINT('Ctrl Pts',(0.0372434277651266,0.0788901466696481,
-0.91818052526969));
#46345=CARTESIAN_POINT('Ctrl Pts',(-0.0458156426390635,0.0742413616113632,
-0.911852864253818));
#46346=CARTESIAN_POINT('Ctrl Pts',(-0.0737467241149971,0.0255601749070422,
-0.907583603853842));
#46347=CARTESIAN_POINT('Ctrl Pts',(-0.0740182045500766,0.000598003895852526,
-0.905423563792489));
#46348=CARTESIAN_POINT('Ctrl Pts',(-0.0740169999568149,1.06868542633994E-5,
-0.905372744069761));
#46349=CARTESIAN_POINT('Origin',(2.39206768658147E-17,-5.43753587379397E-18,
-0.013325));
#46350=CARTESIAN_POINT('',(-0.0452560140322625,0.0854280329804665,-0.013325));
#46351=CARTESIAN_POINT('Ctrl Pts',(0.0740154662741574,-0.000526981588892629,
-0.013325));
#46352=CARTESIAN_POINT('Ctrl Pts',(0.0743274162787444,0.00138720916901943,
-0.0133249999999999));
#46353=CARTESIAN_POINT('Ctrl Pts',(0.0745584091685309,0.00331039779856178,
-0.0133250000000001));
#46354=CARTESIAN_POINT('Ctrl Pts',(0.0747064997395148,0.00523801887942489,
-0.0133250000000002));
#46355=CARTESIAN_POINT('Ctrl Pts',(0.0750471992924708,0.0096727349869759,
-0.0133250000000002));
#46356=CARTESIAN_POINT('Ctrl Pts',(0.0749501667319329,0.0141305889760572,
-0.0133250000000002));
#46357=CARTESIAN_POINT('Ctrl Pts',(0.0744523966822522,0.0185654001727163,
-0.0133250000000004));
#46358=CARTESIAN_POINT('Ctrl Pts',(0.0741100333998832,0.0216156369616686,
-0.0133250000000006));
#46359=CARTESIAN_POINT('Ctrl Pts',(0.0735783232628857,0.0246476071870298,
-0.0133249999999998));
#46360=CARTESIAN_POINT('Ctrl Pts',(0.0728709746069023,0.0276395260463149,
-0.0133249999999999));
#46361=CARTESIAN_POINT('Ctrl Pts',(0.0719811966983897,0.0314030778429219,
-0.0133250000000001));
#46362=CARTESIAN_POINT('Ctrl Pts',(0.0708133325873436,0.0351067594379044,
-0.0133250000000001));
#46363=CARTESIAN_POINT('Ctrl Pts',(0.069386882975893,0.0387224916969436,
-0.0133250000000001));
#46364=CARTESIAN_POINT('Ctrl Pts',(0.0684028077464189,0.0412169033634814,
-0.0133250000000002));
#46365=CARTESIAN_POINT('Ctrl Pts',(0.0672972189702868,0.0436644443409473,
-0.0133250000000002));
#46366=CARTESIAN_POINT('Ctrl Pts',(0.0660807270923872,0.0460490974145337,
-0.0133250000000002));
#46367=CARTESIAN_POINT('Ctrl Pts',(0.0630085800683589,0.0520713364252927,
-0.0133250000000003));
#46368=CARTESIAN_POINT('Ctrl Pts',(0.0592273612473775,0.0577071685296467,
-0.0133250000000001));
#46369=CARTESIAN_POINT('Ctrl Pts',(0.054825249512648,0.0628151653134337,
-0.0133250000000001));
#46370=CARTESIAN_POINT('Ctrl Pts',(0.0527049155254095,0.0652754979537713,
-0.0133250000000001));
#46371=CARTESIAN_POINT('Ctrl Pts',(0.0504362001885655,0.0676156486678103,
-0.0133250000000002));
#46372=CARTESIAN_POINT('Ctrl Pts',(0.0480475571159952,0.0697999749756303,
-0.0133250000000002));
#46373=CARTESIAN_POINT('Ctrl Pts',(0.0460015562349771,0.071670967591292,
-0.0133250000000001));
#46374=CARTESIAN_POINT('Ctrl Pts',(0.0438653825571326,0.0734306648289896,
-0.0133250000000002));
#46375=CARTESIAN_POINT('Ctrl Pts',(0.0416450739245558,0.0750698920282756,
-0.0133250000000002));
#46376=CARTESIAN_POINT('Ctrl Pts',(0.0374507997065208,0.0781664743135446,
-0.0133250000000002));
#46377=CARTESIAN_POINT('Ctrl Pts',(0.0329571089215552,0.0808340896140399,
-0.0133250000000002));
#46378=CARTESIAN_POINT('Ctrl Pts',(0.0282314170935856,0.0830783479911864,
-0.0133250000000001));
#46379=CARTESIAN_POINT('Ctrl Pts',(0.0254273460850914,0.0844100175286878,
-0.0133250000000001));
#46380=CARTESIAN_POINT('Ctrl Pts',(0.0225383922404567,0.0855928024630465,
-0.0133250000000001));
#46381=CARTESIAN_POINT('Ctrl Pts',(0.0196009575542751,0.0866189242160582,
-0.0133250000000001));
#46382=CARTESIAN_POINT('Ctrl Pts',(0.0144103595069212,0.0884321340867615,
-0.0133250000000002));
#46383=CARTESIAN_POINT('Ctrl Pts',(0.00905575240102509,0.0897644221558753,
-0.0133250000000002));
#46384=CARTESIAN_POINT('Ctrl Pts',(0.00361197019240061,0.0906224587811647,
-0.0133250000000002));
#46385=CARTESIAN_POINT('Ctrl Pts',(-0.000441340334494331,0.0912613324084449,
-0.0133250000000001));
#46386=CARTESIAN_POINT('Ctrl Pts',(-0.00454446622826156,0.0916370240537867,
-0.0133250000000001));
#46387=CARTESIAN_POINT('Ctrl Pts',(-0.00866962335769465,0.0917466885842836,
-0.0133250000000001));
#46388=CARTESIAN_POINT('Ctrl Pts',(-0.0114737278358596,0.0918212338176926,
-0.0133250000000001));
#46389=CARTESIAN_POINT('Ctrl Pts',(-0.014279644527722,0.0917723286717455,
-0.013325));
#46390=CARTESIAN_POINT('Ctrl Pts',(-0.0170720954237708,0.091600917740833,
-0.013325));
#46391=CARTESIAN_POINT('Ctrl Pts',(-0.0245642157420065,0.0911410237745421,
-0.013325));
#46392=CARTESIAN_POINT('Ctrl Pts',(-0.0319725491600437,0.0898033415291956,
-0.0133249999999999));
#46393=CARTESIAN_POINT('Ctrl Pts',(-0.039131992857135,0.0875766958826527,
-0.0133250000000001));
#46394=CARTESIAN_POINT('Ctrl Pts',(-0.041195285566919,0.0869349949455183,
-0.0133250000000001));
#46395=CARTESIAN_POINT('Ctrl Pts',(-0.0432379503387495,0.0862191367302635,
-0.013325));
#46396=CARTESIAN_POINT('Ctrl Pts',(-0.0452560140322624,0.0854280329804665,
-0.013325));
#46397=CARTESIAN_POINT('',(-0.096675,-1.1839272930757E-17,-0.013325));
#46398=CARTESIAN_POINT('Origin',(0.,0.,-0.013325));
#46399=CARTESIAN_POINT('',(-0.0953105349179715,0.0166374124980891,-0.0133249999999999));
#46400=CARTESIAN_POINT('Origin',(0.,0.,-0.013325));
#46401=CARTESIAN_POINT('Ctrl Pts',(-0.0953893049619548,0.0166325119362263,
-0.0133249999999998));
#46402=CARTESIAN_POINT('Ctrl Pts',(-0.0955491516473957,0.0141405248991806,
-0.0133249999999998));
#46403=CARTESIAN_POINT('Ctrl Pts',(-0.0956055203501725,0.0116461842161637,
-0.0133249999999999));
#46404=CARTESIAN_POINT('Ctrl Pts',(-0.0955546587076807,0.00915419853455082,
-0.0133249999999998));
#46405=CARTESIAN_POINT('Ctrl Pts',(-0.0954492895571674,0.00399159659135037,
-0.0133249999999998));
#46406=CARTESIAN_POINT('Ctrl Pts',(-0.0948843160835839,-0.00116127963385684,
-0.013325));
#46407=CARTESIAN_POINT('Ctrl Pts',(-0.0938852470810883,-0.00625275390846729,
-0.0133250000000003));
#46408=CARTESIAN_POINT('Ctrl Pts',(-0.093293720913368,-0.00926730070972282,
-0.0133250000000004));
#46409=CARTESIAN_POINT('Ctrl Pts',(-0.092549661853774,-0.0122589890978512,
-0.0133250000000002));
#46410=CARTESIAN_POINT('Ctrl Pts',(-0.0916618445562462,-0.0152047979384899,
-0.0133250000000002));
#46411=CARTESIAN_POINT('Ctrl Pts',(-0.0899959881019879,-0.020732167909602,
-0.0133250000000002));
#46412=CARTESIAN_POINT('Ctrl Pts',(-0.0878227127820439,-0.0261107468918155,
-0.0133250000000002));
#46413=CARTESIAN_POINT('Ctrl Pts',(-0.085173648547477,-0.0312627955199005,
-0.0133250000000003));
#46414=CARTESIAN_POINT('Ctrl Pts',(-0.0838153418310689,-0.0339045065677011,
-0.0133250000000004));
#46415=CARTESIAN_POINT('Ctrl Pts',(-0.0823348229585785,-0.0364799319891756,
-0.0133250000000005));
#46416=CARTESIAN_POINT('Ctrl Pts',(-0.0807412291085146,-0.0389724889468894,
-0.0133250000000004));
#46417=CARTESIAN_POINT('Ctrl Pts',(-0.0769763666135518,-0.0448611501049876,
-0.0133250000000003));
#46418=CARTESIAN_POINT('Ctrl Pts',(-0.072575731259438,-0.0503026910650738,
-0.013325));
#46419=CARTESIAN_POINT('Ctrl Pts',(-0.067591694538167,-0.0551448578224046,
-0.0133250000000001));
#46420=CARTESIAN_POINT('Ctrl Pts',(-0.0650390110357168,-0.0576248795174292,
-0.0133250000000001));
#46421=CARTESIAN_POINT('Ctrl Pts',(-0.0623280400111939,-0.0599498046813196,
-0.0133250000000003));
#46422=CARTESIAN_POINT('Ctrl Pts',(-0.0594904268278414,-0.0620765235258152,
-0.0133250000000003));
#46423=CARTESIAN_POINT('Ctrl Pts',(-0.0573688668117999,-0.0636665787498022,
-0.0133250000000003));
#46424=CARTESIAN_POINT('Ctrl Pts',(-0.0551746319546616,-0.0651481417695435,
-0.0133250000000003));
#46425=CARTESIAN_POINT('Ctrl Pts',(-0.0529107688590407,-0.0665124204372184,
-0.0133250000000003));
#46426=CARTESIAN_POINT('Ctrl Pts',(-0.0488178690201689,-0.0689789370520721,
-0.0133250000000003));
#46427=CARTESIAN_POINT('Ctrl Pts',(-0.044497278097604,-0.0710627972144308,
-0.0133250000000002));
#46428=CARTESIAN_POINT('Ctrl Pts',(-0.040004671478209,-0.0727554835895005,
-0.0133250000000002));
#46429=CARTESIAN_POINT('Ctrl Pts',(-0.0368908382283995,-0.0739286873802436,
-0.0133250000000002));
#46430=CARTESIAN_POINT('Ctrl Pts',(-0.0336895004235565,-0.0749142680218583,
-0.0133249999999998));
#46431=CARTESIAN_POINT('Ctrl Pts',(-0.0304486889041091,-0.0757008149597433,
-0.013325));
#46432=CARTESIAN_POINT('Ctrl Pts',(-0.0259717963066162,-0.0767873595312704,
-0.0133250000000001));
#46433=CARTESIAN_POINT('Ctrl Pts',(-0.0214104423515735,-0.0774991875316017,
-0.0133250000000001));
#46434=CARTESIAN_POINT('Ctrl Pts',(-0.0168162976082181,-0.0778292284117383,
-0.013325));
#46435=CARTESIAN_POINT('Ctrl Pts',(-0.0135048506864013,-0.0780671209723031,
-0.0133249999999999));
#46436=CARTESIAN_POINT('Ctrl Pts',(-0.0101763407192596,-0.078106396707891,
-0.0133250000000004));
#46437=CARTESIAN_POINT('Ctrl Pts',(-0.00685168166603567,-0.0779406634282734,
-0.0133250000000005));
#46438=CARTESIAN_POINT('Ctrl Pts',(-0.0044924871884174,-0.0778230582748511,
-0.0133250000000006));
#46439=CARTESIAN_POINT('Ctrl Pts',(-0.00213599500253028,-0.0776018117801322,
-0.013325));
#46440=CARTESIAN_POINT('Ctrl Pts',(0.000197121312828762,-0.0772768152441007,
-0.013325));
#46441=CARTESIAN_POINT('Ctrl Pts',(0.00625486133427826,-0.0764329891089909,
-0.0133250000000001));
#46442=CARTESIAN_POINT('Ctrl Pts',(0.0121811594338303,-0.0748919729606164,
-0.0133250000000003));
#46443=CARTESIAN_POINT('Ctrl Pts',(0.017838523980557,-0.0726157902902942,
-0.0133250000000001));
#46444=CARTESIAN_POINT('Ctrl Pts',(0.0197116627554222,-0.0718621520929956,
-0.0133250000000001));
#46445=CARTESIAN_POINT('Ctrl Pts',(0.0215550621983123,-0.0710275991192391,
-0.0133250000000002));
#46446=CARTESIAN_POINT('Ctrl Pts',(0.0233628051714133,-0.070109837644389,
-0.0133250000000002));
#46447=CARTESIAN_POINT('Ctrl Pts',(0.0663714283216842,0.0324968229607071,
-0.962474152380794));
#46448=CARTESIAN_POINT('Ctrl Pts',(0.0556047253532112,0.0544867096396884,
-0.96036493204217));
#46449=CARTESIAN_POINT('Ctrl Pts',(0.0106964331164646,0.0865570854208283,
-0.95614649136492));
#46450=CARTESIAN_POINT('Ctrl Pts',(-0.0668730934586114,0.0561130448027703,
-0.949818830349052));
#46451=CARTESIAN_POINT('Ctrl Pts',(-0.0834262416657708,-0.0254206125080873,
-0.943491169333177));
#46452=CARTESIAN_POINT('Ctrl Pts',(-0.0242332971309306,-0.0838051103417385,
-0.937163508317307));
#46453=CARTESIAN_POINT('Ctrl Pts',(0.0570492242990965,-0.06601055836573,
-0.930835847301434));
#46454=CARTESIAN_POINT('Ctrl Pts',(0.0864315571449822,0.0118125778999351,
-0.924508186285562));
#46455=CARTESIAN_POINT('Ctrl Pts',(0.0372434277651266,0.0788901466696481,
-0.91818052526969));
#46456=CARTESIAN_POINT('Ctrl Pts',(-0.0458156426390635,0.0742413616113632,
-0.911852864253818));
#46457=CARTESIAN_POINT('Ctrl Pts',(-0.0872135427032971,0.00208880626078628,
-0.905525203237946));
#46458=CARTESIAN_POINT('Ctrl Pts',(-0.0493167351776861,-0.0719621815782819,
-0.899197542222075));
#46459=CARTESIAN_POINT('Ctrl Pts',(0.0334214198190593,-0.0805835554203335,
-0.892869881206202));
#46460=CARTESIAN_POINT('Ctrl Pts',(0.0857712573590327,-0.0159359034660176,
-0.88654222019033));
#46461=CARTESIAN_POINT('Ctrl Pts',(0.0601358128673054,0.0632010030064432,
-0.880214559174458));
#46462=CARTESIAN_POINT('Ctrl Pts',(-0.0201769626930229,0.084873857253752,
-0.873886898158586));
#46463=CARTESIAN_POINT('Ctrl Pts',(-0.0821441893694497,0.029377006100539,
-0.867559237142714));
#46464=CARTESIAN_POINT('Ctrl Pts',(-0.0694236808259852,-0.0528302204192478,
-0.861231576126843));
#46465=CARTESIAN_POINT('Ctrl Pts',(0.00641879698876544,-0.0870027483201755,
-0.85490391511097));
#46466=CARTESIAN_POINT('Ctrl Pts',(0.076425112291304,-0.0420699505040234,
-0.8485762540951));
#46467=CARTESIAN_POINT('Ctrl Pts',(0.0769435948053001,0.0411140152158757,
-0.842248593079225));
#46468=CARTESIAN_POINT('Ctrl Pts',(0.0075028148617241,0.0869159748679489,
-0.835920932063356));
#46469=CARTESIAN_POINT('Ctrl Pts',(-0.0687597312600683,0.0536915095569343,
-0.829593271047482));
#46470=CARTESIAN_POINT('Ctrl Pts',(-0.0825040163400733,-0.0283507707839517,
-0.823265610031611));
#46471=CARTESIAN_POINT('Ctrl Pts',(-0.0212333521088858,-0.0846157411642612,
-0.816937949015739));
#46472=CARTESIAN_POINT('Ctrl Pts',(0.0593432667534829,-0.0639457236824982,
-0.810610287999866));
#46473=CARTESIAN_POINT('Ctrl Pts',(0.0859633353842028,0.014865526115561,
-0.804282626983996));
#46474=CARTESIAN_POINT('Ctrl Pts',(0.0344231459854351,0.0801606257062834,
-0.797954965968122));
#46475=CARTESIAN_POINT('Ctrl Pts',(-0.0484155261201637,0.0725714525340945,
-0.791627304952252));
#46476=CARTESIAN_POINT('Ctrl Pts',(-0.0872334539001633,-0.00100170583074655,
-0.785299643936378));
#46477=CARTESIAN_POINT('Ctrl Pts',(-0.0467362966021223,-0.0736640853684918,
-0.778971982920508));
#46478=CARTESIAN_POINT('Ctrl Pts',(0.0362548028063699,-0.0793490275094065,
-0.772644321904634));
#46479=CARTESIAN_POINT('Ctrl Pts',(0.0862820260894591,-0.0128876245803302,
-0.766316660888764));
#46480=CARTESIAN_POINT('Ctrl Pts',(0.0578592289600791,0.0652915654389009,
-0.759988999872889));
#46481=CARTESIAN_POINT('Ctrl Pts',(-0.0231707900729891,0.0841058462933171,
-0.753661338857021));
#46482=CARTESIAN_POINT('Ctrl Pts',(-0.0831332816440542,0.0264487499976755,
-0.747333677841146));
#46483=CARTESIAN_POINT('Ctrl Pts',(-0.0675086789221911,-0.0552562861900129,
-0.741006016825276));
#46484=CARTESIAN_POINT('Ctrl Pts',(0.00949669427259201,-0.0867207685115116,
-0.734678355809403));
#46485=CARTESIAN_POINT('Ctrl Pts',(0.0778674086249794,-0.0393363135965772,
-0.728350694793532));
#46486=CARTESIAN_POINT('Ctrl Pts',(0.0754389070476233,0.0438138128538845,
-0.722023033777659));
#46487=CARTESIAN_POINT('Ctrl Pts',(0.00441925078978631,0.0871272007801963,
-0.715695372761787));
#46488=CARTESIAN_POINT('Ctrl Pts',(-0.070618511328248,0.0512221119353569,
-0.709367711745916));
#46489=CARTESIAN_POINT('Ctrl Pts',(-0.0814479567647437,-0.0312555472225994,
-0.703040050730043));
#46490=CARTESIAN_POINT('Ctrl Pts',(-0.0182226522121619,-0.0853147926193951,
-0.696712389714172));
#46491=CARTESIAN_POINT('Ctrl Pts',(0.0615711950922978,-0.0618034532064518,
-0.690384728698299));
#46492=CARTESIAN_POINT('Ctrl Pts',(0.0853827975350567,0.0179013066121811,
-0.684057067682429));
#46493=CARTESIAN_POINT('Ctrl Pts',(0.0315619832053435,0.0813297000454412,
-0.677729406666555));
#46494=CARTESIAN_POINT('Ctrl Pts',(-0.0509558650129233,0.0708108657913499,
-0.671401745650684));
#46495=CARTESIAN_POINT('Ctrl Pts',(-0.087143222032879,-0.00409117917771768,
-0.665074084634812));
#46496=CARTESIAN_POINT('Ctrl Pts',(-0.044097535312672,-0.0752734101305599,
-0.65874642361894));
#46497=CARTESIAN_POINT('Ctrl Pts',(0.0390428582906939,-0.0780149608077107,
-0.652418762603067));
#46498=CARTESIAN_POINT('Ctrl Pts',(0.0866843980931254,-0.00982313700242362,
-0.646091101587197));
#46499=CARTESIAN_POINT('Ctrl Pts',(0.0555100696561328,0.0673001564642097,
-0.639763440571324));
#46500=CARTESIAN_POINT('Ctrl Pts',(-0.0261355596403159,0.0832322738823306,
-0.633435779555452));
#46501=CARTESIAN_POINT('Ctrl Pts',(-0.0840180104376559,0.0234872905085658,
-0.62710811853958));
#46502=CARTESIAN_POINT('Ctrl Pts',(-0.0655089468902942,-0.0576129913358129,
-0.620780457523708));
#46503=CARTESIAN_POINT('Ctrl Pts',(0.012562675089579,-0.0863299373793905,
-0.614452796507836));
#46504=CARTESIAN_POINT('Ctrl Pts',(0.0792119631042182,-0.0365533007334742,
-0.608125135491964));
#46505=CARTESIAN_POINT('Ctrl Pts',(0.0738395288211365,0.0464586146673402,
-0.601797474476092));
#46506=CARTESIAN_POINT('Ctrl Pts',(0.00133013907144687,0.0872290640978479,
-0.59546981346022));
#46507=CARTESIAN_POINT('Ctrl Pts',(-0.0723886501561355,0.0486884197926824,
-0.589142152444349));
#46508=CARTESIAN_POINT('Ctrl Pts',(-0.0802896631951301,-0.0341210913856576,
-0.582814491428475));
#46509=CARTESIAN_POINT('Ctrl Pts',(-0.0151890790080958,-0.0859067562664407,
-0.576486830412606));
#46510=CARTESIAN_POINT('Ctrl Pts',(0.0637218387120179,-0.0595836065079599,
-0.570159169396731));
#46511=CARTESIAN_POINT('Ctrl Pts',(0.0846950865125139,0.0209146172322998,
-0.563831508380862));
#46512=CARTESIAN_POINT('Ctrl Pts',(0.0286612035496907,0.0823966886738722,
-0.557503847364987));
#46513=CARTESIAN_POINT('Ctrl Pts',(-0.053432243674384,0.0689613966597043,
-0.551176186349117));
#46514=CARTESIAN_POINT('Ctrl Pts',(-0.0869436072730663,-0.00717551724147037,
-0.544848525333244));
#46515=CARTESIAN_POINT('Ctrl Pts',(-0.0414034224289421,-0.076788251083785,
-0.538520864317373));
#46516=CARTESIAN_POINT('Ctrl Pts',(0.0417819068541502,-0.0765829690790775,
-0.532193203301501));
#46517=CARTESIAN_POINT('Ctrl Pts',(0.0869779631209978,-0.00674631934155149,
-0.525865542285629));
#46518=CARTESIAN_POINT('Ctrl Pts',(0.0530912336515535,0.0692242717743709,
-0.519537881269757));
#46519=CARTESIAN_POINT('Ctrl Pts',(-0.0290675236360216,0.0822542276299836,
-0.513210220253885));
#46520=CARTESIAN_POINT('Ctrl Pts',(-0.0847972791269669,0.0204963495774027,
-0.506882559238013));
#46521=CARTESIAN_POINT('Ctrl Pts',(-0.0634269874842546,-0.0598973801764987,
-0.500554898222141));
#46522=CARTESIAN_POINT('Ctrl Pts',(0.015612887132456,-0.0858307441930048,
-0.494227237206269));
#46523=CARTESIAN_POINT('Ctrl Pts',(0.0804570900696259,-0.0337244058637655,
-0.487899576190397));
#46524=CARTESIAN_POINT('Ctrl Pts',(0.0721474666049248,0.0490451012418884,
-0.481571915174525));
#46525=CARTESIAN_POINT('Ctrl Pts',(-0.00176064224849756,0.087221436769917,
-0.475244254158653));
#46526=CARTESIAN_POINT('Ctrl Pts',(-0.0740679261492535,0.04609361354119,
-0.468916593142781));
#46527=CARTESIAN_POINT('Ctrl Pts',(-0.0790305893735705,-0.0369438064714765,
-0.462588932126909));
#46528=CARTESIAN_POINT('Ctrl Pts',(-0.0121364403459336,-0.0863908890396749,
-0.456261271111038));
#46529=CARTESIAN_POINT('Ctrl Pts',(0.0657924981506585,-0.0572889699718141,
-0.449933610095165));
#46530=CARTESIAN_POINT('Ctrl Pts',(0.0839010655140964,0.0239016756511994,
-0.443605949079294));
#46531=CARTESIAN_POINT('Ctrl Pts',(0.0257244481133483,0.0833602522944807,
-0.437278288063421));
#46532=CARTESIAN_POINT('Ctrl Pts',(-0.0558415537398982,0.0670253666103355,
-0.43095062704755));
#46533=CARTESIAN_POINT('Ctrl Pts',(-0.0866348601754494,-0.0102508485363977,
-0.424622966031677));
#46534=CARTESIAN_POINT('Ctrl Pts',(-0.0386573396255769,-0.078206706786622,
-0.418295305015806));
#46535=CARTESIAN_POINT('Ctrl Pts',(0.0444685104211786,-0.0750548497717326,
-0.411967643999933));
#46536=CARTESIAN_POINT('Ctrl Pts',(0.0871623526873201,-0.00366103364462123,
-0.405639982984062));
#46537=CARTESIAN_POINT('Ctrl Pts',(0.0506057570896398,0.0710614962037825,
-0.399312321968189));
#46538=CARTESIAN_POINT('Ctrl Pts',(-0.0319630018346919,0.081172935188099,
-0.392984660952318));
#46539=CARTESIAN_POINT('Ctrl Pts',(-0.085470109567385,0.0174796814580538,
-0.386656999936446));
#46540=CARTESIAN_POINT('Ctrl Pts',(-0.0612654139968446,-0.0621065853282167,
-0.380329338920573));
#46541=CARTESIAN_POINT('Ctrl Pts',(0.0186435017497599,-0.0852238155437934,
-0.374001677904702));
#46542=CARTESIAN_POINT('Ctrl Pts',(0.0816012266274847,-0.0308531798397786,
-0.367674016888829));
#46543=CARTESIAN_POINT('Ctrl Pts',(0.0703648442895387,0.0515700259981008,
-0.361346355872959));
#46544=CARTESIAN_POINT('Ctrl Pts',(-0.0048492135956714,0.0871043283702904,
-0.355018694857085));
#46545=CARTESIAN_POINT('Ctrl Pts',(-0.0756542314664302,0.043440950203232,
-0.348691033841215));
#46546=CARTESIAN_POINT('Ctrl Pts',(-0.0776723156999812,-0.039720149384642,
-0.342363372825342));
#46547=CARTESIAN_POINT('Ctrl Pts',(-0.00906856792307098,-0.086766583251621,
-0.33603571180947));
#46548=CARTESIAN_POINT('Ctrl Pts',(0.0677805742992985,-0.0549224238448479,
-0.329708050793598));
#46549=CARTESIAN_POINT('Ctrl Pts',(0.0830017312015545,0.0268587324883495,
-0.323380389777726));
#46550=CARTESIAN_POINT('Ctrl Pts',(0.0227554031361251,0.0842191814342093,
-0.317052728761854));
#46551=CARTESIAN_POINT('Ctrl Pts',(-0.0581807710234661,0.0650052057642372,
-0.310725067745983));
#46552=CARTESIAN_POINT('Ctrl Pts',(-0.0862173682819487,-0.0133133128811225,
-0.30439740673011));
#46553=CARTESIAN_POINT('Ctrl Pts',(-0.0358627338085138,-0.0795269967816936,
-0.298069745714238));
#46554=CARTESIAN_POINT('Ctrl Pts',(0.0470992967446723,-0.0734325209937202,
-0.291742084698366));
#46555=CARTESIAN_POINT('Ctrl Pts',(0.0872373353447779,-0.000571152587860333,
-0.285414423682494));
#46556=CARTESIAN_POINT('Ctrl Pts',(0.0480567597612106,0.0728095236530848,
-0.279086762666623));
#46557=CARTESIAN_POINT('Ctrl Pts',(-0.0348183598080465,0.0799897538039288,
-0.27275910165075));
#46558=CARTESIAN_POINT('Ctrl Pts',(-0.0860356572165558,0.0144410726973928,
-0.266431440634879));
#46559=CARTESIAN_POINT('Ctrl Pts',(-0.0590269396530525,-0.0642378337783162,
-0.260103779619007));
#46560=CARTESIAN_POINT('Ctrl Pts',(0.0216507148888523,-0.0845099132536343,
-0.253776118603134));
#46561=CARTESIAN_POINT('Ctrl Pts',(0.0826429366480972,-0.0279432266482656,
-0.247448457587263));
#46562=CARTESIAN_POINT('Ctrl Pts',(0.0684938994372912,0.0540302196294675,
-0.241120796571391));
#46563=CARTESIAN_POINT('Ctrl Pts',(-0.00793169816963801,0.0868778858943854,
-0.234793135555519));
#46564=CARTESIAN_POINT('Ctrl Pts',(-0.077145574964127,0.0407337594238917,
-0.228465474539647));
#46565=CARTESIAN_POINT('Ctrl Pts',(-0.0762165470906266,-0.0424466352365409,
-0.222137813523775));
#46566=CARTESIAN_POINT('Ctrl Pts',(-0.00598931255869429,-0.0870333673276597,
-0.215810152507903));
#46567=CARTESIAN_POINT('Ctrl Pts',(0.0696835717087142,-0.0524869386356467,
-0.209482491492031));
#46568=CARTESIAN_POINT('Ctrl Pts',(0.0819982124259003,0.0297820760219009,
-0.203154830476159));
#46569=CARTESIAN_POINT('Ctrl Pts',(0.0197577953896086,0.0849723979572207,
-0.196827169460287));
#46570=CARTESIAN_POINT('Ctrl Pts',(-0.0604469593233129,0.062903449845688,
-0.190499508444415));
#46571=CARTESIAN_POINT('Ctrl Pts',(-0.085691655625816,-0.0163590662480221,
-0.184171847428543));
#46572=CARTESIAN_POINT('Ctrl Pts',(-0.0330231128016351,-0.0807474638242463,
-0.177844186412671));
#46573=CARTESIAN_POINT('Ctrl Pts',(0.0496709636615209,-0.0717180191165734,
-0.171516525396799));
#46574=CARTESIAN_POINT('Ctrl Pts',(0.0872028169333057,0.00251944540519899,
-0.165188864380927));
#46575=CARTESIAN_POINT('Ctrl Pts',(0.0454474412670434,0.0744661599442045,
-0.158861203365055));
#46576=CARTESIAN_POINT('Ctrl Pts',(-0.0376300136353005,0.078706168691497,
-0.152533542349183));
#46577=CARTESIAN_POINT('Ctrl Pts',(-0.0864932119131863,0.0113843372402568,
-0.146205881333311));
#46578=CARTESIAN_POINT('Ctrl Pts',(-0.0567143747377854,-0.0662884500965085,
-0.139878220317439));
#46579=CARTESIAN_POINT('Ctrl Pts',(0.0246307528823777,-0.083689933929838,
-0.133550559301567));
#46580=CARTESIAN_POINT('Ctrl Pts',(0.0835809106498128,-0.0249981979169972,
-0.127222898285695));
#46581=CARTESIAN_POINT('Ctrl Pts',(0.0665369841126368,0.0564225922414199,
-0.120895237269823));
#46582=CARTESIAN_POINT('Ctrl Pts',(-0.0110042337120753,0.0865423970628537,
-0.114567576253952));
#46583=CARTESIAN_POINT('Ctrl Pts',(-0.0785400716048779,0.0379754326755566,
-0.108239915238079));
#46584=CARTESIAN_POINT('Ctrl Pts',(-0.0746651356672856,-0.0451198291711274,
-0.101912254222208));
#46585=CARTESIAN_POINT('Ctrl Pts',(-0.00290249226713311,-0.0871909301984517,
-0.0955845932063355));
#46586=CARTESIAN_POINT('Ctrl Pts',(0.0714990124011491,-0.0499855262439841,
-0.0892569321904637));
#46587=CARTESIAN_POINT('Ctrl Pts',(0.0808919382230671,0.032667951227759,
-0.0829292711745915));
#46588=CARTESIAN_POINT('Ctrl Pts',(0.0167350661775352,0.0856191188118938,
-0.0766016101587197));
#46589=CARTESIAN_POINT('Ctrl Pts',(-0.0626366646621712,0.0607224289900663,
-0.0702739491428476));
#46590=CARTESIAN_POINT('Ctrl Pts',(-0.0850595379996997,-0.0193837013910442,
-0.0639462881269757));
#46591=CARTESIAN_POINT('Ctrl Pts',(-0.0301398485007547,-0.0818676840127184,
-0.0576186271111039));
#46592=CARTESIAN_POINT('Ctrl Pts',(0.0521761247033908,-0.0699113944796167,
-0.0512909660952318));
#46593=CARTESIAN_POINT('Ctrl Pts',(0.0870667295313287,0.00560289368117736,
-0.04496330507936));
#46594=CARTESIAN_POINT('Ctrl Pts',(0.0427661024466595,0.0760368969037317,
-0.0386356440634878));
#46595=CARTESIAN_POINT('Ctrl Pts',(-0.0403659317628278,0.0773093583706435,
-0.032307983047616));
#46596=CARTESIAN_POINT('Ctrl Pts',(-0.0868971070713012,0.00834129536707174,
-0.025980322031744));
#46597=CARTESIAN_POINT('Ctrl Pts',(-0.0542193581796284,-0.0683140096653152,
-0.0196526610158722));
#46598=CARTESIAN_POINT('Ctrl Pts',(0.00013432532901024,-0.0778502984302035,
-0.015434220338624));
#46599=CARTESIAN_POINT('Ctrl Pts',(0.0233628051714152,-0.0701098376443883,
-0.013325));
#46600=CARTESIAN_POINT('Ctrl Pts',(0.0731896930038058,0.0358351862576404,
-0.958091101587196));
#46601=CARTESIAN_POINT('Ctrl Pts',(0.0613169383433753,0.0600840700909465,
-0.955981881248572));
#46602=CARTESIAN_POINT('Ctrl Pts',(0.0117952660629124,0.0954490007138341,
-0.951763440571324));
#46603=CARTESIAN_POINT('Ctrl Pts',(-0.0737428936549124,0.0618774768974165,
-0.945435779555452));
#46604=CARTESIAN_POINT('Ctrl Pts',(-0.0919965287832173,-0.02803204439745,
-0.93910811853958));
#46605=CARTESIAN_POINT('Ctrl Pts',(-0.0267227574022744,-0.0924143182264165,
-0.932780457523708));
#46606=CARTESIAN_POINT('Ctrl Pts',(0.0629098290957223,-0.0727917512695617,
-0.926452796507837));
#46607=CARTESIAN_POINT('Ctrl Pts',(0.0953105770546664,0.0130260711866786,
-0.920125135491964));
#46608=CARTESIAN_POINT('Ctrl Pts',(0.0410694046137993,0.086994445679126,
-0.913797474476093));
#46609=CARTESIAN_POINT('Ctrl Pts',(-0.0505222338032704,0.0818680959852864,
-0.907469813460219));
#46610=CARTESIAN_POINT('Ctrl Pts',(-0.0961728951393259,0.00230338705731037,
-0.901142152444349));
#46611=CARTESIAN_POINT('Ctrl Pts',(-0.0543829897725069,-0.0793547782649999,
-0.894814491428476));
#46612=CARTESIAN_POINT('Ctrl Pts',(0.0368547659461639,-0.0888618164699416,
-0.888486830412605));
#46613=CARTESIAN_POINT('Ctrl Pts',(0.0945824453894882,-0.0175729815058846,
-0.882159169396731));
#46614=CARTESIAN_POINT('Ctrl Pts',(0.0663134995522529,0.0696935733423554,
-0.875831508380861));
#46615=CARTESIAN_POINT('Ctrl Pts',(-0.0222497201370175,0.093592856346915,
-0.869503847364988));
#46616=CARTESIAN_POINT('Ctrl Pts',(-0.0905827726481562,0.0323948740028382,
-0.863176186349117));
#46617=CARTESIAN_POINT('Ctrl Pts',(-0.0765555000899085,-0.0582574115335841,
-0.856848525333245));
#46618=CARTESIAN_POINT('Ctrl Pts',(0.00707819302583869,-0.0959404460783713,
-0.850520864317372));
#46619=CARTESIAN_POINT('Ctrl Pts',(0.0842761809987215,-0.0463917507869694,
-0.844193203301502));
#46620=CARTESIAN_POINT('Ctrl Pts',(0.0848479266577615,0.0453376133058242,
-0.837865542285628));
#46621=CARTESIAN_POINT('Ctrl Pts',(0.00827357087649971,0.0958447584837249,
-0.831537881269757));
#46622=CARTESIAN_POINT('Ctrl Pts',(-0.0758233437068345,0.0592071799681169,
-0.825210220253884));
#46623=CARTESIAN_POINT('Ctrl Pts',(-0.0909795642523203,-0.0312632146477519,
-0.818882559238014));
#46624=CARTESIAN_POINT('Ctrl Pts',(-0.0234146312892188,-0.093308224272137,
-0.812554898222141));
#46625=CARTESIAN_POINT('Ctrl Pts',(0.0654395360376984,-0.0705147983639095,
-0.806227237206269));
#46626=CARTESIAN_POINT('Ctrl Pts',(0.0947942553813848,0.0163926454537744,
-0.799899576190397));
#46627=CARTESIAN_POINT('Ctrl Pts',(0.0379593983526802,0.0883954396461148,
-0.793571915174525));
#46628=CARTESIAN_POINT('Ctrl Pts',(-0.0533892004881688,0.0800266389637921,
-0.787244254158654));
#46629=CARTESIAN_POINT('Ctrl Pts',(-0.0961948517918018,-0.00110460998183024,
-0.780916593142781));
#46630=CARTESIAN_POINT('Ctrl Pts',(-0.0515374655471529,-0.0812315167815159,
-0.774588932126909));
#46631=CARTESIAN_POINT('Ctrl Pts',(0.039979219287719,-0.0875004668487241,
-0.768261271111037));
#46632=CARTESIAN_POINT('Ctrl Pts',(0.0951456848363578,-0.0142115562439161,
-0.761933610095165));
#46633=CARTESIAN_POINT('Ctrl Pts',(0.0638030446550082,0.0719988969809441,
-0.755605949079294));
#46634=CARTESIAN_POINT('Ctrl Pts',(-0.0255511001492739,0.0927459484553843,
-0.74927828806342));
#46635=CARTESIAN_POINT('Ctrl Pts',(-0.0916734732969335,0.0291658013337019,
-0.74295062704755));
#46636=CARTESIAN_POINT('Ctrl Pts',(-0.0744437721222492,-0.0609327044037141,
-0.736622966031678));
#46637=CARTESIAN_POINT('Ctrl Pts',(0.0104722793517905,-0.0956294987904907,
-0.730295305015805));
#46638=CARTESIAN_POINT('Ctrl Pts',(0.0858666428669004,-0.0433772903316337,
-0.723967643999934));
#46639=CARTESIAN_POINT('Ctrl Pts',(0.0831886639624164,0.0483147582203582,
-0.717639982984062));
#46640=CARTESIAN_POINT('Ctrl Pts',(0.00487323561945417,0.0960776834043234,
-0.71131232196819));
#46641=CARTESIAN_POINT('Ctrl Pts',(-0.0778730742308229,0.0564841038132446,
-0.704984660952317));
#46642=CARTESIAN_POINT('Ctrl Pts',(-0.0898150168248115,-0.0344663956122913,
-0.698656999936446));
#46643=CARTESIAN_POINT('Ctrl Pts',(-0.0200946454648996,-0.0940790885233498,
-0.692329338920573));
#46644=CARTESIAN_POINT('Ctrl Pts',(0.0678963370328801,-0.0681524547706237,
-0.686001677904703));
#46645=CARTESIAN_POINT('Ctrl Pts',(0.0941540795100721,0.0197402883807532,
-0.679674016888829));
#46646=CARTESIAN_POINT('Ctrl Pts',(0.03480431143043,0.0896846117212867,
-0.673346355872958));
#46647=CARTESIAN_POINT('Ctrl Pts',(-0.0561905056338947,0.0780851890588194,
-0.667018694857086));
#46648=CARTESIAN_POINT('Ctrl Pts',(-0.0960953505028781,-0.00451146156730964,
-0.660691033841214));
#46649=CARTESIAN_POINT('Ctrl Pts',(-0.0486276271789151,-0.0830061657269673,
-0.654363372825342));
#46650=CARTESIAN_POINT('Ctrl Pts',(0.0430536886811791,-0.0860293529249665,
-0.648035711809471));
#46651=CARTESIAN_POINT('Ctrl Pts',(0.0955893920785604,-0.0108322571883965,
-0.641708050793598));
#46652=CARTESIAN_POINT('Ctrl Pts',(0.0612125587694319,0.0742138283788349,
-0.635380389777726));
#46653=CARTESIAN_POINT('Ctrl Pts',(-0.0288204372713859,0.091782634900238,
-0.629052728761854));
#46654=CARTESIAN_POINT('Ctrl Pts',(-0.0926490893177534,0.0259001143305441,
-0.622725067745983));
#46655=CARTESIAN_POINT('Ctrl Pts',(-0.0722386097925335,-0.063531511307275,
-0.61639740673011));
#46656=CARTESIAN_POINT('Ctrl Pts',(0.0138532250452181,-0.0951985180010217,
-0.610069745714238));
#46657=CARTESIAN_POINT('Ctrl Pts',(0.0873493219661874,-0.0403083815823909,
-0.603742084698366));
#46658=CARTESIAN_POINT('Ctrl Pts',(0.0814249833493339,0.0512312576490662,
-0.597414423682494));
#46659=CARTESIAN_POINT('Ctrl Pts',(0.00146678281232274,0.0961900110298664,
-0.591086762666623));
#46660=CARTESIAN_POINT('Ctrl Pts',(-0.0798250574962617,0.0536901282310149,
-0.58475910165075));
#46661=CARTESIAN_POINT('Ctrl Pts',(-0.0885377330159198,-0.0376263140122176,
-0.578431440634879));
#46662=CARTESIAN_POINT('Ctrl Pts',(-0.0167494365832395,-0.0947318639523595,
-0.572103779619006));
#46663=CARTESIAN_POINT('Ctrl Pts',(0.0702679139337871,-0.0657045656338903,
-0.565776118603135));
#46664=CARTESIAN_POINT('Ctrl Pts',(0.0933957206817628,0.0230631531252437,
-0.559448457587262));
#46665=CARTESIAN_POINT('Ctrl Pts',(0.031605537834058,0.0908612109316414,
-0.553120796571392));
#46666=CARTESIAN_POINT('Ctrl Pts',(-0.0589212799832885,0.0760457259737537,
-0.546793135555518));
#46667=CARTESIAN_POINT('Ctrl Pts',(-0.095875229535782,-0.00791265032750778,
-0.540465474539648));
#46668=CARTESIAN_POINT('Ctrl Pts',(-0.0456567510072874,-0.0846766246446023,
-0.534137813523774));
#46669=CARTESIAN_POINT('Ctrl Pts',(0.046074116726064,-0.0844502542427039,
-0.527810152507903));
#46670=CARTESIAN_POINT('Ctrl Pts',(0.0959131147226248,-0.00743936139389169,
-0.521482491492031));
#46671=CARTESIAN_POINT('Ctrl Pts',(0.058545238371509,0.0763356059631905,
-0.515154830476159));
#46672=CARTESIAN_POINT('Ctrl Pts',(-0.0320535987411656,0.0907041150195771,
-0.508827169460288));
#46673=CARTESIAN_POINT('Ctrl Pts',(-0.0935084114324098,0.0226019172888386,
-0.502499508444415));
#46674=CARTESIAN_POINT('Ctrl Pts',(-0.0699427729599149,-0.0660505729303092,
-0.496171847428543));
#46675=CARTESIAN_POINT('Ctrl Pts',(0.0172167820555128,-0.0946480432412487,
-0.489844186412671));
#46676=CARTESIAN_POINT('Ctrl Pts',(0.0887223594712305,-0.0371888774178803,
-0.483516525396799));
#46677=CARTESIAN_POINT('Ctrl Pts',(0.0795590974210148,0.0540834511777658,
-0.477188864380928));
#46678=CARTESIAN_POINT('Ctrl Pts',(-0.00194151111277164,0.0961816001548283,
-0.470861203365055));
#46679=CARTESIAN_POINT('Ctrl Pts',(-0.081676843686688,0.0508287603540027,
-0.464533542349184));
#46680=CARTESIAN_POINT('Ctrl Pts',(-0.0871493159093535,-0.0407390035503574,
-0.458205881333311));
#46681=CARTESIAN_POINT('Ctrl Pts',(-0.0133832036696982,-0.0952657311591092,
-0.45187822031744));
#46682=CARTESIAN_POINT('Ctrl Pts',(0.0725512899656393,-0.0631742035807814,
-0.445550559301567));
#46683=CARTESIAN_POINT('Ctrl Pts',(0.0925201307693222,0.0263570688084213,
-0.439222898285696));
#46684=CARTESIAN_POINT('Ctrl Pts',(0.0283670927041534,0.0919237603955488,
-0.432895237269823));
#46685=CARTESIAN_POINT('Ctrl Pts',(-0.0615780958527814,0.0739108096619836,
-0.426567576253952));
#46686=CARTESIAN_POINT('Ctrl Pts',(-0.0955347651844519,-0.0113039070633101,
-0.420239915238079));
#46687=CARTESIAN_POINT('Ctrl Pts',(-0.0426285661026744,-0.0862407967598531,
-0.413912254222208));
#46688=CARTESIAN_POINT('Ctrl Pts',(0.0490367121570486,-0.0827651529000646,
-0.407584593206335));
#46689=CARTESIAN_POINT('Ctrl Pts',(0.096116446428654,-0.00403712765118974,
-0.401256932190464));
#46690=CARTESIAN_POINT('Ctrl Pts',(0.0558044315042385,0.0783615664610724,
-0.394929271174592));
#46691=CARTESIAN_POINT('Ctrl Pts',(-0.0352465262676424,0.0895117425805614,
-0.388601610158719));
#46692=CARTESIAN_POINT('Ctrl Pts',(-0.0942503610125686,0.0192753501328719,
-0.382273949142848));
#46693=CARTESIAN_POINT('Ctrl Pts',(-0.0675591433778916,-0.0684867273257366,
-0.375946288126975));
#46694=CARTESIAN_POINT('Ctrl Pts',(0.0205587284180089,-0.0939787654716684,
-0.369618627111104));
#46695=CARTESIAN_POINT('Ctrl Pts',(0.0899840319339393,-0.0340226934656285,
-0.363290966095232));
#46696=CARTESIAN_POINT('Ctrl Pts',(0.0775933482529769,0.0568677587094528,
-0.356963305079361));
#46697=CARTESIAN_POINT('Ctrl Pts',(-0.005347368036995,0.0960524613366115,
-0.350635644063487));
#46698=CARTESIAN_POINT('Ctrl Pts',(-0.0834261084246978,0.0479035917949261,
-0.344307983047617));
#46699=CARTESIAN_POINT('Ctrl Pts',(-0.0856515082577939,-0.043800557152956,
-0.337980322031744));
#46700=CARTESIAN_POINT('Ctrl Pts',(-0.0100001720477796,-0.0956800200290485,
-0.331652661015872));
#46701=CARTESIAN_POINT('Ctrl Pts',(0.0747435990158817,-0.0605645447427567,
-0.325325));
#46702=CARTESIAN_POINT('Ctrl Pts',(0.0915284088204783,0.0296179008799696,
-0.318997338984128));
#46703=CARTESIAN_POINT('Ctrl Pts',(0.0250930409639339,0.0928709263920988,
-0.312669677968256));
#46704=CARTESIAN_POINT('Ctrl Pts',(-0.0641576183850333,0.0716831198881908,
-0.306342016952384));
#46705=CARTESIAN_POINT('Ctrl Pts',(-0.0950743848025683,-0.0146809750411026,
-0.300014355936512));
#46706=CARTESIAN_POINT('Ctrl Pts',(-0.0395468734679134,-0.0876967187108911,
-0.293686694920641));
#46707=CARTESIAN_POINT('Ctrl Pts',(0.0519377562997463,-0.0809761640502468,
-0.287359033904768));
#46708=CARTESIAN_POINT('Ctrl Pts',(0.0961991319730023,-0.00062982647233715,
-0.281031372888897));
#46709=CARTESIAN_POINT('Ctrl Pts',(0.0529935784511589,0.0802891668700402,
-0.274703711873025));
#46710=CARTESIAN_POINT('Ctrl Pts',(-0.0383952120616697,0.0882070142589782,
-0.268376050857152));
#46711=CARTESIAN_POINT('Ctrl Pts',(-0.0948740067569576,0.0159245883973617,
-0.26204838984128));
#46712=CARTESIAN_POINT('Ctrl Pts',(-0.0650907129981055,-0.0708369166123314,
-0.255720728825409));
#46713=CARTESIAN_POINT('Ctrl Pts',(0.0238748692938754,-0.093191524775292,
-0.249393067809537));
#46714=CARTESIAN_POINT('Ctrl Pts',(0.0911327556925737,-0.0308138039460294,
-0.243065406793665));
#46715=CARTESIAN_POINT('Ctrl Pts',(0.075530203269877,0.0595806853582052,
-0.236737745777793));
#46716=CARTESIAN_POINT('Ctrl Pts',(-0.00874651290041614,0.0958027566713121,
-0.230410084761921));
#46717=CARTESIAN_POINT('Ctrl Pts',(-0.0850706560187414,0.0449182942496883,
-0.224082423746049));
#46718=CARTESIAN_POINT('Ctrl Pts',(-0.0840461901217001,-0.0468071319325816,
-0.217754762730177));
#46719=CARTESIAN_POINT('Ctrl Pts',(-0.00660458812713927,-0.0959742105432099,
-0.211427101714305));
#46720=CARTESIAN_POINT('Ctrl Pts',(0.0768420892805049,-0.0578788647855197,
-0.205099440698433));
#46721=CARTESIAN_POINT('Ctrl Pts',(0.0904217996518807,0.0328415563168887,
-0.198771779682561));
#46722=CARTESIAN_POINT('Ctrl Pts',(0.0217874922321812,0.0937015200297318,
-0.192444118666689));
#46723=CARTESIAN_POINT('Ctrl Pts',(-0.0666566097454531,0.0693654528688523,
-0.186116457650817));
#46724=CARTESIAN_POINT('Ctrl Pts',(-0.0944946662567494,-0.0180396153404836,
-0.179788796634945));
#46725=CARTESIAN_POINT('Ctrl Pts',(-0.0364155412818212,-0.0890425630060109,
-0.173461135619073));
#46726=CARTESIAN_POINT('Ctrl Pts',(0.0547736077634206,-0.079085533259018,
-0.167133474603201));
#46727=CARTESIAN_POINT('Ctrl Pts',(0.0961610675226428,0.00277826529290049,
-0.160805813587329));
#46728=CARTESIAN_POINT('Ctrl Pts',(0.0501162075045576,0.0821159876064926,
-0.154478152571457));
#46729=CARTESIAN_POINT('Ctrl Pts',(-0.0414957040301764,0.0867915678432734,
-0.148150491555585));
#46730=CARTESIAN_POINT('Ctrl Pts',(-0.0953785655501859,0.0125538378295524,
-0.141822830539713));
#46731=CARTESIAN_POINT('Ctrl Pts',(-0.0625405808029773,-0.0730981905157598,
-0.135495169523841));
#46732=CARTESIAN_POINT('Ctrl Pts',(0.0271610433510118,-0.0922873098669243,
-0.129167508507969));
#46733=CARTESIAN_POINT('Ctrl Pts',(0.0921670867438566,-0.0275662356146048,
-0.122839847492097));
#46734=CARTESIAN_POINT('Ctrl Pts',(0.0733722561611948,0.0622188238079439,
-0.116512186476225));
#46735=CARTESIAN_POINT('Ctrl Pts',(-0.0121346866791143,0.0954328034368117,
-0.110184525460353));
#46736=CARTESIAN_POINT('Ctrl Pts',(-0.0866084077835025,0.0418766075929485,
-0.103856864444482));
#46737=CARTESIAN_POINT('Ctrl Pts',(-0.0823354038893083,-0.0497549401741605,
-0.0975292034286096));
#46738=CARTESIAN_POINT('Ctrl Pts',(-0.00320066214256808,-0.0961479596764388,
-0.0912015424127376));
#46739=CARTESIAN_POINT('Ctrl Pts',(0.0788440282217904,-0.0551204850180334,
-0.0848738813968658));
#46740=CARTESIAN_POINT('Ctrl Pts',(0.089201879102771,0.0360238943455408,
-0.0785462203809937));
#46741=CARTESIAN_POINT('Ctrl Pts',(0.018454241334023,0.0944146778147846,
-0.0722185593651218));
#46742=CARTESIAN_POINT('Ctrl Pts',(-0.069071261133443,0.0669603781116214,
-0.0658908983492497));
#46743=CARTESIAN_POINT('Ctrl Pts',(-0.0937976118740486,-0.0213749679638049,
-0.0595632373333777));
#46744=CARTESIAN_POINT('Ctrl Pts',(-0.0332360823735769,-0.0902778621967042,
-0.053235576317506));
#46745=CARTESIAN_POINT('Ctrl Pts',(0.0575361212758751,-0.0770933160370063,
-0.0469079153016338));
#46746=CARTESIAN_POINT('Ctrl Pts',(0.0960110000097951,0.0061784728583936,
-0.0405802542857622));
#46747=CARTESIAN_POINT('Ctrl Pts',(0.0471594176619174,0.0838480846663952,
-0.0342525932698898));
#46748=CARTESIAN_POINT('Ctrl Pts',(-0.0445126800528523,0.0852512647165678,
-0.0279249322540182));
#46749=CARTESIAN_POINT('Ctrl Pts',(-0.0958239524188379,0.00919818757268762,
-0.021597271238146));
#46750=CARTESIAN_POINT('Ctrl Pts',(-0.0597892539060201,-0.0753318336171761,
-0.0152696102222743));
#46751=CARTESIAN_POINT('Ctrl Pts',(0.000148124424040622,-0.085847774960415,
-0.0110511695450261));
#46752=CARTESIAN_POINT('Ctrl Pts',(0.0257628407500305,-0.0773121450523764,
-0.00894194920640212));
#46753=CARTESIAN_POINT('Ctrl Pts',(0.0800079576859273,0.0391735495545737,
-0.953708050793598));
#46754=CARTESIAN_POINT('Ctrl Pts',(0.0670291513335393,0.0656814305422046,
-0.951598830454974));
#46755=CARTESIAN_POINT('Ctrl Pts',(0.0128940990093602,0.10434091600684,
-0.947380389777726));
#46756=CARTESIAN_POINT('Ctrl Pts',(-0.0806126938512132,0.0676419089920627,
-0.941052728761855));
#46757=CARTESIAN_POINT('Ctrl Pts',(-0.100566815900664,-0.0306434762868126,
-0.934725067745981));
#46758=CARTESIAN_POINT('Ctrl Pts',(-0.0292122176736183,-0.101023526111094,
-0.928397406730112));
#46759=CARTESIAN_POINT('Ctrl Pts',(0.0687704338923482,-0.0795729441733933,
-0.922069745714236));
#46760=CARTESIAN_POINT('Ctrl Pts',(0.10418959696435,0.0142395644734221,
-0.915742084698368));
#46761=CARTESIAN_POINT('Ctrl Pts',(0.0448953814624721,0.0950987446886038,
-0.909414423682493));
#46762=CARTESIAN_POINT('Ctrl Pts',(-0.0552288249674775,0.0894948303592097,
-0.903086762666623));
#46763=CARTESIAN_POINT('Ctrl Pts',(-0.105132247575355,0.00251796785383443,
-0.89675910165075));
#46764=CARTESIAN_POINT('Ctrl Pts',(-0.0594492443673278,-0.086747374951718,
-0.890431440634879));
#46765=CARTESIAN_POINT('Ctrl Pts',(0.0402881120732685,-0.0971400775195495,
-0.884103779619007));
#46766=CARTESIAN_POINT('Ctrl Pts',(0.103393633419944,-0.0192100595457518,
-0.877776118603135));
#46767=CARTESIAN_POINT('Ctrl Pts',(0.0724911862372003,0.0761861436782678,
-0.871448457587262));
#46768=CARTESIAN_POINT('Ctrl Pts',(-0.0243224775810121,0.102311855440078,
-0.86512079657139));
#46769=CARTESIAN_POINT('Ctrl Pts',(-0.0990213559268627,0.0354127419051376,
-0.85879313555552));
#46770=CARTESIAN_POINT('Ctrl Pts',(-0.0836873193538318,-0.0636846026479206,
-0.852465474539646));
#46771=CARTESIAN_POINT('Ctrl Pts',(0.00773758906291201,-0.104878143836567,
-0.846137813523777));
#46772=CARTESIAN_POINT('Ctrl Pts',(0.092127249706139,-0.0507135510699152,
-0.839810152507902));
#46773=CARTESIAN_POINT('Ctrl Pts',(0.0927522585102229,0.0495612113957726,
-0.833482491492031));
#46774=CARTESIAN_POINT('Ctrl Pts',(0.00904432689127528,0.104773542099501,
-0.827154830476159));
#46775=CARTESIAN_POINT('Ctrl Pts',(-0.0828869561536006,0.0647228503792993,
-0.820827169460287));
#46776=CARTESIAN_POINT('Ctrl Pts',(-0.0994551121645673,-0.034175658511552,
-0.814499508444414));
#46777=CARTESIAN_POINT('Ctrl Pts',(-0.025595910469552,-0.102000707380013,
-0.808171847428544));
#46778=CARTESIAN_POINT('Ctrl Pts',(0.0715358053219139,-0.0770838730453207,
-0.801844186412671));
#46779=CARTESIAN_POINT('Ctrl Pts',(0.103625175378567,0.0179197647919879,
-0.795516525396799));
#46780=CARTESIAN_POINT('Ctrl Pts',(0.0414956507199254,0.0966302535859462,
-0.789188864380927));
#46781=CARTESIAN_POINT('Ctrl Pts',(-0.058362874856174,0.0874818253934899,
-0.782861203365056));
#46782=CARTESIAN_POINT('Ctrl Pts',(-0.10515624968344,-0.00120751413291408,
-0.776533542349183));
#46783=CARTESIAN_POINT('Ctrl Pts',(-0.0563386344921838,-0.0887989481945397,
-0.770205881333312));
#46784=CARTESIAN_POINT('Ctrl Pts',(0.0437036357690681,-0.0956519061880418,
-0.763878220317438));
#46785=CARTESIAN_POINT('Ctrl Pts',(0.104009343583256,-0.0155354879075021,
-0.757550559301568));
#46786=CARTESIAN_POINT('Ctrl Pts',(0.0697468603499374,0.0787062285229874,
-0.751222898285696));
#46787=CARTESIAN_POINT('Ctrl Pts',(-0.0279314102255587,0.101386050617451,
-0.744895237269823));
#46788=CARTESIAN_POINT('Ctrl Pts',(-0.100213664949813,0.0318828526697282,
-0.738567576253952));
#46789=CARTESIAN_POINT('Ctrl Pts',(-0.0813788653223073,-0.0666091226174153,
-0.732239915238079));
#46790=CARTESIAN_POINT('Ctrl Pts',(0.0114478644309889,-0.10453822906947,
-0.725912254222208));
#46791=CARTESIAN_POINT('Ctrl Pts',(0.0938658771088217,-0.0474182670666902,
-0.719584593206335));
#46792=CARTESIAN_POINT('Ctrl Pts',(0.0909384208772093,0.052815703586832,
-0.713256932190464));
#46793=CARTESIAN_POINT('Ctrl Pts',(0.00532722044912209,0.105028166028451,
-0.706929271174591));
#46794=CARTESIAN_POINT('Ctrl Pts',(-0.0851276371333977,0.0617460956911325,
-0.70060161015872));
#46795=CARTESIAN_POINT('Ctrl Pts',(-0.0981820768848795,-0.0376772440019834,
-0.694273949142847));
#46796=CARTESIAN_POINT('Ctrl Pts',(-0.0219666387176374,-0.102843384427304,
-0.687946288126977));
#46797=CARTESIAN_POINT('Ctrl Pts',(0.0742214789734623,-0.0745014563347958,
-0.681618627111103));
#46798=CARTESIAN_POINT('Ctrl Pts',(0.102925361485087,0.0215792701493254,
-0.675290966095233));
#46799=CARTESIAN_POINT('Ctrl Pts',(0.0380466396555165,0.098039523397132,
-0.668963305079359));
#46800=CARTESIAN_POINT('Ctrl Pts',(-0.0614251462548661,0.0853595123262889,
-0.662635644063488));
#46801=CARTESIAN_POINT('Ctrl Pts',(-0.105047478972877,-0.00493174395690157,
-0.656307983047617));
#46802=CARTESIAN_POINT('Ctrl Pts',(-0.0531577190451583,-0.0907389213233747,
-0.649980322031743));
#46803=CARTESIAN_POINT('Ctrl Pts',(0.0470645190716644,-0.0940437450422222,
-0.643652661015872));
#46804=CARTESIAN_POINT('Ctrl Pts',(0.104494386063995,-0.0118413773743694,
-0.637325));
#46805=CARTESIAN_POINT('Ctrl Pts',(0.066915047882731,0.08112750029346,-0.630997338984128));
#46806=CARTESIAN_POINT('Ctrl Pts',(-0.0315053149024559,0.100332995918145,
-0.624669677968256));
#46807=CARTESIAN_POINT('Ctrl Pts',(-0.101280168197851,0.0283129381525223,
-0.618342016952384));
#46808=CARTESIAN_POINT('Ctrl Pts',(-0.0789682726947726,-0.0694500312787372,
-0.612014355936513));
#46809=CARTESIAN_POINT('Ctrl Pts',(0.015143775000857,-0.104067098622653,
-0.60568669492064));
#46810=CARTESIAN_POINT('Ctrl Pts',(0.0954866808281567,-0.0440634624313079,
-0.599359033904768));
#46811=CARTESIAN_POINT('Ctrl Pts',(0.0890104378775313,0.0560039006307925,
-0.593031372888897));
#46812=CARTESIAN_POINT('Ctrl Pts',(0.00160342655319863,0.105150957961885,
-0.586703711873024));
#46813=CARTESIAN_POINT('Ctrl Pts',(-0.0872614648363879,0.0586918366693476,
-0.580376050857153));
#46814=CARTESIAN_POINT('Ctrl Pts',(-0.0967858028367096,-0.0411315366387778,
-0.57404838984128));
#46815=CARTESIAN_POINT('Ctrl Pts',(-0.0183097941583832,-0.103556971638278,
-0.56772072882541));
#46816=CARTESIAN_POINT('Ctrl Pts',(0.0768139891555562,-0.0718255247598207,
-0.561393067809536));
#46817=CARTESIAN_POINT('Ctrl Pts',(0.102096354851012,0.0252116890181875,
-0.555065406793666));
#46818=CARTESIAN_POINT('Ctrl Pts',(0.034549872118425,0.0993257331894107,
-0.548737745777792));
#46819=CARTESIAN_POINT('Ctrl Pts',(-0.064410316292193,0.0831300552878031,
-0.542410084761922));
#46820=CARTESIAN_POINT('Ctrl Pts',(-0.104806851798498,-0.00864978341354531,
-0.536082423746048));
#46821=CARTESIAN_POINT('Ctrl Pts',(-0.0499100795856327,-0.0925649982054197,
-0.529754762730178));
#46822=CARTESIAN_POINT('Ctrl Pts',(0.0503663265979779,-0.0923175394063303,
-0.523427101714305));
#46823=CARTESIAN_POINT('Ctrl Pts',(0.104848266324252,-0.00813240344623186,
-0.517099440698433));
#46824=CARTESIAN_POINT('Ctrl Pts',(0.0639992430914645,0.0834469401520101,
-0.51077177968256));
#46825=CARTESIAN_POINT('Ctrl Pts',(-0.0350396738463096,0.0991540024091705,
-0.50444411866669));
#46826=CARTESIAN_POINT('Ctrl Pts',(-0.102219543737853,0.0247074850002744,
-0.498116457650817));
#46827=CARTESIAN_POINT('Ctrl Pts',(-0.0764585584355753,-0.0722037656841195,
-0.491788796634945));
#46828=CARTESIAN_POINT('Ctrl Pts',(0.0188206769785697,-0.103465342289493,
-0.485461135619074));
#46829=CARTESIAN_POINT('Ctrl Pts',(0.096987628872835,-0.040653348971995,
-0.479133474603201));
#46830=CARTESIAN_POINT('Ctrl Pts',(0.0869707282371049,0.0591218011136432,
-0.472805813587329));
#46831=CARTESIAN_POINT('Ctrl Pts',(-0.00212237997704562,0.10514176353974,
-0.466478152571458));
#46832=CARTESIAN_POINT('Ctrl Pts',(-0.0892857612241227,0.0555639071668154,
-0.460150491555585));
#46833=CARTESIAN_POINT('Ctrl Pts',(-0.0952680424451362,-0.0445342006292383,
-0.453822830539714));
#46834=CARTESIAN_POINT('Ctrl Pts',(-0.0146299669934629,-0.104140573278544,
-0.447495169523841));
#46835=CARTESIAN_POINT('Ctrl Pts',(0.0793100817806202,-0.0690594371897487,
-0.441167508507969));
#46836=CARTESIAN_POINT('Ctrl Pts',(0.101139196024548,0.028812461965643,
-0.434839847492098));
#46837=CARTESIAN_POINT('Ctrl Pts',(0.0310097372949585,0.100487268496617,
-0.428512186476226));
#46838=CARTESIAN_POINT('Ctrl Pts',(-0.0673146379656645,0.0807962527136316,
-0.422184525460353));
#46839=CARTESIAN_POINT('Ctrl Pts',(-0.104434670193454,-0.0123569655902224,
-0.415856864444482));
#46840=CARTESIAN_POINT('Ctrl Pts',(-0.0465997925797717,-0.0942748867330842,
-0.409529203428609));
#46841=CARTESIAN_POINT('Ctrl Pts',(0.0536049138929184,-0.0904754560283965,
-0.403201542412738));
#46842=CARTESIAN_POINT('Ctrl Pts',(0.105070540169988,-0.00441322165775816,
-0.396873881396865));
#46843=CARTESIAN_POINT('Ctrl Pts',(0.0610031059188372,0.0856616367183621,
-0.390546220380995));
#46844=CARTESIAN_POINT('Ctrl Pts',(-0.0385300507005929,0.0978505499730241,
-0.384218559365121));
#46845=CARTESIAN_POINT('Ctrl Pts',(-0.103030612457752,0.0210710188076898,
-0.37789089834925));
#46846=CARTESIAN_POINT('Ctrl Pts',(-0.0738528727589387,-0.0748668693232562,
-0.371563237333377));
#46847=CARTESIAN_POINT('Ctrl Pts',(0.022473955086258,-0.102733715399544,
-0.365235576317507));
#46848=CARTESIAN_POINT('Ctrl Pts',(0.0983668372403937,-0.0371922070914784,
-0.358907915301634));
#46849=CARTESIAN_POINT('Ctrl Pts',(0.084821852216415,0.0621654914208049,
-0.352580254285762));
#46850=CARTESIAN_POINT('Ctrl Pts',(-0.00584552247831859,0.105000594302933,
-0.34625259326989));
#46851=CARTESIAN_POINT('Ctrl Pts',(-0.0911979853829655,0.0523662333866202,
-0.339924932254018));
#46852=CARTESIAN_POINT('Ctrl Pts',(-0.0936307008156065,-0.0478809649212701,
-0.333597271238147));
#46853=CARTESIAN_POINT('Ctrl Pts',(-0.0109317761724884,-0.104593456806476,
-0.327269610222274));
#46854=CARTESIAN_POINT('Ctrl Pts',(0.0817066237324652,-0.0662066656406656,
-0.320941949206403));
#46855=CARTESIAN_POINT('Ctrl Pts',(0.100055086439402,0.0323770692715896,
-0.31461428819053));
#46856=CARTESIAN_POINT('Ctrl Pts',(0.0274306787917429,0.101522671349988,
-0.308286627174658));
#46857=CARTESIAN_POINT('Ctrl Pts',(-0.0701344657466005,0.0783610340121442,
-0.301958966158786));
#46858=CARTESIAN_POINT('Ctrl Pts',(-0.103931401323188,-0.0160486372010826,
-0.295631305142914));
#46859=CARTESIAN_POINT('Ctrl Pts',(-0.0432310131273129,-0.0958664406400886,
-0.289303644127042));
#46860=CARTESIAN_POINT('Ctrl Pts',(0.0567762158548203,-0.0885198071067735,
-0.28297598311117));
#46861=CARTESIAN_POINT('Ctrl Pts',(0.105160928601227,-0.00068850035681389,
-0.276648322095299));
#46862=CARTESIAN_POINT('Ctrl Pts',(0.0579303971411072,0.0877688100869956,
-0.270320661079426));
#46863=CARTESIAN_POINT('Ctrl Pts',(-0.0419720643152929,0.0964242747140277,
-0.263993000063555));
#46864=CARTESIAN_POINT('Ctrl Pts',(-0.103712356297359,0.0174081040973306,
-0.257665339047682));
#46865=CARTESIAN_POINT('Ctrl Pts',(-0.0711544863431584,-0.0774359994463466,
-0.251337678031811));
#46866=CARTESIAN_POINT('Ctrl Pts',(0.0260990236988984,-0.10187313629695,
-0.245010017015938));
#46867=CARTESIAN_POINT('Ctrl Pts',(0.0996225747370502,-0.0336843812437931,
-0.238682356000067));
#46868=CARTESIAN_POINT('Ctrl Pts',(0.0825665071024629,0.0651311510869428,
-0.232354694984194));
#46869=CARTESIAN_POINT('Ctrl Pts',(-0.00956132763119429,0.104727627448239,
-0.226027033968323));
#46870=CARTESIAN_POINT('Ctrl Pts',(-0.0929957370733558,0.049102829075485,
-0.219699372952451));
#46871=CARTESIAN_POINT('Ctrl Pts',(-0.0918758331527737,-0.0511676286286223,
-0.213371711936579));
#46872=CARTESIAN_POINT('Ctrl Pts',(-0.00721986369558417,-0.10491505375876,
-0.207044050920707));
#46873=CARTESIAN_POINT('Ctrl Pts',(0.0840006068522954,-0.0632707909353925,
-0.200716389904835));
#46874=CARTESIAN_POINT('Ctrl Pts',(0.0988453868778612,0.0359010366118765,
-0.194388728888963));
#46875=CARTESIAN_POINT('Ctrl Pts',(0.0238171890747536,0.102430642102243,
-0.188061067873091));
#46876=CARTESIAN_POINT('Ctrl Pts',(-0.0728662601675932,0.0758274558920166,
-0.181733406857219));
#46877=CARTESIAN_POINT('Ctrl Pts',(-0.103297676887683,-0.0197201644329452,
-0.175405745841347));
#46878=CARTESIAN_POINT('Ctrl Pts',(-0.0398079697620071,-0.0973376621877754,
-0.169078084825476));
#46879=CARTESIAN_POINT('Ctrl Pts',(0.0598762518653202,-0.0864530474014625,
-0.162750423809603));
#46880=CARTESIAN_POINT('Ctrl Pts',(0.10511931811198,0.00303708518060201,
-0.156422762793732));
#46881=CARTESIAN_POINT('Ctrl Pts',(0.0547849737420719,0.0897658152687806,
-0.150095101777859));
#46882=CARTESIAN_POINT('Ctrl Pts',(-0.0453613944250523,0.0948769669950499,
-0.143767440761988));
#46883=CARTESIAN_POINT('Ctrl Pts',(-0.104263919187185,0.013723338418848,
-0.137439779746115));
#46884=CARTESIAN_POINT('Ctrl Pts',(-0.0683667868681693,-0.079907930935011,
-0.131112118730244));
#46885=CARTESIAN_POINT('Ctrl Pts',(0.0296913338196458,-0.100884685804011,
-0.124784457714371));
#46886=CARTESIAN_POINT('Ctrl Pts',(0.1007532628379,-0.0301342733122123,
-0.1184567966985));
#46887=CARTESIAN_POINT('Ctrl Pts',(0.0802075282097526,0.0680150553744678,
-0.112129135682628));
#46888=CARTESIAN_POINT('Ctrl Pts',(-0.0132651396461531,0.10432320981077,
-0.105801474666756));
#46889=CARTESIAN_POINT('Ctrl Pts',(-0.0946767439621274,0.0457777825103404,
-0.0994738136508837));
#46890=CARTESIAN_POINT('Ctrl Pts',(-0.0900056721113309,-0.0543900511771936,
-0.0931461526350116));
#46891=CARTESIAN_POINT('Ctrl Pts',(-0.00349883201800313,-0.105104989154426,
-0.0868184916191398));
#46892=CARTESIAN_POINT('Ctrl Pts',(0.0861890440424318,-0.0602554437920826,
-0.0804908306032677));
#46893=CARTESIAN_POINT('Ctrl Pts',(0.0975118199824748,0.0393798374633225,
-0.0741631695873958));
#46894=CARTESIAN_POINT('Ctrl Pts',(0.0201734164905109,0.103210236817675,
-0.0678355085715238));
#46895=CARTESIAN_POINT('Ctrl Pts',(-0.0755058576047149,0.0731983272331764,
-0.0615078475556519));
#46896=CARTESIAN_POINT('Ctrl Pts',(-0.102535685748398,-0.0233662345365656,
-0.0551801865397799));
#46897=CARTESIAN_POINT('Ctrl Pts',(-0.036332316246399,-0.0986880403806901,
-0.048852525523908));
#46898=CARTESIAN_POINT('Ctrl Pts',(0.0628961178483592,-0.0842752375943958,
-0.0425248645080358));
#46899=CARTESIAN_POINT('Ctrl Pts',(0.104955270488262,0.00675405203560971,
-0.0361972034921642));
#46900=CARTESIAN_POINT('Ctrl Pts',(0.0515527328771752,0.0916592724290588,
-0.0298695424762917));
#46901=CARTESIAN_POINT('Ctrl Pts',(-0.0486594283428768,0.0931931710624919,
-0.0235418814604202));
#46902=CARTESIAN_POINT('Ctrl Pts',(-0.104750797766374,0.0100550797783035,
-0.017214220444548));
#46903=CARTESIAN_POINT('Ctrl Pts',(-0.0653591496324117,-0.082349657569037,
-0.0108865594286763));
#46904=CARTESIAN_POINT('Ctrl Pts',(0.000161923519070843,-0.0938452514906264,
-0.00666811875142807));
#46905=CARTESIAN_POINT('Ctrl Pts',(0.0281628763286457,-0.0845144524603643,
-0.0045588984128041));
#46906=CARTESIAN_POINT('Ctrl Pts',(0.0868262223680489,0.042511912851507,
-0.949325));
#46907=CARTESIAN_POINT('Ctrl Pts',(0.0727413643237034,0.0712787909934627,
-0.947215779661376));
#46908=CARTESIAN_POINT('Ctrl Pts',(0.0139929319558079,0.113232831299845,
-0.942997338984128));
#46909=CARTESIAN_POINT('Ctrl Pts',(-0.0874824940475139,0.0734063410867091,
-0.936669677968257));
#46910=CARTESIAN_POINT('Ctrl Pts',(-0.109137103018111,-0.0332549081761753,
-0.930342016952384));
#46911=CARTESIAN_POINT('Ctrl Pts',(-0.0317016779449621,-0.109632733995772,
-0.924014355936513));
#46912=CARTESIAN_POINT('Ctrl Pts',(0.0746310386889739,-0.0863541370772251,
-0.91768669492064));
#46913=CARTESIAN_POINT('Ctrl Pts',(0.113068616874035,0.0154530577601656,
-0.91135903390477));
#46914=CARTESIAN_POINT('Ctrl Pts',(0.0487213583111448,0.103203043698082,
-0.905031372888895));
#46915=CARTESIAN_POINT('Ctrl Pts',(-0.0599354161316844,0.0971215647331329,
-0.898703711873025));
#46916=CARTESIAN_POINT('Ctrl Pts',(-0.114091600011384,0.00273254865035857,
-0.892376050857152));
#46917=CARTESIAN_POINT('Ctrl Pts',(-0.0645154989621486,-0.094139971638436,
-0.88604838984128));
#46918=CARTESIAN_POINT('Ctrl Pts',(0.0437214582003731,-0.105418338569157,
-0.879720728825409));
#46919=CARTESIAN_POINT('Ctrl Pts',(0.112204821450399,-0.0208471375856189,
-0.873393067809536));
#46920=CARTESIAN_POINT('Ctrl Pts',(0.0786688729221479,0.0826787140141801,
-0.867065406793666));
#46921=CARTESIAN_POINT('Ctrl Pts',(-0.0263952350250068,0.111030854533241,
-0.860737745777791));
#46922=CARTESIAN_POINT('Ctrl Pts',(-0.107459939205569,0.0384306098074368,
-0.854410084761922));
#46923=CARTESIAN_POINT('Ctrl Pts',(-0.0908191386177551,-0.069111793762257,
-0.848082423746048));
#46924=CARTESIAN_POINT('Ctrl Pts',(0.00839698509998528,-0.113815841594763,
-0.841754762730177));
#46925=CARTESIAN_POINT('Ctrl Pts',(0.0999783184135565,-0.0550353513528612,
-0.835427101714305));
#46926=CARTESIAN_POINT('Ctrl Pts',(0.100656590362684,0.0537848094857212,
-0.829099440698433));
#46927=CARTESIAN_POINT('Ctrl Pts',(0.00981508290605088,0.113702325715277,
-0.822771779682561));
#46928=CARTESIAN_POINT('Ctrl Pts',(-0.0899505686003668,0.0702385207904819,
-0.816444118666689));
#46929=CARTESIAN_POINT('Ctrl Pts',(-0.107930660076814,-0.0370881023753524,
-0.810116457650817));
#46930=CARTESIAN_POINT('Ctrl Pts',(-0.0277771896498851,-0.110693190487889,
-0.803788796634946));
#46931=CARTESIAN_POINT('Ctrl Pts',(0.0776320746061295,-0.083652947726732,
-0.797461135619073));
#46932=CARTESIAN_POINT('Ctrl Pts',(0.112456095375748,0.0194468841302012,
-0.791133474603202));
#46933=CARTESIAN_POINT('Ctrl Pts',(0.0450319030871707,0.104865067525778,
-0.784805813587328));
#46934=CARTESIAN_POINT('Ctrl Pts',(-0.0633365492241791,0.0949370118231875,
-0.778478152571458));
#46935=CARTESIAN_POINT('Ctrl Pts',(-0.114117647575078,-0.00131041828399773,
-0.772150491555585));
#46936=CARTESIAN_POINT('Ctrl Pts',(-0.0611398034372145,-0.0963663796075638,
-0.765822830539714));
#46937=CARTESIAN_POINT('Ctrl Pts',(0.0474280522504172,-0.103803345527359,
-0.759495169523841));
#46938=CARTESIAN_POINT('Ctrl Pts',(0.112873002330155,-0.0168594195710881,
-0.753167508507969));
#46939=CARTESIAN_POINT('Ctrl Pts',(0.0756906760448665,0.0854135600650306,
-0.746839847492098));
#46940=CARTESIAN_POINT('Ctrl Pts',(-0.0303117203018435,0.110026152779519,
-0.740512186476226));
#46941=CARTESIAN_POINT('Ctrl Pts',(-0.108753856602692,0.0345999040057546,
-0.734184525460354));
#46942=CARTESIAN_POINT('Ctrl Pts',(-0.0883139585223654,-0.0722855408311166,
-0.727856864444481));
#46943=CARTESIAN_POINT('Ctrl Pts',(0.0124234495101874,-0.113446959348449,
-0.72152920342861));
#46944=CARTESIAN_POINT('Ctrl Pts',(0.101865111350743,-0.0514592438017468,
-0.715201542412737));
#46945=CARTESIAN_POINT('Ctrl Pts',(0.0986881777920024,0.0573166489533057,
-0.708873881396867));
#46946=CARTESIAN_POINT('Ctrl Pts',(0.00578120527878995,0.113978648652578,
-0.702546220380993));
#46947=CARTESIAN_POINT('Ctrl Pts',(-0.0923822000359727,0.0670080875690203,
-0.696218559365122));
#46948=CARTESIAN_POINT('Ctrl Pts',(-0.106549136944947,-0.0408880923916753,
-0.68989089834925));
#46949=CARTESIAN_POINT('Ctrl Pts',(-0.0238386319703752,-0.111607680331259,
-0.683563237333378));
#46950=CARTESIAN_POINT('Ctrl Pts',(0.0805466209140446,-0.0808504578989677,
-0.677235576317505));
#46951=CARTESIAN_POINT('Ctrl Pts',(0.111696643460103,0.0234182519178975,
-0.670907915301635));
#46952=CARTESIAN_POINT('Ctrl Pts',(0.041288967880603,0.106394435072978,
-0.664580254285761));
#46953=CARTESIAN_POINT('Ctrl Pts',(-0.0666597868758373,0.0926338355937582,
-0.658252593269891));
#46954=CARTESIAN_POINT('Ctrl Pts',(-0.113999607442876,-0.00535202634649346,
-0.651924932254018));
#46955=CARTESIAN_POINT('Ctrl Pts',(-0.0576878109114013,-0.0984716769197821,
-0.645597271238146));
#46956=CARTESIAN_POINT('Ctrl Pts',(0.0510753494621495,-0.102058137159478,
-0.639269610222274));
#46957=CARTESIAN_POINT('Ctrl Pts',(0.11339938004943,-0.0128504975603422,
-0.632941949206402));
#46958=CARTESIAN_POINT('Ctrl Pts',(0.0726175369960301,0.088041172208085,
-0.62661428819053));
#46959=CARTESIAN_POINT('Ctrl Pts',(-0.0341901925335258,0.108883356936053,
-0.620286627174659));
#46960=CARTESIAN_POINT('Ctrl Pts',(-0.109911247077948,0.0307257619745004,
-0.613958966158786));
#46961=CARTESIAN_POINT('Ctrl Pts',(-0.0856979355970119,-0.0753685512501992,
-0.607631305142914));
#46962=CARTESIAN_POINT('Ctrl Pts',(0.0164343249564961,-0.112935679244284,
-0.601303644127043));
#46963=CARTESIAN_POINT('Ctrl Pts',(0.103624039690126,-0.0478185432802246,
-0.594975983111169));
#46964=CARTESIAN_POINT('Ctrl Pts',(0.0965958924057288,0.0607765436125185,
-0.5886483220953));
#46965=CARTESIAN_POINT('Ctrl Pts',(0.00174007029407456,0.114111904893903,
-0.582320661079425));
#46966=CARTESIAN_POINT('Ctrl Pts',(-0.0946978721765143,0.06369354510768,
-0.575993000063556));
#46967=CARTESIAN_POINT('Ctrl Pts',(-0.105033872657499,-0.0446367592653377,
-0.569665339047682));
#46968=CARTESIAN_POINT('Ctrl Pts',(-0.019870151733527,-0.112382079324197,
-0.563337678031811));
#46969=CARTESIAN_POINT('Ctrl Pts',(0.0833600643773254,-0.0779464838857511,
-0.557010017015939));
#46970=CARTESIAN_POINT('Ctrl Pts',(0.110796989020261,0.0273602249111314,
-0.550682356000067));
#46971=CARTESIAN_POINT('Ctrl Pts',(0.0374942064027922,0.10779025544718,
-0.544354694984195));
#46972=CARTESIAN_POINT('Ctrl Pts',(-0.0698993526010974,0.0902143846018526,
-0.538027033968322));
#46973=CARTESIAN_POINT('Ctrl Pts',(-0.113738474061213,-0.00938691649958287,
-0.531699372952451));
#46974=CARTESIAN_POINT('Ctrl Pts',(-0.054163408163978,-0.100453371766237,
-0.525371711936579));
#46975=CARTESIAN_POINT('Ctrl Pts',(0.0546585364698917,-0.100184824569957,
-0.519044050920707));
#46976=CARTESIAN_POINT('Ctrl Pts',(0.113783417925879,-0.00882544549857192,
-0.512716389904835));
#46977=CARTESIAN_POINT('Ctrl Pts',(0.0694532478114199,0.0905582743408296,
-0.506388728888963));
#46978=CARTESIAN_POINT('Ctrl Pts',(-0.0380257489514535,0.107603889798764,
-0.500061067873091));
#46979=CARTESIAN_POINT('Ctrl Pts',(-0.110930676043295,0.0268130527117103,
-0.493733406857219));
#46980=CARTESIAN_POINT('Ctrl Pts',(-0.0829743439112356,-0.07835695843793,
-0.487405745841347));
#46981=CARTESIAN_POINT('Ctrl Pts',(0.0204245719016267,-0.112282641337737,
-0.481078084825475));
#46982=CARTESIAN_POINT('Ctrl Pts',(0.105252898274439,-0.0441178205261098,
-0.474750423809603));
#46983=CARTESIAN_POINT('Ctrl Pts',(0.0943823590531949,0.0641601510495206,
-0.468422762793731));
#46984=CARTESIAN_POINT('Ctrl Pts',(-0.00230324884131971,0.114101926924651,
-0.46209510177786));
#46985=CARTESIAN_POINT('Ctrl Pts',(-0.0968946787615573,0.0602990539796282,
-0.455767440761987));
#46986=CARTESIAN_POINT('Ctrl Pts',(-0.103386768980919,-0.0483293977081192,
-0.449439779746116));
#46987=CARTESIAN_POINT('Ctrl Pts',(-0.0158767303172275,-0.113015415397978,
-0.443112118730243));
#46988=CARTESIAN_POINT('Ctrl Pts',(0.0860688735956011,-0.074944670798716,
-0.436784457714372));
#46989=CARTESIAN_POINT('Ctrl Pts',(0.109758261279774,0.0312678551228649,
-0.4304567966985));
#46990=CARTESIAN_POINT('Ctrl Pts',(0.0336523818857637,0.109050776597685,
-0.424129135682628));
#46991=CARTESIAN_POINT('Ctrl Pts',(-0.0730511800785477,0.0876816957652797,
-0.417801474666755));
#46992=CARTESIAN_POINT('Ctrl Pts',(-0.113334575202457,-0.0134100241171348,
-0.411473813650884));
#46993=CARTESIAN_POINT('Ctrl Pts',(-0.0505710190568692,-0.102308976706315,
-0.405146152635012));
#46994=CARTESIAN_POINT('Ctrl Pts',(0.0581731156287884,-0.0981857591567285,
-0.39881849161914));
#46995=CARTESIAN_POINT('Ctrl Pts',(0.114024633911322,-0.00478931566432666,
-0.392490830603268));
#46996=CARTESIAN_POINT('Ctrl Pts',(0.066201780333436,0.0929617069756521,
-0.386163169587396));
#46997=CARTESIAN_POINT('Ctrl Pts',(-0.0418135751335435,0.106189357365487,
-0.379835508571524));
#46998=CARTESIAN_POINT('Ctrl Pts',(-0.111810863902936,0.0228666874825079,
-0.373507847555652));
#46999=CARTESIAN_POINT('Ctrl Pts',(-0.0801466021399856,-0.0812470113207761,
-0.36718018653978));
#47000=CARTESIAN_POINT('Ctrl Pts',(0.0243891817545069,-0.111488665327419,
-0.360852525523909));
#47001=CARTESIAN_POINT('Ctrl Pts',(0.106749642546848,-0.0403617207173284,
-0.354524864508036));
#47002=CARTESIAN_POINT('Ctrl Pts',(0.0920503561798531,0.0674632241321569,
-0.348197203492164));
#47003=CARTESIAN_POINT('Ctrl Pts',(-0.00634367691964216,0.113948727269254,
-0.341869542476292));
#47004=CARTESIAN_POINT('Ctrl Pts',(-0.0989698623412332,0.0568288749783143,
-0.335541881460421));
#47005=CARTESIAN_POINT('Ctrl Pts',(-0.101609893373419,-0.0519613726895842,
-0.329214220444548));
#47006=CARTESIAN_POINT('Ctrl Pts',(-0.011863380297197,-0.113506893583903,
-0.322886559428676));
#47007=CARTESIAN_POINT('Ctrl Pts',(0.0886696484490485,-0.0718487865385744,
-0.316558898412804));
#47008=CARTESIAN_POINT('Ctrl Pts',(0.108581764058326,0.0351362376632097,
-0.310231237396933));
#47009=CARTESIAN_POINT('Ctrl Pts',(0.0297683166195517,0.110174416307878,
-0.303903576381061));
#47010=CARTESIAN_POINT('Ctrl Pts',(-0.0761113131081678,0.0850389481360976,
-0.297575915365188));
#47011=CARTESIAN_POINT('Ctrl Pts',(-0.112788417843808,-0.0174162993610626,
-0.291248254349317));
#47012=CARTESIAN_POINT('Ctrl Pts',(-0.0469151527867125,-0.104036162569286,
-0.284920593333444));
#47013=CARTESIAN_POINT('Ctrl Pts',(0.0616146754098945,-0.0960634501633001,
-0.278592932317573));
#47014=CARTESIAN_POINT('Ctrl Pts',(0.114122725229451,-0.000747174241290758,
-0.2722652713017));
#47015=CARTESIAN_POINT('Ctrl Pts',(0.0628672158310556,0.0952484533039511,
-0.265937610285829));
#47016=CARTESIAN_POINT('Ctrl Pts',(-0.0455489165689162,0.104641535169077,
-0.259609949269957));
#47017=CARTESIAN_POINT('Ctrl Pts',(-0.112550705837761,0.0188916197972995,
-0.253282288254085));
#47018=CARTESIAN_POINT('Ctrl Pts',(-0.0772182596882115,-0.0840350822803618,
-0.246954627238213));
#47019=CARTESIAN_POINT('Ctrl Pts',(0.0283231781039216,-0.110554747818607,
-0.240626966222341));
#47020=CARTESIAN_POINT('Ctrl Pts',(0.108112393781527,-0.0365549585415569,
-0.234299305206469));
#47021=CARTESIAN_POINT('Ctrl Pts',(0.0896028109350489,0.0706816168156805,
-0.227971644190597));
#47022=CARTESIAN_POINT('Ctrl Pts',(-0.0103761423619725,0.113652498225165,
-0.221643983174725));
#47023=CARTESIAN_POINT('Ctrl Pts',(-0.10092081812797,0.0532873639012817,
-0.215316322158853));
#47024=CARTESIAN_POINT('Ctrl Pts',(-0.0997054761838474,-0.0555281253246631,
-0.208988661142981));
#47025=CARTESIAN_POINT('Ctrl Pts',(-0.00783513926402908,-0.11385589697431,
-0.202661000127109));
#47026=CARTESIAN_POINT('Ctrl Pts',(0.091159124424086,-0.0686627170852657,
-0.196333339111237));
#47027=CARTESIAN_POINT('Ctrl Pts',(0.107268974103842,0.0389605169068645,
-0.190005678095365));
#47028=CARTESIAN_POINT('Ctrl Pts',(0.0258468859173261,0.111159764174754,
-0.183678017079493));
#47029=CARTESIAN_POINT('Ctrl Pts',(-0.0790759105897333,0.082289458915181,
-0.177350356063621));
#47030=CARTESIAN_POINT('Ctrl Pts',(-0.112100687518616,-0.0214007135254068,
-0.171022695047749));
#47031=CARTESIAN_POINT('Ctrl Pts',(-0.043200398242193,-0.10563276136954,
-0.164695034031877));
#47032=CARTESIAN_POINT('Ctrl Pts',(0.0649788959672199,-0.093820561543907,
-0.158367373016006));
#47033=CARTESIAN_POINT('Ctrl Pts',(0.114077568701317,0.00329590506830352,
-0.152039712000133));
#47034=CARTESIAN_POINT('Ctrl Pts',(0.0594537399795861,0.0974156429310687,
-0.145712050984262));
#47035=CARTESIAN_POINT('Ctrl Pts',(-0.0492270848199282,0.102962366146826,
-0.139384389968389));
#47036=CARTESIAN_POINT('Ctrl Pts',(-0.113149272824185,0.0148928390081436,
-0.133056728952518));
#47037=CARTESIAN_POINT('Ctrl Pts',(-0.0741929929333612,-0.0867176713542623,
-0.126729067936645));
#47038=CARTESIAN_POINT('Ctrl Pts',(0.0322216242882799,-0.109482061741097,
-0.120401406920774));
#47039=CARTESIAN_POINT('Ctrl Pts',(0.109339438931944,-0.0327023110098198,
-0.114073745904902));
#47040=CARTESIAN_POINT('Ctrl Pts',(0.0870428002583105,0.0738112869409917,
-0.10774608488903));
#47041=CARTESIAN_POINT('Ctrl Pts',(-0.0143955926131921,0.113213616184728,
-0.101418423873158));
#47042=CARTESIAN_POINT('Ctrl Pts',(-0.102745080140752,0.0496789574277323,
-0.0950907628572858));
#47043=CARTESIAN_POINT('Ctrl Pts',(-0.0976759403333535,-0.0590251621802268,
-0.0887631018414137));
#47044=CARTESIAN_POINT('Ctrl Pts',(-0.00379700189343816,-0.114062018632413,
-0.0824354408255419));
#47045=CARTESIAN_POINT('Ctrl Pts',(0.0935340598630732,-0.0653904025661319,
-0.0761077798096698));
#47046=CARTESIAN_POINT('Ctrl Pts',(0.105821760862179,0.0427357805811043,
-0.0697801187937979));
#47047=CARTESIAN_POINT('Ctrl Pts',(0.0218925916469987,0.112005795820566,
-0.0634524577779259));
#47048=CARTESIAN_POINT('Ctrl Pts',(-0.0819404540759867,0.0794362763547314,
-0.057124796762054));
#47049=CARTESIAN_POINT('Ctrl Pts',(-0.111273759622746,-0.0253575011093263,
-0.050797135746182));
#47050=CARTESIAN_POINT('Ctrl Pts',(-0.0394285501192212,-0.107098218564676,
-0.0444694747303101));
#47051=CARTESIAN_POINT('Ctrl Pts',(0.0682561144208434,-0.0914571591517854,
-0.0381418137144379));
#47052=CARTESIAN_POINT('Ctrl Pts',(0.113899540966728,0.00732963121282598,
-0.0318141526985663));
#47053=CARTESIAN_POINT('Ctrl Pts',(0.0559460480924329,0.0994704601917223,
-0.0254864916826938));
#47054=CARTESIAN_POINT('Ctrl Pts',(-0.0528061766329012,0.101135077408416,
-0.0191588306668223));
#47055=CARTESIAN_POINT('Ctrl Pts',(-0.113677643113911,0.0109119719839194,
-0.0128311696509501));
#47056=CARTESIAN_POINT('Ctrl Pts',(-0.0709290453588032,-0.0893674815208979,
-0.0065035086350784));
#47057=CARTESIAN_POINT('Ctrl Pts',(0.000175722614101231,-0.101842728020838,
-0.00228506795783016));
#47058=CARTESIAN_POINT('Ctrl Pts',(0.0305629119072609,-0.0917167598683523,
-0.000175847619206193));
#47059=CARTESIAN_POINT('Ctrl Pts',(-0.0966824608565994,-8.60709826375376E-5,
-0.0522235916889671));
#47060=CARTESIAN_POINT('Ctrl Pts',(-0.0967482118542818,-0.00730313201218682,
-0.0517481063747054));
#47061=CARTESIAN_POINT('Ctrl Pts',(-0.0960079295412608,-0.0145068569589153,
-0.0512726210604438));
#47062=CARTESIAN_POINT('Ctrl Pts',(-0.094410673781033,-0.0215153244412058,
-0.0507971357461822));
#47063=CARTESIAN_POINT('Ctrl Pts',(-0.0873253564549061,-0.0526044069277746,
-0.0486879154075581));
#47064=CARTESIAN_POINT('Ctrl Pts',(-0.0633769532870638,-0.0798513127462258,
-0.0465786950689341));
#47065=CARTESIAN_POINT('Ctrl Pts',(-0.0334553076131315,-0.0908679224199693,
-0.0444694747303101));
#47066=CARTESIAN_POINT('Ctrl Pts',(-0.00353366193920001,-0.101884532093712,
-0.0423602543916861));
#47067=CARTESIAN_POINT('Ctrl Pts',(0.0323612262408212,-0.096670845622749,
-0.040251034053062));
#47068=CARTESIAN_POINT('Ctrl Pts',(0.0579159080884793,-0.077599537326499,
-0.0381418137144381));
#47069=CARTESIAN_POINT('Ctrl Pts',(0.0834705899361389,-0.058528229030248,
-0.036032593375814));
#47070=CARTESIAN_POINT('Ctrl Pts',(0.0986850654514341,-0.0255992989087089,
-0.03392337303719));
#47071=CARTESIAN_POINT('Ctrl Pts',(0.0966333877300311,0.00622197098187709,
-0.0318141526985659));
#47072=CARTESIAN_POINT('Ctrl Pts',(0.0945817100086281,0.0380432408724604,
-0.029704932359942));
#47073=CARTESIAN_POINT('Ctrl Pts',(0.0752638790505303,0.0687568505320909,
-0.0275957120213179));
#47074=CARTESIAN_POINT('Ctrl Pts',(0.0474795927839263,0.0843910915646887,
-0.025486491682694));
#47075=CARTESIAN_POINT('Ctrl Pts',(0.0196953065173216,0.100025332597287,
-0.02337727134407));
#47076=CARTESIAN_POINT('Ctrl Pts',(-0.0165554350577898,0.100580205002852,
-0.0212680510054461));
#47077=CARTESIAN_POINT('Ctrl Pts',(-0.0448260502588471,0.0858204569682178,
-0.0191588306668222));
#47078=CARTESIAN_POINT('Ctrl Pts',(-0.0708903387085866,0.0722126055831592,
-0.0172142204445482));
#47079=CARTESIAN_POINT('Ctrl Pts',(-0.090171483783908,0.0455872578200469,
-0.015269610222274));
#47080=CARTESIAN_POINT('Ctrl Pts',(-0.0953893049619544,0.016632511936229,
-0.013325));
#47081=CARTESIAN_POINT('',(-0.060188439738649,0.0430776079607707,-0.949325000000001));
#47082=CARTESIAN_POINT('Ctrl Pts',(-0.060189526236291,0.0430788597277722,
-0.949325000000001));
#47083=CARTESIAN_POINT('Ctrl Pts',(-0.0593167659583275,0.0448108322152602,
-0.949325000000001));
#47084=CARTESIAN_POINT('Ctrl Pts',(-0.058373221122004,0.0465024987601996,
-0.949325000000001));
#47085=CARTESIAN_POINT('Ctrl Pts',(-0.0573600015023254,0.0481490225008083,
-0.949325000000001));
#47086=CARTESIAN_POINT('Ctrl Pts',(-0.0550289716257877,0.0519370423508429,
-0.949325000000001));
#47087=CARTESIAN_POINT('Ctrl Pts',(-0.0523302084036976,0.0554864887030456,
-0.949325000000001));
#47088=CARTESIAN_POINT('Ctrl Pts',(-0.0493207856021755,0.058781745439232,
-0.949325000000001));
#47089=CARTESIAN_POINT('Ctrl Pts',(-0.047250923751369,0.0610482020512428,
-0.949325000000001));
#47090=CARTESIAN_POINT('Ctrl Pts',(-0.0450386139126382,0.0631885855487683,
-0.949325000000001));
#47091=CARTESIAN_POINT('Ctrl Pts',(-0.0427077511546215,0.0651933292177597,
-0.949325));
#47092=CARTESIAN_POINT('Ctrl Pts',(-0.0397757434975351,0.0677151095189643,
-0.949325));
#47093=CARTESIAN_POINT('Ctrl Pts',(-0.0366539499723158,0.0700249987493579,
-0.949325));
#47094=CARTESIAN_POINT('Ctrl Pts',(-0.0333746515884088,0.0721117425950514,
-0.949325));
#47095=CARTESIAN_POINT('Ctrl Pts',(-0.0311123386830825,0.0735513394171613,
-0.949325));
#47096=CARTESIAN_POINT('Ctrl Pts',(-0.0287792691540412,0.0748815931761674,
-0.949325));
#47097=CARTESIAN_POINT('Ctrl Pts',(-0.0263934417288112,0.076095782333911,
-0.949325));
#47098=CARTESIAN_POINT('Ctrl Pts',(-0.0203682371240397,0.0791621139666756,
-0.949325));
#47099=CARTESIAN_POINT('Ctrl Pts',(-0.0139965057979827,0.0814990538506737,
-0.949325));
#47100=CARTESIAN_POINT('Ctrl Pts',(-0.00743271588570414,0.0830440140828357,
-0.949325));
#47101=CARTESIAN_POINT('Ctrl Pts',(-0.00427118281189676,0.0837881638708354,
-0.949325));
#47102=CARTESIAN_POINT('Ctrl Pts',(-0.00106024802673121,0.0843478681521641,
-0.949325));
#47103=CARTESIAN_POINT('Ctrl Pts',(0.00215611887931482,0.0847110161631254,
-0.949325));
#47104=CARTESIAN_POINT('Ctrl Pts',(0.00491111070927283,0.0850220720322127,
-0.949325));
#47105=CARTESIAN_POINT('Ctrl Pts',(0.00767363596591655,0.0851900857508143,
-0.949325));
#47106=CARTESIAN_POINT('Ctrl Pts',(0.0104334171757828,0.0852111838068372,
-0.949325));
#47107=CARTESIAN_POINT('Ctrl Pts',(0.0156467829036102,0.085251039097467,
-0.949325));
#47108=CARTESIAN_POINT('Ctrl Pts',(0.0208502407431678,0.0847678597630326,
-0.949325));
#47109=CARTESIAN_POINT('Ctrl Pts',(0.0259925480469261,0.0838058103808331,
-0.949325));
#47110=CARTESIAN_POINT('Ctrl Pts',(0.0290438237261958,0.0832349619836522,
-0.949325));
#47111=CARTESIAN_POINT('Ctrl Pts',(0.0320762587705588,0.0824937705719952,
-0.949325));
#47112=CARTESIAN_POINT('Ctrl Pts',(0.0350558312760954,0.0815973397057138,
-0.949325));
#47113=CARTESIAN_POINT('Ctrl Pts',(0.040320890222968,0.0800132999335661,
-0.949325));
#47114=CARTESIAN_POINT('Ctrl Pts',(0.0454359562981305,0.077943784060909,
-0.949325));
#47115=CARTESIAN_POINT('Ctrl Pts',(0.0503444084903423,0.0754381748870302,
-0.949325));
#47116=CARTESIAN_POINT('Ctrl Pts',(0.0539991272551031,0.0735725568660456,
-0.949325));
#47117=CARTESIAN_POINT('Ctrl Pts',(0.0575394528428315,0.0714647391106675,
-0.949325));
#47118=CARTESIAN_POINT('Ctrl Pts',(0.0609412351239781,0.0691287510149368,
-0.949325));
#47119=CARTESIAN_POINT('Ctrl Pts',(0.0632536174634446,0.067540848800351,
-0.949325));
#47120=CARTESIAN_POINT('Ctrl Pts',(0.0654949036874784,0.065852008116864,
-0.949325));
#47121=CARTESIAN_POINT('Ctrl Pts',(0.0676532889369962,0.0640719733065252,
-0.949325));
#47122=CARTESIAN_POINT('Ctrl Pts',(0.0734442214483512,0.0592961523742621,
-0.949325));
#47123=CARTESIAN_POINT('Ctrl Pts',(0.0786514181655312,0.053859434543402,
-0.949325));
#47124=CARTESIAN_POINT('Ctrl Pts',(0.0831347399305807,0.0478498241354048,
-0.949325));
#47125=CARTESIAN_POINT('Ctrl Pts',(0.0844267955137165,0.0461179050167157,
-0.949325));
#47126=CARTESIAN_POINT('Ctrl Pts',(0.0856585743201443,0.0443381162764104,
-0.949325));
#47127=CARTESIAN_POINT('Ctrl Pts',(0.0868262223680485,0.0425119128515078,
-0.949325));
#47128=CARTESIAN_POINT('Ctrl Pts',(-0.0601895262362904,0.043078859727773,
-0.949325000000001));
#47129=CARTESIAN_POINT('Ctrl Pts',(-0.0689869256062287,0.0306389221630466,
-0.948007581356588));
#47130=CARTESIAN_POINT('Ctrl Pts',(-0.0737422450059072,0.0152538149691926,
-0.946690162713175));
#47131=CARTESIAN_POINT('Ctrl Pts',(-0.0738572813634733,-6.14771210490517E-5,
-0.945372744069761));
#47132=CARTESIAN_POINT('Origin',(-2.39206768658147E-17,-5.43753587379397E-18,
-0.949325));
#47133=CARTESIAN_POINT('Ctrl Pts',(0.0869479092309518,-0.0426124462865232,
-0.949325));
#47134=CARTESIAN_POINT('Ctrl Pts',(0.0856124747599027,-0.044722461608285,
-0.949325));
#47135=CARTESIAN_POINT('Ctrl Pts',(0.0841919414744527,-0.0467735581943342,
-0.949325));
#47136=CARTESIAN_POINT('Ctrl Pts',(0.0826860413332504,-0.0487597210798102,
-0.949325));
#47137=CARTESIAN_POINT('Ctrl Pts',(0.0795662948336701,-0.0528744193523085,
-0.949325));
#47138=CARTESIAN_POINT('Ctrl Pts',(0.0760804375487611,-0.0567111004573341,
-0.949325));
#47139=CARTESIAN_POINT('Ctrl Pts',(0.0722794809423723,-0.0602429512049958,
-0.949325));
#47140=CARTESIAN_POINT('Ctrl Pts',(0.0700290204710016,-0.0623340801815892,
-0.949325));
#47141=CARTESIAN_POINT('Ctrl Pts',(0.0676685942007772,-0.0643170596610832,
-0.949325));
#47142=CARTESIAN_POINT('Ctrl Pts',(0.0652188324310721,-0.0661784227849254,
-0.949325));
#47143=CARTESIAN_POINT('Ctrl Pts',(0.0606222177764784,-0.0696709946416588,
-0.949325));
#47144=CARTESIAN_POINT('Ctrl Pts',(0.0557025495139305,-0.0727449380364621,
-0.949325));
#47145=CARTESIAN_POINT('Ctrl Pts',(0.0505311108350954,-0.0753559521252754,
-0.949325));
#47146=CARTESIAN_POINT('Ctrl Pts',(0.0478794628880133,-0.0766947459461787,
-0.949325));
#47147=CARTESIAN_POINT('Ctrl Pts',(0.0451679051661795,-0.0779080793618369,
-0.949325));
#47148=CARTESIAN_POINT('Ctrl Pts',(0.0424135767913811,-0.0789879073549741,
-0.949325));
#47149=CARTESIAN_POINT('Ctrl Pts',(0.0359064717582129,-0.0815390026540642,
-0.949325));
#47150=CARTESIAN_POINT('Ctrl Pts',(0.0291478261251087,-0.0833546720972159,
-0.949325));
#47151=CARTESIAN_POINT('Ctrl Pts',(0.0222695016912951,-0.0843425229564047,
-0.949325));
#47152=CARTESIAN_POINT('Ctrl Pts',(0.0187466195598109,-0.0848484720685605,
-0.949325));
#47153=CARTESIAN_POINT('Ctrl Pts',(0.0151868435066227,-0.0851359066764804,
-0.949325));
#47154=CARTESIAN_POINT('Ctrl Pts',(0.0116411143525298,-0.0851885509642709,
-0.949325));
#47155=CARTESIAN_POINT('Ctrl Pts',(0.00899012535258925,-0.0852279108312482,
-0.949325));
#47156=CARTESIAN_POINT('Ctrl Pts',(0.00634411118670679,-0.0851367815144602,
-0.949325));
#47157=CARTESIAN_POINT('Ctrl Pts',(0.00371070448365139,-0.0849098407765668,
-0.949325));
#47158=CARTESIAN_POINT('Ctrl Pts',(-0.00105029165046096,-0.0844995494324574,
-0.949325));
#47159=CARTESIAN_POINT('Ctrl Pts',(-0.00577057451462265,-0.0836458514358007,
-0.949325));
#47160=CARTESIAN_POINT('Ctrl Pts',(-0.0104000956501732,-0.0823745810341941,
-0.949325));
#47161=CARTESIAN_POINT('Ctrl Pts',(-0.0136088438978973,-0.0814934560637918,
-0.949325));
#47162=CARTESIAN_POINT('Ctrl Pts',(-0.0167781026383413,-0.0804091054703374,
-0.949325));
#47163=CARTESIAN_POINT('Ctrl Pts',(-0.0198623067016642,-0.0791405298678325,
-0.949325));
#47164=CARTESIAN_POINT('Ctrl Pts',(-0.0241228446148006,-0.0773881119541069,
-0.949325));
#47165=CARTESIAN_POINT('Ctrl Pts',(-0.0282314604779494,-0.0752828969338322,
-0.949325));
#47166=CARTESIAN_POINT('Ctrl Pts',(-0.0321421958340599,-0.0728495357347055,
-0.949325));
#47167=CARTESIAN_POINT('Ctrl Pts',(-0.0349610431368854,-0.0710955756662388,
-0.949325));
#47168=CARTESIAN_POINT('Ctrl Pts',(-0.0376769507073806,-0.0691709018220058,
-0.949325));
#47169=CARTESIAN_POINT('Ctrl Pts',(-0.0402692415138934,-0.0670826356986748,
-0.949325));
#47170=CARTESIAN_POINT('Ctrl Pts',(-0.0421087437862932,-0.0656007918138791,
-0.949325));
#47171=CARTESIAN_POINT('Ctrl Pts',(-0.0438851409941927,-0.0640366886918159,
-0.949325));
#47172=CARTESIAN_POINT('Ctrl Pts',(-0.0455816439518849,-0.062402390001981,
-0.949325));
#47173=CARTESIAN_POINT('Ctrl Pts',(-0.0499864700882501,-0.0581590719747581,
-0.949325));
#47174=CARTESIAN_POINT('Ctrl Pts',(-0.0538751594869068,-0.0534289751223524,
-0.949325));
#47175=CARTESIAN_POINT('Ctrl Pts',(-0.0571141568373989,-0.0482621911224861,
-0.949325));
#47176=CARTESIAN_POINT('Ctrl Pts',(-0.0581865816518023,-0.0465514804387378,
-0.949325));
#47177=CARTESIAN_POINT('Ctrl Pts',(-0.0591873861521787,-0.0447927885495833,
-0.949325));
#47178=CARTESIAN_POINT('Ctrl Pts',(-0.0601104350279403,-0.0429877377952337,
-0.949325));
#47179=CARTESIAN_POINT('Origin',(0.,0.,-0.949325));
#47180=CARTESIAN_POINT('Origin',(0.,0.,-1.05327725593024));
#47181=CARTESIAN_POINT('Ctrl Pts',(-0.0786356739692304,-0.0562359885162954,
-0.962474152380794));
#47182=CARTESIAN_POINT('Ctrl Pts',(-0.0600038161649918,-0.0822892105612963,
-0.96036493204217));
#47183=CARTESIAN_POINT('Ctrl Pts',(0.004853946138599,-0.113990840317091,
-0.956146491364922));
#47184=CARTESIAN_POINT('Ctrl Pts',(0.0983810235117565,-0.0579900836424825,
-0.949818830349049));
#47185=CARTESIAN_POINT('Ctrl Pts',(0.10216681566528,0.0507813110782263,
-0.943491169333179));
#47186=CARTESIAN_POINT('Ctrl Pts',(0.0132059581691852,0.113357553994674,
-0.937163508317305));
#47187=CARTESIAN_POINT('Ctrl Pts',(-0.0878384118263931,0.0728782692965182,
-0.930835847301434));
#47188=CARTESIAN_POINT('Ctrl Pts',(-0.10897753085853,-0.0338704598317053,
-0.924508186285562));
#47189=CARTESIAN_POINT('Ctrl Pts',(-0.0310523850839464,-0.109819800841145,
-0.918180525269691));
#47190=CARTESIAN_POINT('Ctrl Pts',(0.075117597679381,-0.0859197258996397,
-0.911852864253818));
#47191=CARTESIAN_POINT('Ctrl Pts',(0.112982694264295,0.0161019074255883,
-0.905525203237947));
#47192=CARTESIAN_POINT('Ctrl Pts',(0.0481238767758512,0.103482736629349,
-0.899197542222073));
#47193=CARTESIAN_POINT('Ctrl Pts',(-0.0604921422302409,0.0967744449238958,
-0.892869881206203));
#47194=CARTESIAN_POINT('Ctrl Pts',(-0.114106160426482,0.00207599406145328,
-0.88654222019033));
#47195=CARTESIAN_POINT('Ctrl Pts',(-0.0639721344284186,-0.094509934905488,
-0.880214559174458));
#47196=CARTESIAN_POINT('Ctrl Pts',(0.0443273765905862,-0.105164838429805,
-0.873886898158588));
#47197=CARTESIAN_POINT('Ctrl Pts',(0.112323076495157,-0.0202009223948133,
-0.867559237142713));
#47198=CARTESIAN_POINT('Ctrl Pts',(0.0781915744196983,0.0831302239521522,
-0.861231576126844));
#47199=CARTESIAN_POINT('Ctrl Pts',(-0.0270339192117008,0.110877061822789,
-0.85490391511097));
#47200=CARTESIAN_POINT('Ctrl Pts',(-0.107679402325512,0.0378113850182401,
-0.848576254095099));
#47201=CARTESIAN_POINT('Ctrl Pts',(-0.0904197845472554,-0.0696334542227982,
-0.842248593079227));
#47202=CARTESIAN_POINT('Ctrl Pts',(0.00905202397369058,-0.113765618960802,
-0.835920932063354));
#47203=CARTESIAN_POINT('Ctrl Pts',(0.100293477560122,-0.0544589150043569,
-0.829593271047484));
#47204=CARTESIAN_POINT('Ctrl Pts',(0.100345310375543,0.0543633505043467,
-0.823265610031609));
#47205=CARTESIAN_POINT('Ctrl Pts',(0.00916039240033352,0.113756944255607,
-0.81693794901574));
#47206=CARTESIAN_POINT('Ctrl Pts',(-0.090353408994793,0.06971955697025,
-0.810610287999865));
#47207=CARTESIAN_POINT('Ctrl Pts',(-0.107715375494224,-0.0377087926315068,
-0.804282626983996));
#47208=CARTESIAN_POINT('Ctrl Pts',(-0.0271395234400288,-0.110851258090984,
-0.797954965968122));
#47209=CARTESIAN_POINT('Ctrl Pts',(0.0781123388944825,-0.0832046733305623,
-0.791627304952251));
#47210=CARTESIAN_POINT('Ctrl Pts',(0.112342287909493,0.0200939170266501,
-0.785299643936378));
#47211=CARTESIAN_POINT('Ctrl Pts',(0.0444275008731675,0.105122558564952,
-0.778971982920508));
#47212=CARTESIAN_POINT('Ctrl Pts',(-0.0638820069123982,0.0945708430006401,
-0.772644321904634));
#47213=CARTESIAN_POINT('Ctrl Pts',(-0.114108215395601,-0.00196731608905759,
-0.766316660888764));
#47214=CARTESIAN_POINT('Ctrl Pts',(-0.0605840574034091,-0.0967167366163604,
-0.759988999872891));
#47215=CARTESIAN_POINT('Ctrl Pts',(0.0480248123783114,-0.103528607395316,
-0.753661338857019));
#47216=CARTESIAN_POINT('Ctrl Pts',(0.11296818562502,-0.0162093858558479,
-0.747333677841147));
#47217=CARTESIAN_POINT('Ctrl Pts',(0.0751977392068195,0.0858478606104231,
-0.741006016825276));
#47218=CARTESIAN_POINT('Ctrl Pts',(-0.0309445853761717,0.109849842007643,
-0.734678355809402));
#47219=CARTESIAN_POINT('Ctrl Pts',(-0.108951231366766,0.0339732885790987,
-0.728350694793533));
#47220=CARTESIAN_POINT('Ctrl Pts',(-0.0878963843456035,-0.0727927247201165,
-0.722023033777658));
#47221=CARTESIAN_POINT('Ctrl Pts',(0.0130763025601953,-0.113373565986802,
-0.715695372761788));
#47222=CARTESIAN_POINT('Ctrl Pts',(0.10215965110392,-0.0508720044772741,
-0.709367711745915));
#47223=CARTESIAN_POINT('Ctrl Pts',(0.0983566005041366,0.0578837998966845,
-0.703040050730044));
#47224=CARTESIAN_POINT('Ctrl Pts',(0.00512499025186194,0.114010041786363,
-0.696712389714171));
#47225=CARTESIAN_POINT('Ctrl Pts',(-0.0927664038289317,0.0664751793819131,
-0.6903847286983));
#47226=CARTESIAN_POINT('Ctrl Pts',(-0.106312000718267,-0.0415007669385643,
-0.684057067682427));
#47227=CARTESIAN_POINT('Ctrl Pts',(-0.0231957665837685,-0.11174306048163,
-0.677729406666556));
#47228=CARTESIAN_POINT('Ctrl Pts',(0.0810107043522212,-0.0803854522508077,
-0.671401745650683));
#47229=CARTESIAN_POINT('Ctrl Pts',(0.111559987366709,0.0240608472824536,
-0.665074084634812));
#47230=CARTESIAN_POINT('Ctrl Pts',(0.0406758237805722,0.106630354557141,
-0.658746423618939));
#47231=CARTESIAN_POINT('Ctrl Pts',(-0.067191931295414,0.0922485746339869,
-0.652418762603068));
#47232=CARTESIAN_POINT('Ctrl Pts',(-0.113966911659595,-0.00600817775902438,
-0.646091101587196));
#47233=CARTESIAN_POINT('Ctrl Pts',(-0.0571200028417465,-0.0988021276520335,
-0.639763440571324));
#47234=CARTESIAN_POINT('Ctrl Pts',(0.0516620029121628,-0.101762432205179,
-0.633435779555452));
#47235=CARTESIAN_POINT('Ctrl Pts',(0.113471477229269,-0.0121975000970476,
-0.62710811853958));
#47236=CARTESIAN_POINT('Ctrl Pts',(0.0721095251424329,0.088457738705795,
-0.620780457523708));
#47237=CARTESIAN_POINT('Ctrl Pts',(-0.0348164148990489,0.10868473861029,
-0.614452796507836));
#47238=CARTESIAN_POINT('Ctrl Pts',(-0.110086301145192,0.0300925481370394,
-0.608125135491964));
#47239=CARTESIAN_POINT('Ctrl Pts',(-0.0852626573341289,-0.0758606249482087,
-0.601797474476093));
#47240=CARTESIAN_POINT('Ctrl Pts',(0.0170841684337436,-0.112839205696147,
-0.59546981346022));
#47241=CARTESIAN_POINT('Ctrl Pts',(0.103897592599086,-0.0472212389219527,
-0.589142152444348));
#47242=CARTESIAN_POINT('Ctrl Pts',(0.0962444328252329,0.0613315930280561,
-0.582814491428477));
#47243=CARTESIAN_POINT('Ctrl Pts',(0.00108315506015306,0.114120032984247,
-0.576486830412604));
#47244=CARTESIAN_POINT('Ctrl Pts',(-0.0950629574431477,0.0631473615867847,
-0.570159169396732));
#47245=CARTESIAN_POINT('Ctrl Pts',(-0.104775182267608,-0.0452406491332671,
-0.563831508380861));
#47246=CARTESIAN_POINT('Ctrl Pts',(-0.0192228941921356,-0.112494602057556,
-0.557503847364987));
#47247=CARTESIAN_POINT('Ctrl Pts',(0.0838073844924436,-0.0774653306824775,
-0.551176186349117));
#47248=CARTESIAN_POINT('Ctrl Pts',(0.110637655806019,0.0279975761622086,
-0.544848525333244));
#47249=CARTESIAN_POINT('Ctrl Pts',(0.0368730900537828,0.108004307243255,
-0.538520864317373));
#47250=CARTESIAN_POINT('Ctrl Pts',(-0.070417515807047,0.0898105150902397,
-0.5321932033015));
#47251=CARTESIAN_POINT('Ctrl Pts',(-0.113682555710397,-0.0100414979142685,
-0.525865542285629));
#47252=CARTESIAN_POINT('Ctrl Pts',(-0.0535842507778536,-0.100763501436711,
-0.519537881269756));
#47253=CARTESIAN_POINT('Ctrl Pts',(0.055234346870785,-0.0998685239650997,
-0.513210220253885));
#47254=CARTESIAN_POINT('Ctrl Pts',(0.113832338493163,-0.00817030393485694,
-0.506882559238013));
#47255=CARTESIAN_POINT('Ctrl Pts',(0.0689307986032583,0.0909565839130236,
-0.50055489822214));
#47256=CARTESIAN_POINT('Ctrl Pts',(-0.0386445425688116,0.107383213226543,
-0.494227237206269));
#47257=CARTESIAN_POINT('Ctrl Pts',(-0.111083189684309,0.0261740352786816,
-0.487899576190397));
#47258=CARTESIAN_POINT('Ctrl Pts',(-0.0825219079271646,-0.078833304289941,
-0.481571915174525));
#47259=CARTESIAN_POINT('Ctrl Pts',(0.0210705901172056,-0.112163208697516,
-0.475244254158653));
#47260=CARTESIAN_POINT('Ctrl Pts',(0.105505120973288,-0.0435112008754263,
-0.468916593142781));
#47261=CARTESIAN_POINT('Ctrl Pts',(0.09401145833506,0.064702402234578,-0.46258893212691));
#47262=CARTESIAN_POINT('Ctrl Pts',(-0.00296003971678002,0.114086779769108,
-0.456261271111036));
#47263=CARTESIAN_POINT('Ctrl Pts',(-0.0972401872438056,0.0597402806990355,
-0.449933610095166));
#47264=CARTESIAN_POINT('Ctrl Pts',(-0.103106849138143,-0.0489237448895124,
-0.443605949079292));
#47265=CARTESIAN_POINT('Ctrl Pts',(-0.0152258930640914,-0.113104939474856,
-0.437278288063422));
#47266=CARTESIAN_POINT('Ctrl Pts',(0.0864988689077382,-0.0744479739878243,
-0.430950627047549));
#47267=CARTESIAN_POINT('Ctrl Pts',(0.109576450941058,0.0318991622518809,
-0.424622966031678));
#47268=CARTESIAN_POINT('Ctrl Pts',(0.0330240729181738,0.10924269202608,
-0.418295305015805));
#47269=CARTESIAN_POINT('Ctrl Pts',(-0.0735547116681115,0.0872597246421901,
-0.411967643999934));
#47270=CARTESIAN_POINT('Ctrl Pts',(-0.113255504473285,-0.0140622138979488,
-0.405639982984062));
#47271=CARTESIAN_POINT('Ctrl Pts',(-0.0499812393174355,-0.102598396037673,
-0.399312321968189));
#47272=CARTESIAN_POINT('Ctrl Pts',(0.0587373602185643,-0.0978492599244596,
-0.392984660952318));
#47273=CARTESIAN_POINT('Ctrl Pts',(0.114050316460549,-0.00413285233932352,
-0.386656999936446));
#47274=CARTESIAN_POINT('Ctrl Pts',(0.0656655495532949,0.093341259660847,
-0.380329338920574));
#47275=CARTESIAN_POINT('Ctrl Pts',(-0.0424241632878486,0.105946899541873,
-0.374001677904702));
#47276=CARTESIAN_POINT('Ctrl Pts',(-0.111940645681331,0.0222226685538999,
-0.36767401688883));
#47277=CARTESIAN_POINT('Ctrl Pts',(-0.0796775763361311,-0.0817070314135196,
-0.361346355872957));
#47278=CARTESIAN_POINT('Ctrl Pts',(0.0250305638209899,-0.111346423507957,
-0.355018694857086));
#47279=CARTESIAN_POINT('Ctrl Pts',(0.10698021844356,-0.0397465472082552,
-0.348691033841214));
#47280=CARTESIAN_POINT('Ctrl Pts',(0.0916604798817394,0.0679919964485462,
-0.342363372825342));
#47281=CARTESIAN_POINT('Ctrl Pts',(-0.00699951902728272,0.113910323880659,
-0.33603571180947));
#47282=CARTESIAN_POINT('Ctrl Pts',(-0.09929536035398,0.0562582133148854,
-0.329708050793598));
#47283=CARTESIAN_POINT('Ctrl Pts',(-0.10130909543547,-0.0525454311549234,
-0.323380389777726));
#47284=CARTESIAN_POINT('Ctrl Pts',(-0.0112097802686418,-0.113573306632935,
-0.317052728761854));
#47285=CARTESIAN_POINT('Ctrl Pts',(0.0890817792245178,-0.0713371695780267,
-0.310725067745982));
#47286=CARTESIAN_POINT('Ctrl Pts',(0.108377704804983,0.035760708248213,
-0.30439740673011));
#47287=CARTESIAN_POINT('Ctrl Pts',(0.0291336036920155,0.110343954474753,
-0.298069745714238));
#47288=CARTESIAN_POINT('Ctrl Pts',(-0.0765995810443127,0.0845994050631894,
-0.291742084698366));
#47289=CARTESIAN_POINT('Ctrl Pts',(-0.112686293986516,-0.0180652788739757,
-0.285414423682494));
#47290=CARTESIAN_POINT('Ctrl Pts',(-0.0463154909903957,-0.10430450827998,
-0.279086762666623));
#47291=CARTESIAN_POINT('Ctrl Pts',(0.0621666459440579,-0.0957071746802496,
-0.27275910165075));
#47292=CARTESIAN_POINT('Ctrl Pts',(0.114125137523673,-9.02131532161566E-5,
-0.266431440634879));
#47293=CARTESIAN_POINT('Ctrl Pts',(0.06231787656026,0.095608772684466,-0.260103779619006));
#47294=CARTESIAN_POINT('Ctrl Pts',(-0.0461505328448423,0.104377600429143,
-0.253776118603135));
#47295=CARTESIAN_POINT('Ctrl Pts',(-0.112657592850385,0.0182434077510212,
-0.247448457587262));
#47296=CARTESIAN_POINT('Ctrl Pts',(-0.0767332327896328,-0.0844781991928046,
-0.241120796571391));
#47297=CARTESIAN_POINT('Ctrl Pts',(0.0289591189531694,-0.110389875363005,
-0.234793135555518));
#47298=CARTESIAN_POINT('Ctrl Pts',(0.108321033455404,-0.0359320033450135,
-0.228465474539647));
#47299=CARTESIAN_POINT('Ctrl Pts',(0.0891944484327669,0.0711962465440421,
-0.222137813523774));
#47300=CARTESIAN_POINT('Ctrl Pts',(-0.0110302124830365,0.113590886807688,
-0.215810152507903));
#47301=CARTESIAN_POINT('Ctrl Pts',(-0.101225897103969,0.0527055301544334,
-0.209482491492031));
#47302=CARTESIAN_POINT('Ctrl Pts',(-0.099384177713727,-0.0561011619592128,
-0.203154830476159));
#47303=CARTESIAN_POINT('Ctrl Pts',(-0.00717959686625945,-0.113899115632717,
-0.196827169460287));
#47304=CARTESIAN_POINT('Ctrl Pts',(0.0915528733567521,-0.0681368221619972,
-0.190499508444415));
#47305=CARTESIAN_POINT('Ctrl Pts',(0.107042922065464,0.0395773671092362,
-0.184171847428543));
#47306=CARTESIAN_POINT('Ctrl Pts',(0.025206565740586,0.111306712270516,
-0.177844186412671));
#47307=CARTESIAN_POINT('Ctrl Pts',(-0.0795483020206782,0.0818328956179269,
-0.171516525396799));
#47308=CARTESIAN_POINT('Ctrl Pts',(-0.111975638670248,-0.0220456681799031,
-0.165188864380927));
#47309=CARTESIAN_POINT('Ctrl Pts',(-0.0425916071836757,-0.105879696603329,
-0.158861203365055));
#47310=CARTESIAN_POINT('Ctrl Pts',(0.0655178997864847,-0.0934449570602429,
-0.152533542349183));
#47311=CARTESIAN_POINT('Ctrl Pts',(0.11405670737362,0.00395253939170301,
-0.146205881333311));
#47312=CARTESIAN_POINT('Ctrl Pts',(0.0588919823963425,0.0977562765503247,
-0.139878220317439));
#47313=CARTESIAN_POINT('Ctrl Pts',(-0.0498189752833788,0.10267728612641,
-0.133550559301567));
#47314=CARTESIAN_POINT('Ctrl Pts',(-0.113233128592107,0.0142412468351748,
-0.127222898285695));
#47315=CARTESIAN_POINT('Ctrl Pts',(-0.0736925781380903,-0.0871433276491138,
-0.120895237269823));
#47316=CARTESIAN_POINT('Ctrl Pts',(0.0328513340057859,-0.109294767937933,
-0.114567576253951));
#47317=CARTESIAN_POINT('Ctrl Pts',(0.109525864708063,-0.0320723516270534,
-0.10823991523808));
#47318=CARTESIAN_POINT('Ctrl Pts',(0.0866164940802407,0.0743111196969755,
-0.101912254222207));
#47319=CARTESIAN_POINT('Ctrl Pts',(-0.0150471265603088,0.113128890038952,
-0.0955845932063355));
#47320=CARTESIAN_POINT('Ctrl Pts',(-0.103029249389535,0.0490866516361247,
-0.0892569321904636));
#47321=CARTESIAN_POINT('Ctrl Pts',(-0.0973347490159742,-0.0595864002598666,
-0.0829292711745916));
#47322=CARTESIAN_POINT('Ctrl Pts',(-0.0031399522792829,-0.114082097613606,
-0.0766016101587196));
#47323=CARTESIAN_POINT('Ctrl Pts',(0.0939081973359286,-0.0648506831041721,
-0.0702739491428478));
#47324=CARTESIAN_POINT('Ctrl Pts',(0.105575394673151,0.0433438440773199,
-0.0639462881269755));
#47325=CARTESIAN_POINT('Ctrl Pts',(0.0212448220591022,0.112130713062334,
-0.057618627111104));
#47326=CARTESIAN_POINT('Ctrl Pts',(-0.0823913570012463,0.0789618551753083,
-0.0512909660952317));
#47327=CARTESIAN_POINT('Ctrl Pts',(-0.111135465058482,-0.0259949443945141,
-0.0449633050793599));
#47328=CARTESIAN_POINT('Ctrl Pts',(-0.0387933145627912,-0.107328519621086,
-0.0386356440634877));
#47329=CARTESIAN_POINT('Ctrl Pts',(0.0687470363868423,-0.0910529777988239,
-0.0323079830476161));
#47330=CARTESIAN_POINT('Ctrl Pts',(0.113921978618372,0.0079660765599,-0.0259803220317439));
#47331=CARTESIAN_POINT('Ctrl Pts',(0.0552360881026894,0.0998320942404049,
-0.0196526610158721));
#47332=CARTESIAN_POINT('Ctrl Pts',(-0.0169523777846908,0.10042205443332,
-0.015434220338624));
#47333=CARTESIAN_POINT('Ctrl Pts',(-0.0452560140322625,0.0854280329804665,
-0.013325));
#47334=CARTESIAN_POINT('Ctrl Pts',(-0.0724605943221337,-0.0518199049426082,
-0.958091101587196));
#47335=CARTESIAN_POINT('Ctrl Pts',(-0.0552918537025914,-0.0758272270407944,
-0.955981881248572));
#47336=CARTESIAN_POINT('Ctrl Pts',(0.00447277684868737,-0.105039400309431,
-0.951763440571323));
#47337=CARTESIAN_POINT('Ctrl Pts',(0.0906553867201687,-0.0534362549899266,
-0.945435779555453));
#47338=CARTESIAN_POINT('Ctrl Pts',(0.0941438892734977,0.0467935708496025,
-0.939108118539579));
#47339=CARTESIAN_POINT('Ctrl Pts',(0.0121689244744929,0.104455844513668,
-0.932780457523709));
#47340=CARTESIAN_POINT('Ctrl Pts',(-0.0809406622208554,0.0671553054719232,
-0.926452796507834));
#47341=CARTESIAN_POINT('Ctrl Pts',(-0.100419774577854,-0.0312106900785216,
-0.920125135491966));
#47342=CARTESIAN_POINT('Ctrl Pts',(-0.0286139122961286,-0.101195903024898,
-0.91379747447609));
#47343=CARTESIAN_POINT('Ctrl Pts',(0.0692187845179366,-0.0791726463121411,
-0.907469813460221));
#47344=CARTESIAN_POINT('Ctrl Pts',(0.10411042166066,0.0148374614584551,
-0.901142152444347));
#47345=CARTESIAN_POINT('Ctrl Pts',(0.0443448187857815,0.095356473973601,
-0.894814491428477));
#47346=CARTESIAN_POINT('Ctrl Pts',(-0.0557418326386755,0.0891749690747734,
-0.888486830412603));
#47347=CARTESIAN_POINT('Ctrl Pts',(-0.105145664594354,0.0019129709953397,
-0.882159169396733));
#47348=CARTESIAN_POINT('Ctrl Pts',(-0.0589485490078265,-0.0870882858494668,
-0.87583150838086));
#47349=CARTESIAN_POINT('Ctrl Pts',(0.0408464490779558,-0.0969064841664184,
-0.869503847364989));
#47350=CARTESIAN_POINT('Ctrl Pts',(0.103502602166471,-0.0186145901560687,
-0.863176186349116));
#47351=CARTESIAN_POINT('Ctrl Pts',(0.0720513688946276,0.0766021975733563,
-0.856848525333245));
#47352=CARTESIAN_POINT('Ctrl Pts',(-0.0249110073591139,0.102170139719473,
-0.850520864317372));
#47353=CARTESIAN_POINT('Ctrl Pts',(-0.0992235851098809,0.0348421434225487,
-0.844193203301501));
#47354=CARTESIAN_POINT('Ctrl Pts',(-0.0833193256452169,-0.0641652983054661,
-0.837865542285629));
#47355=CARTESIAN_POINT('Ctrl Pts',(0.00834118923185522,-0.104831865071198,
-0.831537881269756));
#47356=CARTESIAN_POINT('Ctrl Pts',(0.0924176601256532,-0.0501823809496229,
-0.825210220253886));
#47357=CARTESIAN_POINT('Ctrl Pts',(0.0924654226286142,0.0500943209112546,
-0.818882559238012));
#47358=CARTESIAN_POINT('Ctrl Pts',(0.00844104773377868,0.104823871570765,
-0.812554898222141));
#47359=CARTESIAN_POINT('Ctrl Pts',(-0.083258162413097,0.0642446396010664,
-0.806227237206269));
#47360=CARTESIAN_POINT('Ctrl Pts',(-0.0992567333879196,-0.0347476073813297,
-0.799899576190397));
#47361=CARTESIAN_POINT('Ctrl Pts',(-0.0250083187288948,-0.102146362295717,
-0.793571915174525));
#47362=CARTESIAN_POINT('Ctrl Pts',(0.0719783555540055,-0.0766708006123362,
-0.787244254158653));
#47363=CARTESIAN_POINT('Ctrl Pts',(0.103520304952373,0.0185159876747599,
-0.780916593142782));
#47364=CARTESIAN_POINT('Ctrl Pts',(0.0409387108295975,0.0968675244426629,
-0.774588932126909));
#47365=CARTESIAN_POINT('Ctrl Pts',(-0.058865498999529,0.0871444109711961,
-0.768261271111037));
#47366=CARTESIAN_POINT('Ctrl Pts',(-0.105147558191447,-0.00181282725558375,
-0.761933610095165));
#47367=CARTESIAN_POINT('Ctrl Pts',(-0.0558265299234932,-0.089121792468657,
-0.755605949079293));
#47368=CARTESIAN_POINT('Ctrl Pts',(0.0442535336888328,-0.0953987426132174,
-0.749278288063421));
#47369=CARTESIAN_POINT('Ctrl Pts',(0.104097052351647,-0.0149364998533759,
-0.74295062704755));
#47370=CARTESIAN_POINT('Ctrl Pts',(0.069292632714499,0.0791064244397399,
-0.736622966031677));
#47371=CARTESIAN_POINT('Ctrl Pts',(-0.0285145778528813,0.101223585127291,
-0.730295305015805));
#47372=CARTESIAN_POINT('Ctrl Pts',(-0.100395540325034,0.0313054439195385,
-0.723967643999934));
#47373=CARTESIAN_POINT('Ctrl Pts',(-0.0809940822907079,-0.0670764785154766,
-0.717639982984061));
#47374=CARTESIAN_POINT('Ctrl Pts',(0.012049450423971,-0.104470599120672,
-0.71131232196819));
#47375=CARTESIAN_POINT('Ctrl Pts',(0.094137287328756,-0.0468771423034273,
-0.704984660952317));
#47376=CARTESIAN_POINT('Ctrl Pts',(0.090632881595485,0.0533383174636288,
-0.698656999936446));
#47377=CARTESIAN_POINT('Ctrl Pts',(0.00472253648757906,0.105057093931231,
-0.692329338920574));
#47378=CARTESIAN_POINT('Ctrl Pts',(-0.0854816702811205,0.0612550355652661,
-0.686001677904702));
#47379=CARTESIAN_POINT('Ctrl Pts',(-0.0979635624237802,-0.0382418066178133,
-0.67967401688883));
#47380=CARTESIAN_POINT('Ctrl Pts',(-0.0213742560796902,-0.102968133484064,
-0.673346355872957));
#47381=CARTESIAN_POINT('Ctrl Pts',(0.0746491190005382,-0.0740729665167775,
-0.667018694857086));
#47382=CARTESIAN_POINT('Ctrl Pts',(0.102799436682193,0.0221714039694361,
-0.660691033841214));
#47383=CARTESIAN_POINT('Ctrl Pts',(0.0374816443594792,0.0982569166637223,
-0.654363372825342));
#47384=CARTESIAN_POINT('Ctrl Pts',(-0.0619155025901194,0.0850045050286458,
-0.64803571180947));
#47385=CARTESIAN_POINT('Ctrl Pts',(-0.105017350714686,-0.00553636929954055,
-0.641708050793597));
#47386=CARTESIAN_POINT('Ctrl Pts',(-0.0526344996447092,-0.0910434225153208,
-0.635380389777726));
#47387=CARTESIAN_POINT('Ctrl Pts',(0.0476051039678494,-0.0937712611217446,
-0.629052728761854));
#47388=CARTESIAN_POINT('Ctrl Pts',(0.104560821617178,-0.0112396583085458,
-0.622725067745982));
#47389=CARTESIAN_POINT('Ctrl Pts',(0.0664469290382389,0.0815113547767389,
-0.61639740673011));
#47390=CARTESIAN_POINT('Ctrl Pts',(-0.0320823614577048,0.10014997463529,
-0.610069745714238));
#47391=CARTESIAN_POINT('Ctrl Pts',(-0.10144147566952,0.0277294491496382,
-0.603742084698366));
#47392=CARTESIAN_POINT('Ctrl Pts',(-0.0785671758384483,-0.0699034635545515,
-0.597414423682494));
#47393=CARTESIAN_POINT('Ctrl Pts',(0.015742587755945,-0.103978200921628,
-0.591086762666622));
#47394=CARTESIAN_POINT('Ctrl Pts',(0.0957387522527569,-0.0435130630183326,
-0.584759101650751));
#47395=CARTESIAN_POINT('Ctrl Pts',(0.0886865776141488,0.0565153632850548,
-0.578431440634878));
#47396=CARTESIAN_POINT('Ctrl Pts',(0.000998097370316146,0.105158447771881,
-0.572103779619006));
#47397=CARTESIAN_POINT('Ctrl Pts',(-0.087597880791936,0.0581885436912965,
-0.565776118603135));
#47398=CARTESIAN_POINT('Ctrl Pts',(-0.0965474268115447,-0.0416880044163974,
-0.559448457587262));
#47399=CARTESIAN_POINT('Ctrl Pts',(-0.0177133642715224,-0.103660658218711,
-0.553120796571391));
#47400=CARTESIAN_POINT('Ctrl Pts',(0.0772261822449981,-0.0713821554172644,
-0.546793135555518));
#47401=CARTESIAN_POINT('Ctrl Pts',(0.10194953370971,0.0257989905330583,
-0.540465474539647));
#47402=CARTESIAN_POINT('Ctrl Pts',(0.0339775306158899,0.0995229759874494,
-0.534137813523775));
#47403=CARTESIAN_POINT('Ctrl Pts',(-0.0648877893265522,0.0827579007253394,
-0.527810152507903));
#47404=CARTESIAN_POINT('Ctrl Pts',(-0.104755324587893,-0.00925296204667948,
-0.521482491492031));
#47405=CARTESIAN_POINT('Ctrl Pts',(-0.049376402104582,-0.0928507741020977,
-0.515154830476159));
#47406=CARTESIAN_POINT('Ctrl Pts',(0.0508969199248936,-0.0920260771646337,
-0.508827169460287));
#47407=CARTESIAN_POINT('Ctrl Pts',(0.104893345271262,-0.00752870865129053,
-0.502499508444414));
#47408=CARTESIAN_POINT('Ctrl Pts',(0.0635178206248455,0.0838139713843825,
-0.496171847428543));
#47409=CARTESIAN_POINT('Ctrl Pts',(-0.0356098750159982,0.098950655063507,
-0.489844186412671));
#47410=CARTESIAN_POINT('Ctrl Pts',(-0.102360080831417,0.0241186481449105,
-0.483516525396799));
#47411=CARTESIAN_POINT('Ctrl Pts',(-0.0760416512146703,-0.0726427051857141,
-0.477188864380927));
#47412=CARTESIAN_POINT('Ctrl Pts',(0.0194159648610402,-0.103355288421382,
-0.470861203365055));
#47413=CARTESIAN_POINT('Ctrl Pts',(0.097220045099944,-0.0400943657752184,
-0.464533542349183));
#47414=CARTESIAN_POINT('Ctrl Pts',(0.0866289535041628,0.059621470553197,
-0.458205881333311));
#47415=CARTESIAN_POINT('Ctrl Pts',(-0.00272759456705263,0.105127805855682,
-0.45187822031744));
#47416=CARTESIAN_POINT('Ctrl Pts',(-0.0896041377153937,0.0550490130741048,
-0.445550559301567));
#47417=CARTESIAN_POINT('Ctrl Pts',(-0.0950101040674725,-0.0450818750856725,
-0.439222898285696));
#47418=CARTESIAN_POINT('Ctrl Pts',(-0.0140302385014343,-0.104223067234394,
-0.432895237269823));
#47419=CARTESIAN_POINT('Ctrl Pts',(0.0797063105442395,-0.0686017448435343,
-0.426567576253952));
#47420=CARTESIAN_POINT('Ctrl Pts',(0.100971662835955,0.0293941939895359,
-0.420239915238079));
#47421=CARTESIAN_POINT('Ctrl Pts',(0.0304307679937315,0.100664113245306,
-0.413912254222208));
#47422=CARTESIAN_POINT('Ctrl Pts',(-0.0677786283710122,0.0804074180178444,
-0.407584593206336));
#47423=CARTESIAN_POINT('Ctrl Pts',(-0.104361808707819,-0.0129579403990236,
-0.401256932190463));
#47424=CARTESIAN_POINT('Ctrl Pts',(-0.0460563268945252,-0.0945415786262148,
-0.394929271174592));
#47425=CARTESIAN_POINT('Ctrl Pts',(0.0541248496454143,-0.0901653813113073,
-0.38860161015872));
#47426=CARTESIAN_POINT('Ctrl Pts',(0.105094205927356,-0.00380830889641988,
-0.382273949142848));
#47427=CARTESIAN_POINT('Ctrl Pts',(0.0605089841155697,0.0860113839991769,
-0.375946288126976));
#47428=CARTESIAN_POINT('Ctrl Pts',(-0.0390926907634774,0.0976271318078293,
-0.369618627111104));
#47429=CARTESIAN_POINT('Ctrl Pts',(-0.103150202769885,0.0204775732127567,
-0.363290966095232));
#47430=CARTESIAN_POINT('Ctrl Pts',(-0.0734206784788588,-0.0752907650901236,
-0.35696330507936));
#47431=CARTESIAN_POINT('Ctrl Pts',(0.0230649708858186,-0.102602643504875,
-0.350635644063488));
#47432=CARTESIAN_POINT('Ctrl Pts',(0.0985793065392342,-0.0366253417512498,
-0.344307983047616));
#47433=CARTESIAN_POINT('Ctrl Pts',(0.0844625920123951,0.0626527404564226,
-0.337980322031744));
#47434=CARTESIAN_POINT('Ctrl Pts',(-0.00644986280507308,0.10496520664462,
-0.331652661015872));
#47435=CARTESIAN_POINT('Ctrl Pts',(-0.0914979227811434,0.0518403844785903,
-0.325325));
#47436=CARTESIAN_POINT('Ctrl Pts',(-0.0933535238518378,-0.0484191586109931,
-0.318997338984129));
#47437=CARTESIAN_POINT('Ctrl Pts',(-0.010329501859476,-0.104654654590645,
-0.312669677968256));
#47438=CARTESIAN_POINT('Ctrl Pts',(0.0820863908206271,-0.0657352247900273,
-0.306342016952385));
#47439=CARTESIAN_POINT('Ctrl Pts',(0.0998670514925671,0.0329525016096368,
-0.300014355936512));
#47440=CARTESIAN_POINT('Ctrl Pts',(0.026845808418899,0.101678896072331,
-0.293686694920641));
#47441=CARTESIAN_POINT('Ctrl Pts',(-0.0705843911183263,0.0779560072515728,
-0.287359033904769));
#47442=CARTESIAN_POINT('Ctrl Pts',(-0.103837297018865,-0.0166466538369796,
-0.281031372888896));
#47443=CARTESIAN_POINT('Ctrl Pts',(-0.0426784414005113,-0.096113713775794,
-0.274703711873025));
#47444=CARTESIAN_POINT('Ctrl Pts',(0.0572848414052219,-0.0881915091226506,
-0.268376050857152));
#47445=CARTESIAN_POINT('Ctrl Pts',(0.1051631514635,-8.31289205999597E-5,
-0.262048389841281));
#47446=CARTESIAN_POINT('Ctrl Pts',(0.0574241962269787,0.0881008344105628,
-0.255720728825408));
#47447=CARTESIAN_POINT('Ctrl Pts',(-0.0425264370408898,0.0961810661656361,
-0.249393067809537));
#47448=CARTESIAN_POINT('Ctrl Pts',(-0.103810849717319,0.0168107946606686,
-0.243065406793664));
#47449=CARTESIAN_POINT('Ctrl Pts',(-0.0707075474977308,-0.0778443194010069,
-0.236737745777793));
#47450=CARTESIAN_POINT('Ctrl Pts',(0.02668502556757,-0.101721210898243,
-0.230410084761921));
#47451=CARTESIAN_POINT('Ctrl Pts',(0.0998148304144701,-0.0331103452942156,
-0.224082423746049));
#47452=CARTESIAN_POINT('Ctrl Pts',(0.0821902123736124,0.0656053681196284,
-0.217754762730176));
#47453=CARTESIAN_POINT('Ctrl Pts',(-0.0101640351214257,0.104670854234478,
-0.211427101714305));
#47454=CARTESIAN_POINT('Ctrl Pts',(-0.0932768588950464,0.0485666854021975,
-0.205099440698433));
#47455=CARTESIAN_POINT('Ctrl Pts',(-0.0915797655167434,-0.0516956660067222,
-0.198771779682561));
#47456=CARTESIAN_POINT('Ctrl Pts',(-0.00661579954317001,-0.104954878554757,
-0.192444118666689));
#47457=CARTESIAN_POINT('Ctrl Pts',(0.0843634355817327,-0.0627861933377942,
-0.186116457650817));
#47458=CARTESIAN_POINT('Ctrl Pts',(0.0986370861891049,0.0364694469785133,
-0.179788796634945));
#47459=CARTESIAN_POINT('Ctrl Pts',(0.0232271517771629,0.102566050700096,
-0.173461135619074));
#47460=CARTESIAN_POINT('Ctrl Pts',(-0.0733015557797646,0.0754067454663942,
-0.167133474603201));
#47461=CARTESIAN_POINT('Ctrl Pts',(-0.103182447839406,-0.0203144722733525,
-0.16080581358733));
#47462=CARTESIAN_POINT('Ctrl Pts',(-0.039246985673088,-0.0975652061623642,
-0.154478152571457));
#47463=CARTESIAN_POINT('Ctrl Pts',(0.0603729289472908,-0.0861069382789412,
-0.148150491555585));
#47464=CARTESIAN_POINT('Ctrl Pts',(0.10510009497664,0.00364215551222339,
-0.141822830539713));
#47465=CARTESIAN_POINT('Ctrl Pts',(0.0542673296971727,0.090079699708902,
-0.135495169523841));
#47466=CARTESIAN_POINT('Ctrl Pts',(-0.0459068050839857,0.0946142736566952,
-0.129167508507969));
#47467=CARTESIAN_POINT('Ctrl Pts',(-0.10434118995342,0.0131229142891147,
-0.122839847492097));
#47468=CARTESIAN_POINT('Ctrl Pts',(-0.0679056685023866,-0.0803001614144492,
-0.116512186476226));
#47469=CARTESIAN_POINT('Ctrl Pts',(0.0302715938731016,-0.100712099754892,
-0.110184525460353));
#47470=CARTESIAN_POINT('Ctrl Pts',(0.100925049024152,-0.0295537831991381,
-0.103856864444482));
#47471=CARTESIAN_POINT('Ctrl Pts',(0.0798146988809391,0.0684756374071776,
-0.0975292034286096));
#47472=CARTESIAN_POINT('Ctrl Pts',(-0.0138655101223774,0.104245137015464,
-0.0912015424127377));
#47473=CARTESIAN_POINT('Ctrl Pts',(-0.0949385980496625,0.0452319891380204,
-0.0848738813968657));
#47474=CARTESIAN_POINT('Ctrl Pts',(-0.0896912737678446,-0.054907216513919,
-0.0785462203809937));
#47475=CARTESIAN_POINT('Ctrl Pts',(-0.00289337900745932,-0.105123491379144,
-0.0722185593651219));
#47476=CARTESIAN_POINT('Ctrl Pts',(0.0865338013551485,-0.0597581072652013,
-0.06589089834925));
#47477=CARTESIAN_POINT('Ctrl Pts',(0.0972848003668635,0.0399401511237437,
-0.0595632373333777));
#47478=CARTESIAN_POINT('Ctrl Pts',(0.019576514766986,0.103325344594117,
-0.0532355763175061));
#47479=CARTESIAN_POINT('Ctrl Pts',(-0.0759213521544111,0.0727611612640329,
-0.0469079153016338));
#47480=CARTESIAN_POINT('Ctrl Pts',(-0.102408251140003,-0.0239536208583187,
-0.0405802542857621));
#47481=CARTESIAN_POINT('Ctrl Pts',(-0.0357469642855133,-0.0989002564218097,
-0.0342525932698899));
#47482=CARTESIAN_POINT('Ctrl Pts',(0.0633484888350438,-0.0839027956787714,
-0.0279249322540183));
#47483=CARTESIAN_POINT('Ctrl Pts',(0.104975946162434,0.00734051878504697,
-0.021597271238146));
#47484=CARTESIAN_POINT('Ctrl Pts',(0.0508985244218387,0.0919925081829091,
-0.0152696102222743));
#47485=CARTESIAN_POINT('Ctrl Pts',(-0.015621146325174,0.0925361401510375,
-0.0110511695450261));
#47486=CARTESIAN_POINT('Ctrl Pts',(-0.0417021627450121,0.0787195649134718,
-0.00894194920640216));
#47487=CARTESIAN_POINT('Ctrl Pts',(-0.066285514675037,-0.0474038213689209,
-0.953708050793598));
#47488=CARTESIAN_POINT('Ctrl Pts',(-0.050579891240191,-0.0693652435202928,
-0.951598830454974));
#47489=CARTESIAN_POINT('Ctrl Pts',(0.00409160755877578,-0.0960879603017703,
-0.947380389777727));
#47490=CARTESIAN_POINT('Ctrl Pts',(0.0829297499285808,-0.0488824263373707,
-0.941052728761854));
#47491=CARTESIAN_POINT('Ctrl Pts',(0.0861209628817152,0.0428058306209787,
-0.934725067745982));
#47492=CARTESIAN_POINT('Ctrl Pts',(0.0111318907798004,0.0955541350326624,
-0.92839740673011));
#47493=CARTESIAN_POINT('Ctrl Pts',(-0.0740429126153175,0.0614323416473282,
-0.922069745714238));
#47494=CARTESIAN_POINT('Ctrl Pts',(-0.0918620182971786,-0.028550920325338,
-0.915742084698367));
#47495=CARTESIAN_POINT('Ctrl Pts',(-0.0261754395083107,-0.0925720052086505,
-0.909414423682494));
#47496=CARTESIAN_POINT('Ctrl Pts',(0.0633199713564921,-0.0724255667246425,
-0.903086762666622));
#47497=CARTESIAN_POINT('Ctrl Pts',(0.0952381490570246,0.013573015491322,
-0.89675910165075));
#47498=CARTESIAN_POINT('Ctrl Pts',(0.0405657607957116,0.0872302113178526,
-0.890431440634878));
#47499=CARTESIAN_POINT('Ctrl Pts',(-0.0509915230471101,0.081575493225651,
-0.884103779619006));
#47500=CARTESIAN_POINT('Ctrl Pts',(-0.0961851687622249,0.00174994792922621,
-0.877776118603136));
#47501=CARTESIAN_POINT('Ctrl Pts',(-0.0539249635872344,-0.0796666367934459,
-0.871448457587261));
#47502=CARTESIAN_POINT('Ctrl Pts',(0.0373655215653255,-0.0886481299030314,
-0.865120796571392));
#47503=CARTESIAN_POINT('Ctrl Pts',(0.094682127837785,-0.0170282579173243,
-0.858793135555518));
#47504=CARTESIAN_POINT('Ctrl Pts',(0.0659111633695569,0.0700741711945603,
-0.852465474539647));
#47505=CARTESIAN_POINT('Ctrl Pts',(-0.022788095506527,0.0934632176161583,
-0.846137813523775));
#47506=CARTESIAN_POINT('Ctrl Pts',(-0.0907677678942492,0.0318729018268572,
-0.839810152507903));
#47507=CARTESIAN_POINT('Ctrl Pts',(-0.0762188667431783,-0.058697142388134,
-0.83348249149203));
#47508=CARTESIAN_POINT('Ctrl Pts',(0.00763035449001975,-0.0958981111815948,
-0.827154830476159));
#47509=CARTESIAN_POINT('Ctrl Pts',(0.0845418426911846,-0.0459058468948889,
-0.820827169460287));
#47510=CARTESIAN_POINT('Ctrl Pts',(0.0845855348816854,0.0458252913181626,
-0.814499508444415));
#47511=CARTESIAN_POINT('Ctrl Pts',(0.00772170306722385,0.0958907988859224,
-0.808171847428543));
#47512=CARTESIAN_POINT('Ctrl Pts',(-0.0761629158314008,0.0587697222318829,
-0.801844186412671));
#47513=CARTESIAN_POINT('Ctrl Pts',(-0.0907980912816151,-0.0317864221311527,
-0.795516525396799));
#47514=CARTESIAN_POINT('Ctrl Pts',(-0.0228771140177608,-0.0934414665004511,
-0.789188864380927));
#47515=CARTESIAN_POINT('Ctrl Pts',(0.0658443722135284,-0.0701369278941099,
-0.782861203365055));
#47516=CARTESIAN_POINT('Ctrl Pts',(0.094698321995253,0.0169380583228695,
-0.776533542349183));
#47517=CARTESIAN_POINT('Ctrl Pts',(0.0374499207860274,0.0886124903203744,
-0.770205881333311));
#47518=CARTESIAN_POINT('Ctrl Pts',(-0.0538489910866597,0.0797179789417516,
-0.76387822031744));
#47519=CARTESIAN_POINT('Ctrl Pts',(-0.096186900987293,-0.00165833842210959,
-0.757550559301566));
#47520=CARTESIAN_POINT('Ctrl Pts',(-0.0510690024435771,-0.0815268483209539,
-0.751222898285696));
#47521=CARTESIAN_POINT('Ctrl Pts',(0.040482254999354,-0.0872688778311181,
-0.744895237269823));
#47522=CARTESIAN_POINT('Ctrl Pts',(0.0952259190782751,-0.0136636138509041,
-0.738567576253951));
#47523=CARTESIAN_POINT('Ctrl Pts',(0.0633875262221782,0.0723649882690567,
-0.732239915238079));
#47524=CARTESIAN_POINT('Ctrl Pts',(-0.0260845703295907,0.0925973282469388,
-0.725912254222209));
#47525=CARTESIAN_POINT('Ctrl Pts',(-0.0918398492833032,0.0286375992599782,
-0.719584593206334));
#47526=CARTESIAN_POINT('Ctrl Pts',(-0.0740917802358122,-0.0613602323108368,
-0.713256932190464));
#47527=CARTESIAN_POINT('Ctrl Pts',(0.0110225982877466,-0.095567632254542,
-0.706929271174592));
#47528=CARTESIAN_POINT('Ctrl Pts',(0.0861149235535926,-0.0428822801295805,
-0.700601610158719));
#47529=CARTESIAN_POINT('Ctrl Pts',(0.0829091626868333,0.0487928350305729,
-0.694273949142848));
#47530=CARTESIAN_POINT('Ctrl Pts',(0.00432008272329617,0.0961041460761004,
-0.687946288126975));
#47531=CARTESIAN_POINT('Ctrl Pts',(-0.0781969367333093,0.056034891748619,
-0.681618627111104));
#47532=CARTESIAN_POINT('Ctrl Pts',(-0.0896151241292935,-0.0349828462970623,
-0.675290966095232));
#47533=CARTESIAN_POINT('Ctrl Pts',(-0.0195527455756119,-0.0941932064864976,
-0.668963305079359));
#47534=CARTESIAN_POINT('Ctrl Pts',(0.0682875336488553,-0.0677604807827472,
-0.662635644063488));
#47535=CARTESIAN_POINT('Ctrl Pts',(0.0940388859976769,0.0202819606564187,
-0.656307983047616));
#47536=CARTESIAN_POINT('Ctrl Pts',(0.0342874649383861,0.089883478770303,
-0.649980322031744));
#47537=CARTESIAN_POINT('Ctrl Pts',(-0.0566390738848248,0.0777604354233048,
-0.643652661015872));
#47538=CARTESIAN_POINT('Ctrl Pts',(-0.0960677897697764,-0.00506456084005674,
-0.637325000000001));
#47539=CARTESIAN_POINT('Ctrl Pts',(-0.0481489964476719,-0.0832847173786083,
-0.630997338984128));
#47540=CARTESIAN_POINT('Ctrl Pts',(0.0435482050235359,-0.0857800900383107,
-0.624669677968256));
#47541=CARTESIAN_POINT('Ctrl Pts',(0.0956501660050871,-0.010281816520044,
-0.618342016952384));
#47542=CARTESIAN_POINT('Ctrl Pts',(0.0607843329340448,0.0745649708476828,
-0.612014355936513));
#47543=CARTESIAN_POINT('Ctrl Pts',(-0.0293483080163605,0.0916152106602906,
-0.60568669492064));
#47544=CARTESIAN_POINT('Ctrl Pts',(-0.0927966501938481,0.0253663501622369,
-0.599359033904769));
#47545=CARTESIAN_POINT('Ctrl Pts',(-0.0718716943427677,-0.0639463021608941,
-0.593031372888896));
#47546=CARTESIAN_POINT('Ctrl Pts',(0.0144010070781465,-0.0951171961471098,
-0.586703711873026));
#47547=CARTESIAN_POINT('Ctrl Pts',(0.0875799119064274,-0.0398048871147124,
-0.580376050857152));
#47548=CARTESIAN_POINT('Ctrl Pts',(0.0811287224030647,0.0516991335420534,
-0.574048389841281));
#47549=CARTESIAN_POINT('Ctrl Pts',(0.000913039680479169,0.0961968625595162,
-0.567720728825409));
#47550=CARTESIAN_POINT('Ctrl Pts',(-0.0801328041407242,0.0532297257958081,
-0.561393067809536));
#47551=CARTESIAN_POINT('Ctrl Pts',(-0.0883196713554814,-0.0381353596995275,
-0.555065406793665));
#47552=CARTESIAN_POINT('Ctrl Pts',(-0.0162038343509091,-0.0948267143798671,
-0.548737745777793));
#47553=CARTESIAN_POINT('Ctrl Pts',(0.0706449799975524,-0.0652989801520513,
-0.542410084761921));
#47554=CARTESIAN_POINT('Ctrl Pts',(0.0932614116134009,0.023600404903908,
-0.536082423746049));
#47555=CARTESIAN_POINT('Ctrl Pts',(0.0310819711779969,0.0910416447316434,
-0.529754762730177));
#47556=CARTESIAN_POINT('Ctrl Pts',(-0.0593580628460573,0.0757052863604391,
-0.523427101714304));
#47557=CARTESIAN_POINT('Ctrl Pts',(-0.095828093465389,-0.00846442617909054,
-0.517099440698433));
#47558=CARTESIAN_POINT('Ctrl Pts',(-0.0451685534313103,-0.0849380467674849,
-0.510771779682561));
#47559=CARTESIAN_POINT('Ctrl Pts',(0.0465594929790022,-0.0841836303641677,
-0.504444118666689));
#47560=CARTESIAN_POINT('Ctrl Pts',(0.095954352049361,-0.00688711336772415,
-0.498116457650817));
#47561=CARTESIAN_POINT('Ctrl Pts',(0.0581048426464326,0.0766713588557415,
-0.491788796634945));
#47562=CARTESIAN_POINT('Ctrl Pts',(-0.0325752074631849,0.0905180969004709,
-0.485461135619073));
#47563=CARTESIAN_POINT('Ctrl Pts',(-0.0936369719785242,0.0220632610111395,
-0.479133474603201));
#47564=CARTESIAN_POINT('Ctrl Pts',(-0.069561394502176,-0.0664521060814872,
-0.47280581358733));
#47565=CARTESIAN_POINT('Ctrl Pts',(0.0177613396048748,-0.0945473681452471,
-0.466478152571457));
#47566=CARTESIAN_POINT('Ctrl Pts',(0.0889349692265999,-0.0366775306750104,
-0.460150491555585));
#47567=CARTESIAN_POINT('Ctrl Pts',(0.0792464486732655,0.054540538871816,
-0.453822830539714));
#47568=CARTESIAN_POINT('Ctrl Pts',(-0.0024951494173252,0.0961688319422557,
-0.447495169523841));
#47569=CARTESIAN_POINT('Ctrl Pts',(-0.0819680881869817,0.0503577454491741,
-0.44116750850797));
#47570=CARTESIAN_POINT('Ctrl Pts',(-0.0869133589968021,-0.0412400052818326,
-0.434839847492097));
#47571=CARTESIAN_POINT('Ctrl Pts',(-0.0128345839387771,-0.0953411949939326,
-0.428512186476226));
#47572=CARTESIAN_POINT('Ctrl Pts',(0.0729137521807407,-0.0627555156992445,
-0.422184525460353));
#47573=CARTESIAN_POINT('Ctrl Pts',(0.0923668747308512,0.026889225727191,
-0.415856864444482));
#47574=CARTESIAN_POINT('Ctrl Pts',(0.0278374630692892,0.0920855344645321,
-0.409529203428609));
#47575=CARTESIAN_POINT('Ctrl Pts',(-0.0620025450739129,0.0735551113934987,
-0.403201542412738));
#47576=CARTESIAN_POINT('Ctrl Pts',(-0.0954681129423542,-0.0118536669000983,
-0.396873881396865));
#47577=CARTESIAN_POINT('Ctrl Pts',(-0.0421314144716149,-0.0864847612147573,
-0.390546220380994));
#47578=CARTESIAN_POINT('Ctrl Pts',(0.0495123390722645,-0.0824815026981547,
-0.384218559365122));
#47579=CARTESIAN_POINT('Ctrl Pts',(0.0961380953941644,-0.0034837654535165,
-0.37789089834925));
#47580=CARTESIAN_POINT('Ctrl Pts',(0.0553524186778445,0.0786815083375071,
-0.371563237333378));
#47581=CARTESIAN_POINT('Ctrl Pts',(-0.0357612182391062,0.0893073640737851,
-0.365235576317505));
#47582=CARTESIAN_POINT('Ctrl Pts',(-0.094359759858438,0.0187324778716134,
-0.358907915301635));
#47583=CARTESIAN_POINT('Ctrl Pts',(-0.0671637806215868,-0.0688744987667276,
-0.352580254285761));
#47584=CARTESIAN_POINT('Ctrl Pts',(0.0210993779506474,-0.0938588635017939,
-0.346252593269891));
#47585=CARTESIAN_POINT('Ctrl Pts',(0.0901783946349084,-0.0335041362942443,
-0.339924932254018));
#47586=CARTESIAN_POINT('Ctrl Pts',(0.0772647041430507,0.0573134844642988,
-0.333597271238147));
#47587=CARTESIAN_POINT('Ctrl Pts',(-0.00590020658286327,0.0960200894085823,
-0.327269610222274));
#47588=CARTESIAN_POINT('Ctrl Pts',(-0.0837004852083069,0.047422555642295,
-0.320941949206402));
#47589=CARTESIAN_POINT('Ctrl Pts',(-0.0853979522682061,-0.0442928860670627,
-0.31461428819053));
#47590=CARTESIAN_POINT('Ctrl Pts',(-0.00944922345031021,-0.0957360025483553,
-0.308286627174658));
#47591=CARTESIAN_POINT('Ctrl Pts',(0.0750910024167363,-0.0601332800020278,
-0.301958966158787));
#47592=CARTESIAN_POINT('Ctrl Pts',(0.091356398180151,0.0301442949710606,
-0.295631305142914));
#47593=CARTESIAN_POINT('Ctrl Pts',(0.0245580131457824,0.0930138376699088,
-0.289303644127042));
#47594=CARTESIAN_POINT('Ctrl Pts',(-0.0645692011923398,0.0713126094399562,
-0.282975983111171));
#47595=CARTESIAN_POINT('Ctrl Pts',(-0.0949883000512143,-0.0152280287999835,
-0.276648322095299));
#47596=CARTESIAN_POINT('Ctrl Pts',(-0.0390413918106268,-0.087922919271608,
-0.270320661079426));
#47597=CARTESIAN_POINT('Ctrl Pts',(0.0524030368663857,-0.0806758435650515,
-0.263993000063555));
#47598=CARTESIAN_POINT('Ctrl Pts',(0.0962011654033275,-7.60446879838475E-5,
-0.257665339047683));
#47599=CARTESIAN_POINT('Ctrl Pts',(0.0525305158936973,0.0805928961366598,
-0.251337678031811));
#47600=CARTESIAN_POINT('Ctrl Pts',(-0.0389023412369373,0.0879845319021287,
-0.245010017015939));
#47601=CARTESIAN_POINT('Ctrl Pts',(-0.0949641065842529,0.015378181570316,
-0.238682356000067));
#47602=CARTESIAN_POINT('Ctrl Pts',(-0.0646818622058288,-0.0712104396092091,
-0.232354694984195));
#47603=CARTESIAN_POINT('Ctrl Pts',(0.0244109321819707,-0.093052546433482,
-0.226027033968323));
#47604=CARTESIAN_POINT('Ctrl Pts',(0.0913086273735362,-0.0302886872434177,
-0.219699372952451));
#47605=CARTESIAN_POINT('Ctrl Pts',(0.075185976314458,0.0600144896952148,
-0.213371711936579));
#47606=CARTESIAN_POINT('Ctrl Pts',(-0.00929785775981484,0.0957508216612688,
-0.207044050920707));
#47607=CARTESIAN_POINT('Ctrl Pts',(-0.0853278206861234,0.0444278406499617,
-0.200716389904835));
#47608=CARTESIAN_POINT('Ctrl Pts',(-0.08377535331976,-0.0472901700542316,
-0.194388728888963));
#47609=CARTESIAN_POINT('Ctrl Pts',(-0.0060520022200805,-0.0960106414767981,
-0.188061067873091));
#47610=CARTESIAN_POINT('Ctrl Pts',(0.0771739978067131,-0.0574355645135913,
-0.181733406857219));
#47611=CARTESIAN_POINT('Ctrl Pts',(0.0902312503127462,0.0333615268477907,
-0.175405745841347));
#47612=CARTESIAN_POINT('Ctrl Pts',(0.0212477378137396,0.0938253891296762,
-0.169078084825475));
#47613=CARTESIAN_POINT('Ctrl Pts',(-0.0670548095388511,0.0689805953148616,
-0.162750423809603));
#47614=CARTESIAN_POINT('Ctrl Pts',(-0.094389257008564,-0.0185832763668021,
-0.156422762793732));
#47615=CARTESIAN_POINT('Ctrl Pts',(-0.0359023641625004,-0.0892507157213992,
-0.150095101777859));
#47616=CARTESIAN_POINT('Ctrl Pts',(0.055227958108097,-0.0787689194976396,
-0.143767440761988));
#47617=CARTESIAN_POINT('Ctrl Pts',(0.0961434825796593,0.003331771632744,
-0.137439779746115));
#47618=CARTESIAN_POINT('Ctrl Pts',(0.0496426769980031,0.082403122867479,
-0.131112118730244));
#47619=CARTESIAN_POINT('Ctrl Pts',(-0.0419946348845927,0.0865512611869807,
-0.124784457714371));
#47620=CARTESIAN_POINT('Ctrl Pts',(-0.095449251314733,0.0120045817430545,
-0.1184567966985));
#47621=CARTESIAN_POINT('Ctrl Pts',(-0.0621187588666827,-0.0734569951797847,
-0.112129135682628));
#47622=CARTESIAN_POINT('Ctrl Pts',(0.0276918537404171,-0.0921294315718511,
-0.105801474666756));
#47623=CARTESIAN_POINT('Ctrl Pts',(0.0923242333402416,-0.0270352147712229,
-0.0994738136508837));
#47624=CARTESIAN_POINT('Ctrl Pts',(0.0730129036816374,0.0626401551173798,
-0.0931461526350118));
#47625=CARTESIAN_POINT('Ctrl Pts',(-0.0126838936844461,0.0953613839919759,
-0.0868184916191398));
#47626=CARTESIAN_POINT('Ctrl Pts',(-0.0868479467097893,0.041377326639916,
-0.0804908306032678));
#47627=CARTESIAN_POINT('Ctrl Pts',(-0.0820477985197149,-0.0502280327679713,
-0.0741631695873958));
#47628=CARTESIAN_POINT('Ctrl Pts',(-0.0026468057356357,-0.096164885144682,
-0.067835508571524));
#47629=CARTESIAN_POINT('Ctrl Pts',(0.0791594053743683,-0.0546655314262305,
-0.0615078475556519));
#47630=CARTESIAN_POINT('Ctrl Pts',(0.0889942060605761,0.0365364581701673,
-0.0551801865397797));
#47631=CARTESIAN_POINT('Ctrl Pts',(0.0179082074748696,0.0945199761258996,
-0.0488525255239083));
#47632=CARTESIAN_POINT('Ctrl Pts',(-0.0694513473075758,0.0665604673527576,
-0.0425248645080359));
#47633=CARTESIAN_POINT('Ctrl Pts',(-0.0936810372215236,-0.0219122973221233,
-0.0361972034921643));
#47634=CARTESIAN_POINT('Ctrl Pts',(-0.0327006140082352,-0.0904719932225328,
-0.029869542476292));
#47635=CARTESIAN_POINT('Ctrl Pts',(0.0579499412832453,-0.0767526135587191,
-0.0235418814604204));
#47636=CARTESIAN_POINT('Ctrl Pts',(0.0960299137064959,0.00671496101019401,
-0.0172142204445481));
#47637=CARTESIAN_POINT('Ctrl Pts',(0.0465609607409879,0.0841529221254132,
-0.0108865594286764));
#47638=CARTESIAN_POINT('Ctrl Pts',(-0.0142899148656573,0.0846502258687555,
-0.00666811875142826));
#47639=CARTESIAN_POINT('Ctrl Pts',(-0.0381483114577617,0.0720110968464772,
-0.00455889841280429));
#47640=CARTESIAN_POINT('Ctrl Pts',(-0.0601104350279403,-0.0429877377952337,
-0.949325));
#47641=CARTESIAN_POINT('Ctrl Pts',(-0.0458679287777906,-0.0629032599997909,
-0.947215779661376));
#47642=CARTESIAN_POINT('Ctrl Pts',(0.00371043826886423,-0.0871365202941097,
-0.942997338984126));
#47643=CARTESIAN_POINT('Ctrl Pts',(0.0752041131369929,-0.0443285976848148,
-0.936669677968258));
#47644=CARTESIAN_POINT('Ctrl Pts',(0.0780980364899326,0.0388180903923549,
-0.930342016952383));
#47645=CARTESIAN_POINT('Ctrl Pts',(0.0100948570851079,0.0866524255516566,
-0.924014355936512));
#47646=CARTESIAN_POINT('Ctrl Pts',(-0.0671451630097795,0.055709377822733,
-0.91768669492064));
#47647=CARTESIAN_POINT('Ctrl Pts',(-0.0833042620165027,-0.0258911505721542,
-0.911359033904769));
#47648=CARTESIAN_POINT('Ctrl Pts',(-0.0237369667204929,-0.0839481073924034,
-0.905031372888896));
#47649=CARTESIAN_POINT('Ctrl Pts',(0.0574211581950477,-0.0656784871371439,
-0.898703711873025));
#47650=CARTESIAN_POINT('Ctrl Pts',(0.0863658764533893,0.0123085695241889,
-0.892376050857153));
#47651=CARTESIAN_POINT('Ctrl Pts',(0.0367867028056418,0.0791039486621042,
-0.88604838984128));
#47652=CARTESIAN_POINT('Ctrl Pts',(-0.0462412134555447,0.0739760173765286,
-0.879720728825409));
#47653=CARTESIAN_POINT('Ctrl Pts',(-0.0872246729300961,0.00158692486311266,
-0.873393067809536));
#47654=CARTESIAN_POINT('Ctrl Pts',(-0.0489013781666423,-0.0722449877374248,
-0.867065406793666));
#47655=CARTESIAN_POINT('Ctrl Pts',(0.0338845940526951,-0.0803897756396443,
-0.860737745777792));
#47656=CARTESIAN_POINT('Ctrl Pts',(0.0858616535090988,-0.0154419256785799,
-0.854410084761921));
#47657=CARTESIAN_POINT('Ctrl Pts',(0.0597709578444863,0.0635461448157645,
-0.848082423746049));
#47658=CARTESIAN_POINT('Ctrl Pts',(-0.0206651836539401,0.0847562955128429,
-0.841754762730177));
#47659=CARTESIAN_POINT('Ctrl Pts',(-0.0823119506786178,0.0289036602311659,
-0.835427101714305));
#47660=CARTESIAN_POINT('Ctrl Pts',(-0.0691184078411397,-0.0532289864708019,
-0.829099440698434));
#47661=CARTESIAN_POINT('Ctrl Pts',(0.00691951974818428,-0.0869643572919913,
-0.82277177968256));
#47662=CARTESIAN_POINT('Ctrl Pts',(0.0766660252567158,-0.0416293128401549,
-0.81644411866669));
#47663=CARTESIAN_POINT('Ctrl Pts',(0.0767056471347569,0.0415562617250705,
-0.810116457650816));
#47664=CARTESIAN_POINT('Ctrl Pts',(0.00700235840066891,0.0869577262010798,
-0.803788796634946));
#47665=CARTESIAN_POINT('Ctrl Pts',(-0.0690676692497047,0.0532948048626995,
-0.797461135619073));
#47666=CARTESIAN_POINT('Ctrl Pts',(-0.0823394491753107,-0.0288252368809756,
-0.791133474603202));
#47667=CARTESIAN_POINT('Ctrl Pts',(-0.0207459093066268,-0.0847365707051847,
-0.784805813587329));
#47668=CARTESIAN_POINT('Ctrl Pts',(0.0597103888730514,-0.0636030551758837,
-0.778478152571458));
#47669=CARTESIAN_POINT('Ctrl Pts',(0.0858763390381331,0.0153601289709793,
-0.772150491555585));
#47670=CARTESIAN_POINT('Ctrl Pts',(0.0339611307424576,0.0803574561980857,
-0.765822830539714));
#47671=CARTESIAN_POINT('Ctrl Pts',(-0.0488324831737906,0.0722915469123074,
-0.759495169523841));
#47672=CARTESIAN_POINT('Ctrl Pts',(-0.0872262437831388,-0.0015038495886356,
-0.75316750850797));
#47673=CARTESIAN_POINT('Ctrl Pts',(-0.0463114749636612,-0.0739319041732507,
-0.746839847492097));
#47674=CARTESIAN_POINT('Ctrl Pts',(0.0367109763098753,-0.0791390130490189,
-0.740512186476226));
#47675=CARTESIAN_POINT('Ctrl Pts',(0.0863547858049027,-0.0123907278484321,
-0.734184525460353));
#47676=CARTESIAN_POINT('Ctrl Pts',(0.0574824197298575,0.0656235520983735,
-0.727856864444481));
#47677=CARTESIAN_POINT('Ctrl Pts',(-0.0236545628063002,0.0839710713665869,
-0.72152920342861));
#47678=CARTESIAN_POINT('Ctrl Pts',(-0.083284158241572,0.025969754600418,
-0.715201542412737));
#47679=CARTESIAN_POINT('Ctrl Pts',(-0.0671894781809166,-0.055643986106197,
-0.708873881396866));
#47680=CARTESIAN_POINT('Ctrl Pts',(0.00999574615152227,-0.0866646653884117,
-0.702546220380994));
#47681=CARTESIAN_POINT('Ctrl Pts',(0.0780925597784293,-0.0388874179557339,
-0.696218559365122));
#47682=CARTESIAN_POINT('Ctrl Pts',(0.0751854437781816,0.0442473525975172,
-0.68989089834925));
#47683=CARTESIAN_POINT('Ctrl Pts',(0.00391762895901338,0.0871511982209692,
-0.683563237333377));
#47684=CARTESIAN_POINT('Ctrl Pts',(-0.0709122031854983,0.050814747931972,
-0.677235576317507));
#47685=CARTESIAN_POINT('Ctrl Pts',(-0.0812666858348066,-0.0317238859763112,
-0.670907915301633));
#47686=CARTESIAN_POINT('Ctrl Pts',(-0.0177312350715336,-0.0854182794889314,
-0.664580254285763));
#47687=CARTESIAN_POINT('Ctrl Pts',(0.0619259482971724,-0.0614479950487169,
-0.65825259326989));
#47688=CARTESIAN_POINT('Ctrl Pts',(0.0852783353131607,0.0183925173434011,
-0.651924932254018));
#47689=CARTESIAN_POINT('Ctrl Pts',(0.0310932855172931,0.0815100408768839,
-0.645597271238146));
#47690=CARTESIAN_POINT('Ctrl Pts',(-0.0513626451795302,0.0705163658179637,
-0.639269610222275));
#47691=CARTESIAN_POINT('Ctrl Pts',(-0.0871182288248673,-0.0045927523805729,
-0.632941949206402));
#47692=CARTESIAN_POINT('Ctrl Pts',(-0.0436634932506345,-0.0755260122418957,
-0.62661428819053));
#47693=CARTESIAN_POINT('Ctrl Pts',(0.0394913060792223,-0.0777889189548767,
-0.620286627174658));
#47694=CARTESIAN_POINT('Ctrl Pts',(0.0867395103929965,-0.00932397473154213,
-0.613958966158786));
#47695=CARTESIAN_POINT('Ctrl Pts',(0.0551217368298506,0.0676185869186267,
-0.607631305142914));
#47696=CARTESIAN_POINT('Ctrl Pts',(-0.0266142545750163,0.0830804466852906,
-0.601303644127043));
#47697=CARTESIAN_POINT('Ctrl Pts',(-0.0841518247181762,0.0230032511748356,
-0.59497598311117));
#47698=CARTESIAN_POINT('Ctrl Pts',(-0.0651762128470871,-0.0579891407672368,
-0.588648322095299));
#47699=CARTESIAN_POINT('Ctrl Pts',(0.013059426400348,-0.0862561913725913,
-0.582320661079426));
#47700=CARTESIAN_POINT('Ctrl Pts',(0.0794210715600979,-0.0360967112110921,
-0.575993000063554));
#47701=CARTESIAN_POINT('Ctrl Pts',(0.0735708671919806,0.046882903799052,
-0.569665339047683));
#47702=CARTESIAN_POINT('Ctrl Pts',(0.000827981990642192,0.087235277347151,
-0.56333767803181));
#47703=CARTESIAN_POINT('Ctrl Pts',(-0.0726677274895124,0.0482709079003198,
-0.55701001701594));
#47704=CARTESIAN_POINT('Ctrl Pts',(-0.0800919158994181,-0.0345827149826577,
-0.550682356000065));
#47705=CARTESIAN_POINT('Ctrl Pts',(-0.0146943044302958,-0.0859927705410227,
-0.544354694984196));
#47706=CARTESIAN_POINT('Ctrl Pts',(0.0640637777501068,-0.0592158048868383,
-0.538027033968322));
#47707=CARTESIAN_POINT('Ctrl Pts',(0.0845732895170916,0.0214018192747577,
-0.531699372952452));
#47708=CARTESIAN_POINT('Ctrl Pts',(0.0281864117401041,0.0825603134758373,
-0.525371711936578));
#47709=CARTESIAN_POINT('Ctrl Pts',(-0.0538283363655626,0.0686526719955389,
-0.519044050920707));
#47710=CARTESIAN_POINT('Ctrl Pts',(-0.0869008623428846,-0.00767589031150163,
-0.512716389904835));
#47711=CARTESIAN_POINT('Ctrl Pts',(-0.0409607047580388,-0.077025319432872,
-0.506388728888963));
#47712=CARTESIAN_POINT('Ctrl Pts',(0.0422220660331108,-0.0763411835637019,
-0.500061067873091));
#47713=CARTESIAN_POINT('Ctrl Pts',(0.0870153588274602,-0.00624551808415768,
-0.49373340685722));
#47714=CARTESIAN_POINT('Ctrl Pts',(0.0526918646680198,0.0695287463271004,
-0.487405745841347));
#47715=CARTESIAN_POINT('Ctrl Pts',(-0.0295405399103716,0.082085538737435,
-0.481078084825476));
#47716=CARTESIAN_POINT('Ctrl Pts',(-0.0849138631256316,0.0200078738773684,
-0.474750423809603));
#47717=CARTESIAN_POINT('Ctrl Pts',(-0.0630811377896817,-0.0602615069772603,
-0.468422762793731));
#47718=CARTESIAN_POINT('Ctrl Pts',(0.0161067143487094,-0.0857394478691125,
-0.46209510177786));
#47719=CARTESIAN_POINT('Ctrl Pts',(0.0806498933532556,-0.0332606955748025,
-0.455767440761988));
#47720=CARTESIAN_POINT('Ctrl Pts',(0.0718639438423683,0.049459607190435,
-0.449439779746115));
#47721=CARTESIAN_POINT('Ctrl Pts',(-0.00226270426759789,0.0872098580288294,
-0.443112118730244));
#47722=CARTESIAN_POINT('Ctrl Pts',(-0.0743320386585697,0.0456664778242435,
-0.436784457714372));
#47723=CARTESIAN_POINT('Ctrl Pts',(-0.0788166139261316,-0.0373981354779928,
-0.4304567966985));
#47724=CARTESIAN_POINT('Ctrl Pts',(-0.0116389293761198,-0.0864593227534712,
-0.424129135682628));
#47725=CARTESIAN_POINT('Ctrl Pts',(0.0661211938172418,-0.0569092865549545,
-0.417801474666756));
#47726=CARTESIAN_POINT('Ctrl Pts',(0.0837620866257479,0.0243842574648459,
-0.411473813650883));
#47727=CARTESIAN_POINT('Ctrl Pts',(0.0252441581448469,0.0835069556837582,
-0.405146152635012));
#47728=CARTESIAN_POINT('Ctrl Pts',(-0.0562264617768135,0.066702804769153,
-0.398818491619139));
#47729=CARTESIAN_POINT('Ctrl Pts',(-0.0865744171768889,-0.010749393401173,
-0.392490830603268));
#47730=CARTESIAN_POINT('Ctrl Pts',(-0.0382065020487046,-0.0784279438032996,
-0.386163169587396));
#47731=CARTESIAN_POINT('Ctrl Pts',(0.0448998284991146,-0.0747976240850022,
-0.379835508571524));
#47732=CARTESIAN_POINT('Ctrl Pts',(0.0871819848609725,-0.00315922201061306,
-0.373507847555652));
#47733=CARTESIAN_POINT('Ctrl Pts',(0.0501958532401191,0.0713516326758373,
-0.36718018653978));
#47734=CARTESIAN_POINT('Ctrl Pts',(-0.0324297457147349,0.0809875963397409,
-0.360852525523908));
#47735=CARTESIAN_POINT('Ctrl Pts',(-0.0855693169469914,0.0169873825304703,
-0.354524864508036));
#47736=CARTESIAN_POINT('Ctrl Pts',(-0.0609068827643145,-0.0624582324433317,
-0.348197203492164));
#47737=CARTESIAN_POINT('Ctrl Pts',(0.019133785015476,-0.0851150834987123,
-0.341869542476292));
#47738=CARTESIAN_POINT('Ctrl Pts',(0.0817774827305826,-0.030382930837239,
-0.33554188146042));
#47739=CARTESIAN_POINT('Ctrl Pts',(0.0700668162737063,0.0519742284721753,
-0.329214220444548));
#47740=CARTESIAN_POINT('Ctrl Pts',(-0.00535055036065351,0.0870749721725439,
-0.322886559428676));
#47741=CARTESIAN_POINT('Ctrl Pts',(-0.0759030476354704,0.0430047268059999,
-0.316558898412805));
#47742=CARTESIAN_POINT('Ctrl Pts',(-0.0774423806845742,-0.0401666135231323,
-0.310231237396932));
#47743=CARTESIAN_POINT('Ctrl Pts',(-0.00856894504114455,-0.0868173505060656,
-0.303903576381061));
#47744=CARTESIAN_POINT('Ctrl Pts',(0.0680956140128458,-0.0545313352140282,
-0.297575915365189));
#47745=CARTESIAN_POINT('Ctrl Pts',(0.0828457448677347,0.0273360883324843,
-0.291248254349316));
#47746=CARTESIAN_POINT('Ctrl Pts',(0.0222702178726658,0.0843487792674867,
-0.284920593333445));
#47747=CARTESIAN_POINT('Ctrl Pts',(-0.0585540112663533,0.0646692116283394,
-0.278592932317572));
#47748=CARTESIAN_POINT('Ctrl Pts',(-0.0861393030835636,-0.0138094037629872,
-0.272265271301701));
#47749=CARTESIAN_POINT('Ctrl Pts',(-0.0354043422207423,-0.0797321247674219,
-0.265937610285828));
#47750=CARTESIAN_POINT('Ctrl Pts',(0.0475212323275497,-0.0731601780074524,
-0.259609949269957));
#47751=CARTESIAN_POINT('Ctrl Pts',(0.0872391793431545,-6.89604553678452E-5,
-0.253282288254085));
#47752=CARTESIAN_POINT('Ctrl Pts',(0.0476368355604161,0.0730849578627569,
-0.246954627238213));
#47753=CARTESIAN_POINT('Ctrl Pts',(-0.035278245432985,0.0797879976386212,
-0.240626966222341));
#47754=CARTESIAN_POINT('Ctrl Pts',(-0.0861173634511866,0.0139455684799636,
-0.234299305206469));
#47755=CARTESIAN_POINT('Ctrl Pts',(-0.0586561769139268,-0.0645765598174114,
-0.227971644190597));
#47756=CARTESIAN_POINT('Ctrl Pts',(0.0221368387963713,-0.0843838819687206,
-0.221643983174725));
#47757=CARTESIAN_POINT('Ctrl Pts',(0.0828024243326025,-0.0274670291926198,
-0.215316322158853));
#47758=CARTESIAN_POINT('Ctrl Pts',(0.0681817402553036,0.0544236112708011,
-0.208988661142981));
#47759=CARTESIAN_POINT('Ctrl Pts',(-0.00843168039820402,0.0868307890880593,
-0.202661000127109));
#47760=CARTESIAN_POINT('Ctrl Pts',(-0.0773787824772003,0.0402889958977259,
-0.196333339111237));
#47761=CARTESIAN_POINT('Ctrl Pts',(-0.0759709411227765,-0.042884674101741,
-0.190005678095365));
#47762=CARTESIAN_POINT('Ctrl Pts',(-0.00548820489699097,-0.0870664043988389,
-0.183678017079493));
#47763=CARTESIAN_POINT('Ctrl Pts',(0.0699845600316936,-0.0520849356893883,
-0.177350356063621));
#47764=CARTESIAN_POINT('Ctrl Pts',(0.0818254144363875,0.0302536067170679,
-0.17102269504775));
#47765=CARTESIAN_POINT('Ctrl Pts',(0.0192683238503164,0.0850847275592565,
-0.164695034031877));
#47766=CARTESIAN_POINT('Ctrl Pts',(-0.0608080632979376,0.0625544451633288,
-0.158367373016005));
#47767=CARTESIAN_POINT('Ctrl Pts',(-0.0855960661777222,-0.0168520804602516,
-0.152039712000134));
#47768=CARTESIAN_POINT('Ctrl Pts',(-0.0325577426519127,-0.0809362252804344,
-0.145712050984262));
#47769=CARTESIAN_POINT('Ctrl Pts',(0.0500829872689032,-0.0714309007163379,
-0.139384389968389));
#47770=CARTESIAN_POINT('Ctrl Pts',(0.0871868701826791,0.00302138775326442,
-0.133056728952518));
#47771=CARTESIAN_POINT('Ctrl Pts',(0.0450180242988335,0.0747265460260562,
-0.126729067936645));
#47772=CARTESIAN_POINT('Ctrl Pts',(-0.0380824646851997,0.0784882487172661,
-0.120401406920774));
#47773=CARTESIAN_POINT('Ctrl Pts',(-0.0865573126760457,0.0108862491969944,
-0.114073745904902));
#47774=CARTESIAN_POINT('Ctrl Pts',(-0.056331849230979,-0.0666138289451202,
-0.10774608488903));
#47775=CARTESIAN_POINT('Ctrl Pts',(0.0251121136077328,-0.0835467633888102,
-0.101418423873158));
#47776=CARTESIAN_POINT('Ctrl Pts',(0.0837234176563311,-0.0245166463433077,
-0.0950907628572859));
#47777=CARTESIAN_POINT('Ctrl Pts',(0.0662111084823356,0.0568046728275819,
-0.0887631018414139));
#47778=CARTESIAN_POINT('Ctrl Pts',(-0.0115022772465146,0.0864776309684878,
-0.0824354408255419));
#47779=CARTESIAN_POINT('Ctrl Pts',(-0.0787572953699165,0.0375226641418117,
-0.07610777980967));
#47780=CARTESIAN_POINT('Ctrl Pts',(-0.0744043232715852,-0.0455488490220237,
-0.069780118793798));
#47781=CARTESIAN_POINT('Ctrl Pts',(-0.00240023246381204,-0.0872062789102198,
-0.0634524577779261));
#47782=CARTESIAN_POINT('Ctrl Pts',(0.071785009393588,-0.0495729555872598,
-0.057124796762054));
#47783=CARTESIAN_POINT('Ctrl Pts',(0.0807036117542888,0.033132765216591,
-0.050797135746182));
#47784=CARTESIAN_POINT('Ctrl Pts',(0.0162399001827532,0.0857146076576825,
-0.0444694747303104));
#47785=CARTESIAN_POINT('Ctrl Pts',(-0.0629813424607405,0.0603597734414823,
-0.0381418137144381));
#47786=CARTESIAN_POINT('Ctrl Pts',(-0.0849538233030444,-0.0198709737859279,
-0.0318141526985663));
#47787=CARTESIAN_POINT('Ctrl Pts',(-0.0296542637309572,-0.082043730023256,
-0.0254864916826941));
#47788=CARTESIAN_POINT('Ctrl Pts',(0.0525513937314469,-0.0696024314386667,
-0.0191588306668225));
#47789=CARTESIAN_POINT('Ctrl Pts',(0.0870838812505578,0.006089403235341,
-0.0128311696509503));
#47790=CARTESIAN_POINT('Ctrl Pts',(0.0422233970601371,0.0763133360679174,
-0.00650350863507852));
#47791=CARTESIAN_POINT('Ctrl Pts',(-0.0129586834061405,0.0767643115864734,
-0.00228506795783038));
#47792=CARTESIAN_POINT('Ctrl Pts',(-0.0345944601705113,0.0653026287794826,
-0.000175847619206415));
#47793=CARTESIAN_POINT('Ctrl Pts',(-0.0452560140322624,0.0854280329804664,
-0.013325));
#47794=CARTESIAN_POINT('Ctrl Pts',(-0.0169523777846916,0.100422054433319,
-0.0154342203386239));
#47795=CARTESIAN_POINT('Ctrl Pts',(0.0191418551589967,0.100127074336862,
-0.0175434406772479));
#47796=CARTESIAN_POINT('Ctrl Pts',(0.0469699533834549,0.0846685813418844,
-0.0196526610158718));
#47797=CARTESIAN_POINT('Ctrl Pts',(0.0747980516079155,0.0692100883469053,
-0.0217618813544959));
#47798=CARTESIAN_POINT('Ctrl Pts',(0.0943600151131444,0.0385880824534022,
-0.0238711016931199));
#47799=CARTESIAN_POINT('Ctrl Pts',(0.0966118398271697,0.00677390378019592,
-0.025980322031744));
#47800=CARTESIAN_POINT('Ctrl Pts',(0.0988636645411949,-0.0250402748930086,
-0.028089542370368));
#47801=CARTESIAN_POINT('Ctrl Pts',(0.0838053504640186,-0.0580466263459162,
-0.030198762708992));
#47802=CARTESIAN_POINT('Ctrl Pts',(0.0583528016004915,-0.0772623923760804,
-0.032307983047616));
#47803=CARTESIAN_POINT('Ctrl Pts',(0.0329002527369644,-0.0964781584062447,
-0.03441720338624));
#47804=CARTESIAN_POINT('Ctrl Pts',(-0.00294653091291341,-0.101903339013666,
-0.0365264237248639));
#47805=CARTESIAN_POINT('Ctrl Pts',(-0.0329269478204673,-0.0910603334462807,
-0.0386356440634878));
#47806=CARTESIAN_POINT('Ctrl Pts',(-0.0629073647280212,-0.0802173278788959,
-0.0407448644021118));
#47807=CARTESIAN_POINT('Ctrl Pts',(-0.0870214148932512,-0.0531061361367054,
-0.0428540847407358));
#47808=CARTESIAN_POINT('Ctrl Pts',(-0.0942877552996606,-0.0220577403373066,
-0.0449633050793598));
#47809=CARTESIAN_POINT('Ctrl Pts',(-0.0959679031622562,-0.014878625002527,
-0.0454510061565838));
#47810=CARTESIAN_POINT('Ctrl Pts',(-0.0967473007548937,-0.00748900998154789,
-0.0459387072338078));
#47811=CARTESIAN_POINT('Ctrl Pts',(-0.0966799176497682,-8.54770466914428E-5,
-0.0464264083110319));
#47812=CARTESIAN_POINT('Origin',(0.194007127343405,-0.0342086910003853,
0.04));
#47813=CARTESIAN_POINT('',(0.18738691397118,-0.0314029373205391,0.04));
#47814=CARTESIAN_POINT('',(0.186826537413779,-0.0345809907026646,0.04));
#47815=CARTESIAN_POINT('Origin',(0.,0.,0.04));
#47816=CARTESIAN_POINT('',(0.181204626554246,-0.0319512646907152,0.04));
#47817=CARTESIAN_POINT('',(0.208025165376232,-0.02957246303897,0.04));
#47818=CARTESIAN_POINT('',(0.181204626554246,-0.0319512646907152,0.04));
#47819=CARTESIAN_POINT('Origin',(0.181204626554246,-0.0319512646907152,
0.04));
#47820=CARTESIAN_POINT('',(0.186826537413779,-0.0345809907026646,0.185));
#47821=CARTESIAN_POINT('',(0.186826537413779,-0.0345809907026646,0.0925));
#47822=CARTESIAN_POINT('',(0.181204626554246,-0.0319512646907152,0.191));
#47823=CARTESIAN_POINT('',(0.181204626554246,-0.0319512646907152,0.04));
#47824=CARTESIAN_POINT('Ctrl Pts',(0.186826537413779,-0.0345809907026646,
0.185));
#47825=CARTESIAN_POINT('Ctrl Pts',(0.183970486442383,-0.033245033637782,
0.188051499118437));
#47826=CARTESIAN_POINT('Ctrl Pts',(0.181204626554246,-0.0319512646907152,
0.191));
#47827=CARTESIAN_POINT('Origin',(0.208025165376232,-0.02957246303897,0.04));
#47828=CARTESIAN_POINT('',(0.18738691397118,-0.0314029373205391,0.185));
#47829=CARTESIAN_POINT('',(0.18738691397118,-0.0314029373205391,0.0925));
#47830=CARTESIAN_POINT('Ctrl Pts',(0.181204626554246,-0.0319512646907152,
0.191));
#47831=CARTESIAN_POINT('Ctrl Pts',(0.18424617972193,-0.0316814993535168,
0.188051499118469));
#47832=CARTESIAN_POINT('Ctrl Pts',(0.18738691397118,-0.0314029373205392,
0.185));
#47833=CARTESIAN_POINT('Origin',(0.185119446294824,-0.0673779682351569,
0.04));
#47834=CARTESIAN_POINT('',(0.179087022852749,-0.0634652522703487,0.04));
#47835=CARTESIAN_POINT('',(0.17798329649608,-0.0664977155125527,0.04));
#47836=CARTESIAN_POINT('Origin',(0.,0.,0.04));
#47837=CARTESIAN_POINT('',(0.172903442224607,-0.0629317063719232,0.04));
#47838=CARTESIAN_POINT('',(0.19972959136832,-0.0652463817528892,0.04));
#47839=CARTESIAN_POINT('',(0.172903442224607,-0.0629317063719232,0.04));
#47840=CARTESIAN_POINT('Origin',(0.172903442224607,-0.0629317063719232,
0.04));
#47841=CARTESIAN_POINT('',(0.17798329649608,-0.0664977155125527,0.185));
#47842=CARTESIAN_POINT('',(0.17798329649608,-0.0664977155125527,0.0925));
#47843=CARTESIAN_POINT('',(0.172903442224607,-0.0629317063719232,0.191));
#47844=CARTESIAN_POINT('',(0.172903442224607,-0.0629317063719232,0.04));
#47845=CARTESIAN_POINT('Ctrl Pts',(0.17798329649608,-0.0664977155125527,
0.185));
#47846=CARTESIAN_POINT('Ctrl Pts',(0.17540262186618,-0.0646861065908373,
0.188051499118472));
#47847=CARTESIAN_POINT('Ctrl Pts',(0.172903442224607,-0.0629317063719232,
0.191));
#47848=CARTESIAN_POINT('Origin',(0.19972959136832,-0.0652463817528892,0.04));
#47849=CARTESIAN_POINT('',(0.179087022852749,-0.0634652522703487,0.185));
#47850=CARTESIAN_POINT('',(0.179087022852749,-0.0634652522703487,0.0925));
#47851=CARTESIAN_POINT('Ctrl Pts',(0.172903442224607,-0.0629317063719232,
0.191));
#47852=CARTESIAN_POINT('Ctrl Pts',(0.17594563162456,-0.063194199541203,
0.188051499118452));
#47853=CARTESIAN_POINT('Ctrl Pts',(0.179087022852749,-0.0634652522703487,
0.185));
#47854=CARTESIAN_POINT('Origin',(0.170607004545534,-0.0985000000000001,
0.04));
#47855=CARTESIAN_POINT('',(0.165345663167344,-0.0935992076448907,0.04));
#47856=CARTESIAN_POINT('',(0.163732123178242,-0.0963939408860593,0.04));
#47857=CARTESIAN_POINT('Origin',(0.,0.,0.04));
#47858=CARTESIAN_POINT('',(0.159348674296337,-0.0920000000000001,0.04));
#47859=CARTESIAN_POINT('',(0.185365334794732,-0.098937822173509,0.04));
#47860=CARTESIAN_POINT('',(0.159348674296337,-0.0920000000000001,0.04));
#47861=CARTESIAN_POINT('Origin',(0.159348674296337,-0.0920000000000001,
0.04));
#47862=CARTESIAN_POINT('',(0.163732123178242,-0.0963939408860593,0.185));
#47863=CARTESIAN_POINT('',(0.163732123178242,-0.0963939408860593,0.0925));
#47864=CARTESIAN_POINT('',(0.159348674296337,-0.0920000000000001,0.191));
#47865=CARTESIAN_POINT('',(0.159348674296337,-0.0920000000000001,0.04));
#47866=CARTESIAN_POINT('Ctrl Pts',(0.163732123178242,-0.0963939408860593,
0.185));
#47867=CARTESIAN_POINT('Ctrl Pts',(0.161505237382642,-0.0941617249279212,
0.188051499118436));
#47868=CARTESIAN_POINT('Ctrl Pts',(0.159348674296337,-0.0920000000000001,
0.191));
#47869=CARTESIAN_POINT('Origin',(0.185365334794732,-0.098937822173509,0.04));
#47870=CARTESIAN_POINT('',(0.165345663167344,-0.0935992076448907,0.185));
#47871=CARTESIAN_POINT('',(0.165345663167344,-0.0935992076448907,0.0925));
#47872=CARTESIAN_POINT('Ctrl Pts',(0.159348674296337,-0.0920000000000001,
0.191));
#47873=CARTESIAN_POINT('Ctrl Pts',(0.162299064543036,-0.0927867759536363,
0.188051499118462));
#47874=CARTESIAN_POINT('Ctrl Pts',(0.165345663167344,-0.0935992076448907,
0.185));
#47875=CARTESIAN_POINT('Origin',(0.150910755294439,-0.126629159108248,0.04));
#47876=CARTESIAN_POINT('',(0.146580359175541,-0.120889198458627,0.04));
#47877=CARTESIAN_POINT('',(0.144506032150084,-0.123361285143431,0.04));
#47878=CARTESIAN_POINT('Origin',(0.,0.,0.04));
#47879=CARTESIAN_POINT('',(0.140952177533892,-0.118272920182323,0.04));
#47880=CARTESIAN_POINT('',(0.165368846322791,-0.129623086932341,0.04));
#47881=CARTESIAN_POINT('',(0.140952177533892,-0.118272920182323,0.04));
#47882=CARTESIAN_POINT('Origin',(0.140952177533892,-0.118272920182323,0.04));
#47883=CARTESIAN_POINT('',(0.144506032150084,-0.123361285143431,0.185));
#47884=CARTESIAN_POINT('',(0.144506032150084,-0.123361285143431,0.0925));
#47885=CARTESIAN_POINT('',(0.140952177533892,-0.118272920182323,0.191));
#47886=CARTESIAN_POINT('',(0.140952177533892,-0.118272920182323,0.04));
#47887=CARTESIAN_POINT('Ctrl Pts',(0.144506032150084,-0.123361285143431,
0.185));
#47888=CARTESIAN_POINT('Ctrl Pts',(0.1427005979868,-0.120776286901188,0.188051499118426));
#47889=CARTESIAN_POINT('Ctrl Pts',(0.140952177533892,-0.118272920182323,
0.191));
#47890=CARTESIAN_POINT('Origin',(0.165368846322791,-0.129623086932341,0.04));
#47891=CARTESIAN_POINT('',(0.146580359175541,-0.120889198458627,0.185));
#47892=CARTESIAN_POINT('',(0.146580359175541,-0.120889198458627,0.0925));
#47893=CARTESIAN_POINT('Ctrl Pts',(0.140952177533892,-0.118272920182323,
0.191));
#47894=CARTESIAN_POINT('Ctrl Pts',(0.143721122512686,-0.1195600731311,0.188051499118447));
#47895=CARTESIAN_POINT('Ctrl Pts',(0.146580359175541,-0.120889198458627,
0.185));
#47896=CARTESIAN_POINT('Origin',(0.126629159108248,-0.150910755294439,0.04));
#47897=CARTESIAN_POINT('',(0.123361285143431,-0.144506032150084,0.04));
#47898=CARTESIAN_POINT('',(0.120889198458627,-0.146580359175541,0.04));
#47899=CARTESIAN_POINT('Origin',(0.,0.,0.04));
#47900=CARTESIAN_POINT('',(0.118272920182323,-0.140952177533892,0.04));
#47901=CARTESIAN_POINT('',(0.140347709136006,-0.15636981978718,0.04));
#47902=CARTESIAN_POINT('',(0.118272920182323,-0.140952177533892,0.04));
#47903=CARTESIAN_POINT('Origin',(0.118272920182323,-0.140952177533892,0.04));
#47904=CARTESIAN_POINT('',(0.120889198458627,-0.146580359175541,0.185));
#47905=CARTESIAN_POINT('',(0.120889198458627,-0.146580359175541,0.0925));
#47906=CARTESIAN_POINT('',(0.118272920182323,-0.140952177533892,0.191));
#47907=CARTESIAN_POINT('',(0.118272920182323,-0.140952177533892,0.04));
#47908=CARTESIAN_POINT('Ctrl Pts',(0.120889198458627,-0.146580359175541,
0.185));
#47909=CARTESIAN_POINT('Ctrl Pts',(0.119560073131107,-0.143721122512702,
0.18805149911843));
#47910=CARTESIAN_POINT('Ctrl Pts',(0.118272920182323,-0.140952177533892,
0.191));
#47911=CARTESIAN_POINT('Origin',(0.140347709136006,-0.15636981978718,0.04));
#47912=CARTESIAN_POINT('',(0.123361285143431,-0.144506032150084,0.185));
#47913=CARTESIAN_POINT('',(0.123361285143431,-0.144506032150084,0.0925));
#47914=CARTESIAN_POINT('Ctrl Pts',(0.118272920182323,-0.140952177533892,
0.191));
#47915=CARTESIAN_POINT('Ctrl Pts',(0.120776286901169,-0.142700597986787,
0.188051499118449));
#47916=CARTESIAN_POINT('Ctrl Pts',(0.123361285143431,-0.144506032150084,
0.185));
#47917=CARTESIAN_POINT('Origin',(0.0985,-0.170607004545534,0.04));
#47918=CARTESIAN_POINT('',(0.0963939408860592,-0.163732123178242,0.04));
#47919=CARTESIAN_POINT('',(0.0935992076448907,-0.165345663167344,0.04));
#47920=CARTESIAN_POINT('Origin',(0.,0.,0.04));
#47921=CARTESIAN_POINT('',(0.092,-0.159348674296337,0.04));
#47922=CARTESIAN_POINT('',(0.111062177826491,-0.178365334794732,0.04));
#47923=CARTESIAN_POINT('',(0.092,-0.159348674296337,0.04));
#47924=CARTESIAN_POINT('Origin',(0.092,-0.159348674296337,0.04));
#47925=CARTESIAN_POINT('',(0.0935992076448907,-0.165345663167344,0.185));
#47926=CARTESIAN_POINT('',(0.0935992076448907,-0.165345663167344,0.0925));
#47927=CARTESIAN_POINT('',(0.092,-0.159348674296337,0.191));
#47928=CARTESIAN_POINT('',(0.092,-0.159348674296337,0.04));
#47929=CARTESIAN_POINT('Ctrl Pts',(0.0935992076448907,-0.165345663167344,
0.185));
#47930=CARTESIAN_POINT('Ctrl Pts',(0.0927867759536364,-0.162299064543037,
0.188051499118462));
#47931=CARTESIAN_POINT('Ctrl Pts',(0.092,-0.159348674296337,0.191));
#47932=CARTESIAN_POINT('Origin',(0.111062177826491,-0.178365334794732,0.04));
#47933=CARTESIAN_POINT('',(0.0963939408860592,-0.163732123178242,0.185));
#47934=CARTESIAN_POINT('',(0.0963939408860592,-0.163732123178242,0.0925));
#47935=CARTESIAN_POINT('Ctrl Pts',(0.092,-0.159348674296337,0.191));
#47936=CARTESIAN_POINT('Ctrl Pts',(0.0941617249279249,-0.161505237382646,
0.18805149911843));
#47937=CARTESIAN_POINT('Ctrl Pts',(0.0963939408860592,-0.163732123178242,
0.185));
#47938=CARTESIAN_POINT('Origin',(0.0673779682351567,-0.185119446294824,
0.04));
#47939=CARTESIAN_POINT('',(0.0664977155125524,-0.17798329649608,0.04));
#47940=CARTESIAN_POINT('',(0.0634652522703484,-0.179087022852749,0.04));
#47941=CARTESIAN_POINT('Origin',(0.,0.,0.04));
#47942=CARTESIAN_POINT('',(0.062931706371923,-0.172903442224607,0.04));
#47943=CARTESIAN_POINT('',(0.0784020784438917,-0.194941309361761,0.04));
#47944=CARTESIAN_POINT('',(0.062931706371923,-0.172903442224607,0.04));
#47945=CARTESIAN_POINT('Origin',(0.062931706371923,-0.172903442224607,0.04));
#47946=CARTESIAN_POINT('',(0.0634652522703484,-0.179087022852749,0.185));
#47947=CARTESIAN_POINT('',(0.0634652522703484,-0.179087022852749,0.0925));
#47948=CARTESIAN_POINT('',(0.062931706371923,-0.172903442224607,0.191));
#47949=CARTESIAN_POINT('',(0.062931706371923,-0.172903442224607,0.04));
#47950=CARTESIAN_POINT('Ctrl Pts',(0.0634652522703485,-0.179087022852749,
0.185));
#47951=CARTESIAN_POINT('Ctrl Pts',(0.0631941995412026,-0.175945631624558,
0.188051499118454));
#47952=CARTESIAN_POINT('Ctrl Pts',(0.062931706371923,-0.172903442224607,
0.191));
#47953=CARTESIAN_POINT('Origin',(0.0784020784438917,-0.194941309361761,
0.04));
#47954=CARTESIAN_POINT('',(0.0664977155125524,-0.17798329649608,0.185));
#47955=CARTESIAN_POINT('',(0.0664977155125524,-0.17798329649608,0.0925));
#47956=CARTESIAN_POINT('Ctrl Pts',(0.062931706371923,-0.172903442224607,
0.191));
#47957=CARTESIAN_POINT('Ctrl Pts',(0.0646861065908383,-0.175402621866182,
0.18805149911847));
#47958=CARTESIAN_POINT('Ctrl Pts',(0.0664977155125524,-0.17798329649608,
0.185));
#47959=CARTESIAN_POINT('Origin',(0.0342086910003852,-0.194007127343405,
0.04));
#47960=CARTESIAN_POINT('',(0.0345809907026645,-0.186826537413779,0.04));
#47961=CARTESIAN_POINT('',(0.031402937320539,-0.18738691397118,0.04));
#47962=CARTESIAN_POINT('Origin',(0.,0.,0.04));
#47963=CARTESIAN_POINT('',(0.0319512646907151,-0.181204626554246,0.04));
#47964=CARTESIAN_POINT('',(0.0433597715811408,-0.205594090888895,0.04));
#47965=CARTESIAN_POINT('',(0.0319512646907151,-0.181204626554246,0.04));
#47966=CARTESIAN_POINT('Origin',(0.0319512646907151,-0.181204626554246,
0.04));
#47967=CARTESIAN_POINT('',(0.031402937320539,-0.18738691397118,0.185));
#47968=CARTESIAN_POINT('',(0.031402937320539,-0.18738691397118,0.0925));
#47969=CARTESIAN_POINT('',(0.0319512646907151,-0.181204626554246,0.191));
#47970=CARTESIAN_POINT('',(0.0319512646907151,-0.181204626554246,0.04));
#47971=CARTESIAN_POINT('Ctrl Pts',(0.031402937320539,-0.18738691397118,
0.185));
#47972=CARTESIAN_POINT('Ctrl Pts',(0.0316814993535159,-0.184246179721939,
0.18805149911846));
#47973=CARTESIAN_POINT('Ctrl Pts',(0.0319512646907151,-0.181204626554246,
0.191));
#47974=CARTESIAN_POINT('Origin',(0.0433597715811408,-0.205594090888895,
0.04));
#47975=CARTESIAN_POINT('',(0.0345809907026646,-0.186826537413779,0.185));
#47976=CARTESIAN_POINT('',(0.0345809907026646,-0.186826537413779,0.0925));
#47977=CARTESIAN_POINT('Ctrl Pts',(0.0319512646907151,-0.181204626554246,
0.191));
#47978=CARTESIAN_POINT('Ctrl Pts',(0.0332450336377804,-0.18397048644238,
0.188051499118441));
#47979=CARTESIAN_POINT('Ctrl Pts',(0.0345809907026645,-0.186826537413779,
0.185));
#47980=CARTESIAN_POINT('Origin',(-4.16333634234434E-17,-0.197,0.04));
#47981=CARTESIAN_POINT('',(0.00161353998910185,-0.18999314853095,0.04));
#47982=CARTESIAN_POINT('',(-0.00161353998910192,-0.18999314853095,0.04));
#47983=CARTESIAN_POINT('Origin',(0.,0.,0.04));
#47984=CARTESIAN_POINT('',(-3.46944695195361E-17,-0.184,0.04));
#47985=CARTESIAN_POINT('',(0.00699999999999997,-0.21,0.04));
#47986=CARTESIAN_POINT('',(-3.46944695195361E-17,-0.184,0.04));
#47987=CARTESIAN_POINT('Origin',(-3.46944695195361E-17,-0.184,0.04));
#47988=CARTESIAN_POINT('',(-0.00161353998910191,-0.18999314853095,0.185));
#47989=CARTESIAN_POINT('',(-0.00161353998910191,-0.18999314853095,0.0925));
#47990=CARTESIAN_POINT('',(-3.46944695195361E-17,-0.184,0.191));
#47991=CARTESIAN_POINT('',(-3.46944695195361E-17,-0.184,0.04));
#47992=CARTESIAN_POINT('Ctrl Pts',(-0.0016135399891019,-0.18999314853095,
0.185));
#47993=CARTESIAN_POINT('Ctrl Pts',(-0.000793827160417415,-0.18694850088155,
0.18805149911845));
#47994=CARTESIAN_POINT('Ctrl Pts',(-3.46944695195361E-17,-0.184,0.191));
#47995=CARTESIAN_POINT('Origin',(0.00699999999999997,-0.21,0.04));
#47996=CARTESIAN_POINT('',(0.00161353998910184,-0.18999314853095,0.185));
#47997=CARTESIAN_POINT('',(0.00161353998910184,-0.18999314853095,0.0925));
#47998=CARTESIAN_POINT('Ctrl Pts',(-3.46944695195361E-17,-0.184,0.191));
#47999=CARTESIAN_POINT('Ctrl Pts',(0.000793827160417323,-0.18694850088155,
0.18805149911845));
#48000=CARTESIAN_POINT('Ctrl Pts',(0.00161353998910184,-0.18999314853095,
0.185));
#48001=CARTESIAN_POINT('Origin',(-0.0342086910003853,-0.194007127343405,
0.04));
#48002=CARTESIAN_POINT('',(-0.0314029373205391,-0.18738691397118,0.04));
#48003=CARTESIAN_POINT('',(-0.0345809907026646,-0.186826537413779,0.04));
#48004=CARTESIAN_POINT('Origin',(0.,0.,0.04));
#48005=CARTESIAN_POINT('',(-0.0319512646907152,-0.181204626554246,0.04));
#48006=CARTESIAN_POINT('',(-0.0295724630389699,-0.208025165376232,0.04));
#48007=CARTESIAN_POINT('',(-0.0319512646907152,-0.181204626554246,0.04));
#48008=CARTESIAN_POINT('Origin',(-0.0319512646907152,-0.181204626554246,
0.04));
#48009=CARTESIAN_POINT('',(-0.0345809907026646,-0.186826537413779,0.185));
#48010=CARTESIAN_POINT('',(-0.0345809907026646,-0.186826537413779,0.0925));
#48011=CARTESIAN_POINT('',(-0.0319512646907152,-0.181204626554246,0.191));
#48012=CARTESIAN_POINT('',(-0.0319512646907152,-0.181204626554246,0.04));
#48013=CARTESIAN_POINT('Ctrl Pts',(-0.0345809907026646,-0.186826537413779,
0.185));
#48014=CARTESIAN_POINT('Ctrl Pts',(-0.033245033637776,-0.18397048644237,
0.188051499118451));
#48015=CARTESIAN_POINT('Ctrl Pts',(-0.0319512646907152,-0.181204626554246,
0.191));
#48016=CARTESIAN_POINT('Origin',(-0.0295724630389699,-0.208025165376232,
0.04));
#48017=CARTESIAN_POINT('',(-0.0314029373205391,-0.18738691397118,0.185));
#48018=CARTESIAN_POINT('',(-0.0314029373205391,-0.18738691397118,0.0925));
#48019=CARTESIAN_POINT('Ctrl Pts',(-0.0319512646907152,-0.181204626554246,
0.191));
#48020=CARTESIAN_POINT('Ctrl Pts',(-0.0316814993535157,-0.184246179721942,
0.188051499118457));
#48021=CARTESIAN_POINT('Ctrl Pts',(-0.0314029373205391,-0.18738691397118,
0.185));
#48022=CARTESIAN_POINT('Origin',(-0.0673779682351569,-0.185119446294824,
0.04));
#48023=CARTESIAN_POINT('',(-0.0634652522703487,-0.179087022852749,0.04));
#48024=CARTESIAN_POINT('',(-0.0664977155125527,-0.17798329649608,0.04));
#48025=CARTESIAN_POINT('Origin',(0.,0.,0.04));
#48026=CARTESIAN_POINT('',(-0.0629317063719232,-0.172903442224607,0.04));
#48027=CARTESIAN_POINT('',(-0.0652463817528892,-0.19972959136832,0.04));
#48028=CARTESIAN_POINT('',(-0.0629317063719232,-0.172903442224607,0.04));
#48029=CARTESIAN_POINT('Origin',(-0.0629317063719232,-0.172903442224607,
0.04));
#48030=CARTESIAN_POINT('',(-0.0664977155125527,-0.17798329649608,0.185));
#48031=CARTESIAN_POINT('',(-0.0664977155125527,-0.17798329649608,0.0925));
#48032=CARTESIAN_POINT('',(-0.0629317063719232,-0.172903442224607,0.191));
#48033=CARTESIAN_POINT('',(-0.0629317063719232,-0.172903442224607,0.04));
#48034=CARTESIAN_POINT('Ctrl Pts',(-0.0664977155125527,-0.17798329649608,
0.185));
#48035=CARTESIAN_POINT('Ctrl Pts',(-0.0646861065908368,-0.175402621866179,
0.188051499118473));
#48036=CARTESIAN_POINT('Ctrl Pts',(-0.0629317063719232,-0.172903442224607,
0.191));
#48037=CARTESIAN_POINT('Origin',(-0.0652463817528892,-0.19972959136832,
0.04));
#48038=CARTESIAN_POINT('',(-0.0634652522703487,-0.179087022852749,0.185));
#48039=CARTESIAN_POINT('',(-0.0634652522703487,-0.179087022852749,0.0925));
#48040=CARTESIAN_POINT('Ctrl Pts',(-0.0629317063719232,-0.172903442224607,
0.191));
#48041=CARTESIAN_POINT('Ctrl Pts',(-0.0631941995412029,-0.175945631624558,
0.188051499118454));
#48042=CARTESIAN_POINT('Ctrl Pts',(-0.0634652522703487,-0.179087022852749,
0.185));
#48043=CARTESIAN_POINT('Origin',(-0.0985000000000001,-0.170607004545534,
0.04));
#48044=CARTESIAN_POINT('',(-0.0935992076448907,-0.165345663167344,0.04));
#48045=CARTESIAN_POINT('',(-0.0963939408860593,-0.163732123178242,0.04));
#48046=CARTESIAN_POINT('Origin',(0.,0.,0.04));
#48047=CARTESIAN_POINT('',(-0.0920000000000001,-0.159348674296337,0.04));
#48048=CARTESIAN_POINT('',(-0.098937822173509,-0.185365334794732,0.04));
#48049=CARTESIAN_POINT('',(-0.0920000000000001,-0.159348674296337,0.04));
#48050=CARTESIAN_POINT('Origin',(-0.0920000000000001,-0.159348674296337,
0.04));
#48051=CARTESIAN_POINT('',(-0.0963939408860593,-0.163732123178242,0.185));
#48052=CARTESIAN_POINT('',(-0.0963939408860593,-0.163732123178242,0.0925));
#48053=CARTESIAN_POINT('',(-0.0920000000000001,-0.159348674296337,0.191));
#48054=CARTESIAN_POINT('',(-0.0920000000000001,-0.159348674296337,0.04));
#48055=CARTESIAN_POINT('Ctrl Pts',(-0.0963939408860593,-0.163732123178242,
0.185));
#48056=CARTESIAN_POINT('Ctrl Pts',(-0.0941617249279212,-0.161505237382642,
0.188051499118436));
#48057=CARTESIAN_POINT('Ctrl Pts',(-0.0920000000000001,-0.159348674296337,
0.191));
#48058=CARTESIAN_POINT('Origin',(-0.098937822173509,-0.185365334794732,
0.04));
#48059=CARTESIAN_POINT('',(-0.0935992076448907,-0.165345663167344,0.185));
#48060=CARTESIAN_POINT('',(-0.0935992076448907,-0.165345663167344,0.0925));
#48061=CARTESIAN_POINT('Ctrl Pts',(-0.0920000000000001,-0.159348674296337,
0.191));
#48062=CARTESIAN_POINT('Ctrl Pts',(-0.0927867759536363,-0.162299064543036,
0.188051499118462));
#48063=CARTESIAN_POINT('Ctrl Pts',(-0.0935992076448907,-0.165345663167344,
0.185));
#48064=CARTESIAN_POINT('Origin',(-0.126629159108248,-0.150910755294439,
0.04));
#48065=CARTESIAN_POINT('',(-0.120889198458627,-0.146580359175541,0.04));
#48066=CARTESIAN_POINT('',(-0.123361285143431,-0.144506032150084,0.04));
#48067=CARTESIAN_POINT('Origin',(0.,0.,0.04));
#48068=CARTESIAN_POINT('',(-0.118272920182323,-0.140952177533892,0.04));
#48069=CARTESIAN_POINT('',(-0.12962308693234,-0.165368846322791,0.04));
#48070=CARTESIAN_POINT('',(-0.118272920182323,-0.140952177533892,0.04));
#48071=CARTESIAN_POINT('Origin',(-0.118272920182323,-0.140952177533892,
0.04));
#48072=CARTESIAN_POINT('',(-0.123361285143431,-0.144506032150084,0.185));
#48073=CARTESIAN_POINT('',(-0.123361285143431,-0.144506032150084,0.0925));
#48074=CARTESIAN_POINT('',(-0.118272920182323,-0.140952177533892,0.191));
#48075=CARTESIAN_POINT('',(-0.118272920182323,-0.140952177533892,0.04));
#48076=CARTESIAN_POINT('Ctrl Pts',(-0.123361285143431,-0.144506032150084,
0.185));
#48077=CARTESIAN_POINT('Ctrl Pts',(-0.120776286901195,-0.142700597986805,
0.188051499118418));
#48078=CARTESIAN_POINT('Ctrl Pts',(-0.118272920182323,-0.140952177533892,
0.191));
#48079=CARTESIAN_POINT('Origin',(-0.12962308693234,-0.165368846322791,0.04));
#48080=CARTESIAN_POINT('',(-0.120889198458627,-0.146580359175541,0.185));
#48081=CARTESIAN_POINT('',(-0.120889198458627,-0.146580359175541,0.0925));
#48082=CARTESIAN_POINT('Ctrl Pts',(-0.118272920182323,-0.140952177533892,
0.191));
#48083=CARTESIAN_POINT('Ctrl Pts',(-0.119560073131103,-0.143721122512692,
0.188051499118441));
#48084=CARTESIAN_POINT('Ctrl Pts',(-0.120889198458627,-0.146580359175541,
0.185));
#48085=CARTESIAN_POINT('Origin',(-0.150910755294439,-0.126629159108248,
0.04));
#48086=CARTESIAN_POINT('',(-0.144506032150084,-0.123361285143431,0.04));
#48087=CARTESIAN_POINT('',(-0.146580359175541,-0.120889198458627,0.04));
#48088=CARTESIAN_POINT('Origin',(0.,0.,0.04));
#48089=CARTESIAN_POINT('',(-0.140952177533892,-0.118272920182323,0.04));
#48090=CARTESIAN_POINT('',(-0.15636981978718,-0.140347709136006,0.04));
#48091=CARTESIAN_POINT('',(-0.140952177533892,-0.118272920182323,0.04));
#48092=CARTESIAN_POINT('Origin',(-0.140952177533892,-0.118272920182323,
0.04));
#48093=CARTESIAN_POINT('',(-0.146580359175541,-0.120889198458627,0.185));
#48094=CARTESIAN_POINT('',(-0.146580359175541,-0.120889198458627,0.0925));
#48095=CARTESIAN_POINT('',(-0.140952177533892,-0.118272920182323,0.191));
#48096=CARTESIAN_POINT('',(-0.140952177533892,-0.118272920182323,0.04));
#48097=CARTESIAN_POINT('Ctrl Pts',(-0.146580359175541,-0.120889198458627,
0.185));
#48098=CARTESIAN_POINT('Ctrl Pts',(-0.14372112251267,-0.119560073131093,
0.188051499118464));
#48099=CARTESIAN_POINT('Ctrl Pts',(-0.140952177533892,-0.118272920182323,
0.191));
#48100=CARTESIAN_POINT('Origin',(-0.15636981978718,-0.140347709136006,0.04));
#48101=CARTESIAN_POINT('',(-0.144506032150084,-0.123361285143431,0.185));
#48102=CARTESIAN_POINT('',(-0.144506032150084,-0.123361285143431,0.0925));
#48103=CARTESIAN_POINT('Ctrl Pts',(-0.140952177533892,-0.118272920182323,
0.191));
#48104=CARTESIAN_POINT('Ctrl Pts',(-0.142700597986788,-0.120776286901171,
0.188051499118446));
#48105=CARTESIAN_POINT('Ctrl Pts',(-0.144506032150084,-0.123361285143431,
0.185));
#48106=CARTESIAN_POINT('Origin',(-0.170607004545534,-0.0985,0.04));
#48107=CARTESIAN_POINT('',(-0.163732123178242,-0.0963939408860592,0.04));
#48108=CARTESIAN_POINT('',(-0.165345663167344,-0.0935992076448906,0.04));
#48109=CARTESIAN_POINT('Origin',(0.,0.,0.04));
#48110=CARTESIAN_POINT('',(-0.159348674296337,-0.092,0.04));
#48111=CARTESIAN_POINT('',(-0.178365334794732,-0.111062177826491,0.04));
#48112=CARTESIAN_POINT('',(-0.159348674296337,-0.092,0.04));
#48113=CARTESIAN_POINT('Origin',(-0.159348674296337,-0.092,0.04));
#48114=CARTESIAN_POINT('',(-0.165345663167344,-0.0935992076448906,0.185));
#48115=CARTESIAN_POINT('',(-0.165345663167344,-0.0935992076448906,0.0925));
#48116=CARTESIAN_POINT('',(-0.159348674296337,-0.0919999999999999,0.191));
#48117=CARTESIAN_POINT('',(-0.159348674296337,-0.092,0.04));
#48118=CARTESIAN_POINT('Ctrl Pts',(-0.165345663167344,-0.0935992076448906,
0.185));
#48119=CARTESIAN_POINT('Ctrl Pts',(-0.16229906454304,-0.0927867759536372,
0.188051499118458));
#48120=CARTESIAN_POINT('Ctrl Pts',(-0.159348674296337,-0.0919999999999999,
0.191));
#48121=CARTESIAN_POINT('Origin',(-0.178365334794732,-0.111062177826491,
0.04));
#48122=CARTESIAN_POINT('',(-0.163732123178242,-0.0963939408860592,0.185));
#48123=CARTESIAN_POINT('',(-0.163732123178242,-0.0963939408860592,0.0925));
#48124=CARTESIAN_POINT('Ctrl Pts',(-0.159348674296337,-0.0919999999999999,
0.191));
#48125=CARTESIAN_POINT('Ctrl Pts',(-0.161505237382618,-0.0941617249278968,
0.188051499118469));
#48126=CARTESIAN_POINT('Ctrl Pts',(-0.163732123178242,-0.0963939408860592,
0.185));
#48127=CARTESIAN_POINT('Origin',(-0.185119446294824,-0.0673779682351567,
0.04));
#48128=CARTESIAN_POINT('',(-0.17798329649608,-0.0664977155125525,0.04));
#48129=CARTESIAN_POINT('',(-0.179087022852749,-0.0634652522703485,0.04));
#48130=CARTESIAN_POINT('Origin',(0.,0.,0.04));
#48131=CARTESIAN_POINT('',(-0.172903442224607,-0.062931706371923,0.04));
#48132=CARTESIAN_POINT('',(-0.194941309361761,-0.0784020784438918,0.04));
#48133=CARTESIAN_POINT('',(-0.172903442224607,-0.062931706371923,0.04));
#48134=CARTESIAN_POINT('Origin',(-0.172903442224607,-0.062931706371923,
0.04));
#48135=CARTESIAN_POINT('',(-0.179087022852749,-0.0634652522703485,0.185));
#48136=CARTESIAN_POINT('',(-0.179087022852749,-0.0634652522703485,0.0925));
#48137=CARTESIAN_POINT('',(-0.172903442224607,-0.062931706371923,0.191));
#48138=CARTESIAN_POINT('',(-0.172903442224607,-0.062931706371923,0.04));
#48139=CARTESIAN_POINT('Ctrl Pts',(-0.179087022852749,-0.0634652522703485,
0.185));
#48140=CARTESIAN_POINT('Ctrl Pts',(-0.175945631624537,-0.0631941995412009,
0.188051499118474));
#48141=CARTESIAN_POINT('Ctrl Pts',(-0.172903442224607,-0.062931706371923,
0.191));
#48142=CARTESIAN_POINT('Origin',(-0.194941309361761,-0.0784020784438918,
0.04));
#48143=CARTESIAN_POINT('',(-0.17798329649608,-0.0664977155125525,0.185));
#48144=CARTESIAN_POINT('',(-0.17798329649608,-0.0664977155125525,0.0925));
#48145=CARTESIAN_POINT('Ctrl Pts',(-0.172903442224607,-0.062931706371923,
0.191));
#48146=CARTESIAN_POINT('Ctrl Pts',(-0.175402621866193,-0.0646861065908464,
0.188051499118456));
#48147=CARTESIAN_POINT('Ctrl Pts',(-0.17798329649608,-0.0664977155125525,
0.185));
#48148=CARTESIAN_POINT('Origin',(-0.194007127343405,-0.0342086910003852,
0.04));
#48149=CARTESIAN_POINT('',(-0.186826537413779,-0.0345809907026646,0.04));
#48150=CARTESIAN_POINT('',(-0.18738691397118,-0.031402937320539,0.04));
#48151=CARTESIAN_POINT('Origin',(0.,0.,0.04));
#48152=CARTESIAN_POINT('',(-0.181204626554246,-0.0319512646907151,0.04));
#48153=CARTESIAN_POINT('',(-0.205594090888895,-0.0433597715811408,0.04));
#48154=CARTESIAN_POINT('',(-0.181204626554246,-0.0319512646907151,0.04));
#48155=CARTESIAN_POINT('Origin',(-0.181204626554246,-0.0319512646907151,
0.04));
#48156=CARTESIAN_POINT('',(-0.18738691397118,-0.031402937320539,0.185));
#48157=CARTESIAN_POINT('',(-0.18738691397118,-0.031402937320539,0.0925));
#48158=CARTESIAN_POINT('',(-0.181204626554246,-0.0319512646907151,0.191));
#48159=CARTESIAN_POINT('',(-0.181204626554246,-0.0319512646907151,0.04));
#48160=CARTESIAN_POINT('Ctrl Pts',(-0.18738691397118,-0.031402937320539,
0.185));
#48161=CARTESIAN_POINT('Ctrl Pts',(-0.184246179721915,-0.031681499353518,
0.188051499118483));
#48162=CARTESIAN_POINT('Ctrl Pts',(-0.181204626554246,-0.0319512646907151,
0.191));
#48163=CARTESIAN_POINT('Origin',(-0.205594090888895,-0.0433597715811408,
0.04));
#48164=CARTESIAN_POINT('',(-0.186826537413779,-0.0345809907026646,0.185));
#48165=CARTESIAN_POINT('',(-0.186826537413779,-0.0345809907026646,0.0925));
#48166=CARTESIAN_POINT('Ctrl Pts',(-0.181204626554246,-0.0319512646907151,
0.191));
#48167=CARTESIAN_POINT('Ctrl Pts',(-0.183970486442384,-0.0332450336377824,
0.188051499118436));
#48168=CARTESIAN_POINT('Ctrl Pts',(-0.186826537413779,-0.0345809907026646,
0.185));
#48169=CARTESIAN_POINT('Origin',(-0.197,2.08166817117217E-17,0.04));
#48170=CARTESIAN_POINT('',(-0.18999314853095,-0.00161353998910186,0.04));
#48171=CARTESIAN_POINT('',(-0.19,-2.32682891837997E-17,0.04));
#48172=CARTESIAN_POINT('Origin',(0.,0.,0.04));
#48173=CARTESIAN_POINT('',(-0.184,2.08166817117217E-17,0.04));
#48174=CARTESIAN_POINT('',(-0.21,-0.00699999999999998,0.04));
#48175=CARTESIAN_POINT('',(-0.18999314853095,0.0016135399891019,0.04));
#48176=CARTESIAN_POINT('',(-0.184,2.08166817117217E-17,0.04));
#48177=CARTESIAN_POINT('Origin',(0.,0.,0.04));
#48178=CARTESIAN_POINT('Origin',(-0.184,2.08166817117217E-17,0.04));
#48179=CARTESIAN_POINT('',(-0.18999314853095,0.00161353998910189,0.185));
#48180=CARTESIAN_POINT('',(-0.18999314853095,0.00161353998910189,0.0925));
#48181=CARTESIAN_POINT('',(-0.184,2.08166817117217E-17,0.191));
#48182=CARTESIAN_POINT('',(-0.184,2.08166817117217E-17,0.04));
#48183=CARTESIAN_POINT('Ctrl Pts',(-0.18999314853095,0.00161353998910189,
0.185));
#48184=CARTESIAN_POINT('Ctrl Pts',(-0.186948500881544,0.000793827160415821,
0.188051499118456));
#48185=CARTESIAN_POINT('Ctrl Pts',(-0.184,2.08166817117217E-17,0.191));
#48186=CARTESIAN_POINT('Origin',(-0.21,-0.00699999999999998,0.04));
#48187=CARTESIAN_POINT('',(-0.18999314853095,-0.00161353998910186,0.185));
#48188=CARTESIAN_POINT('',(-0.18999314853095,-0.00161353998910186,0.0925));
#48189=CARTESIAN_POINT('Ctrl Pts',(-0.184,2.08166817117217E-17,0.191));
#48190=CARTESIAN_POINT('Ctrl Pts',(-0.186948500881545,-0.000793827160416021,
0.188051499118455));
#48191=CARTESIAN_POINT('Ctrl Pts',(-0.18999314853095,-0.00161353998910185,
0.185));
#48192=CARTESIAN_POINT('Origin',(-0.194007127343405,0.0342086910003854,
0.04));
#48193=CARTESIAN_POINT('',(-0.18738691397118,0.0314029373205392,0.04));
#48194=CARTESIAN_POINT('',(-0.186826537413779,0.0345809907026647,0.04));
#48195=CARTESIAN_POINT('Origin',(0.,0.,0.04));
#48196=CARTESIAN_POINT('',(-0.181204626554246,0.0319512646907152,0.04));
#48197=CARTESIAN_POINT('',(-0.208025165376232,0.02957246303897,0.04));
#48198=CARTESIAN_POINT('',(-0.181204626554246,0.0319512646907152,0.04));
#48199=CARTESIAN_POINT('Origin',(-0.181204626554246,0.0319512646907152,
0.04));
#48200=CARTESIAN_POINT('',(-0.186826537413779,0.0345809907026647,0.185));
#48201=CARTESIAN_POINT('',(-0.186826537413779,0.0345809907026647,0.0925));
#48202=CARTESIAN_POINT('',(-0.181204626554246,0.0319512646907153,0.191));
#48203=CARTESIAN_POINT('',(-0.181204626554246,0.0319512646907152,0.04));
#48204=CARTESIAN_POINT('Ctrl Pts',(-0.186826537413779,0.0345809907026647,
0.185));
#48205=CARTESIAN_POINT('Ctrl Pts',(-0.183970486442384,0.0332450336377824,
0.188051499118436));
#48206=CARTESIAN_POINT('Ctrl Pts',(-0.181204626554246,0.0319512646907153,
0.191));
#48207=CARTESIAN_POINT('Origin',(-0.208025165376232,0.02957246303897,0.04));
#48208=CARTESIAN_POINT('',(-0.18738691397118,0.0314029373205392,0.185));
#48209=CARTESIAN_POINT('',(-0.18738691397118,0.0314029373205392,0.0925));
#48210=CARTESIAN_POINT('Ctrl Pts',(-0.181204626554246,0.0319512646907153,
0.191));
#48211=CARTESIAN_POINT('Ctrl Pts',(-0.184246179721934,0.0316814993535164,
0.188051499118464));
#48212=CARTESIAN_POINT('Ctrl Pts',(-0.18738691397118,0.0314029373205392,
0.185));
#48213=CARTESIAN_POINT('Origin',(-0.185119446294824,0.0673779682351568,
0.04));
#48214=CARTESIAN_POINT('',(-0.179087022852749,0.0634652522703486,0.04));
#48215=CARTESIAN_POINT('',(-0.17798329649608,0.0664977155125526,0.04));
#48216=CARTESIAN_POINT('Origin',(0.,0.,0.04));
#48217=CARTESIAN_POINT('',(-0.172903442224607,0.0629317063719231,0.04));
#48218=CARTESIAN_POINT('',(-0.199729591368321,0.0652463817528891,0.04));
#48219=CARTESIAN_POINT('',(-0.172903442224607,0.0629317063719231,0.04));
#48220=CARTESIAN_POINT('Origin',(-0.172903442224607,0.0629317063719231,
0.04));
#48221=CARTESIAN_POINT('',(-0.17798329649608,0.0664977155125526,0.185));
#48222=CARTESIAN_POINT('',(-0.17798329649608,0.0664977155125526,0.0925));
#48223=CARTESIAN_POINT('',(-0.172903442224607,0.0629317063719231,0.191));
#48224=CARTESIAN_POINT('',(-0.172903442224607,0.0629317063719231,0.04));
#48225=CARTESIAN_POINT('Ctrl Pts',(-0.17798329649608,0.0664977155125526,
0.185));
#48226=CARTESIAN_POINT('Ctrl Pts',(-0.175402621866187,0.0646861065908417,
0.188051499118464));
#48227=CARTESIAN_POINT('Ctrl Pts',(-0.172903442224607,0.0629317063719231,
0.191));
#48228=CARTESIAN_POINT('Origin',(-0.199729591368321,0.0652463817528891,
0.04));
#48229=CARTESIAN_POINT('',(-0.179087022852749,0.0634652522703485,0.185));
#48230=CARTESIAN_POINT('',(-0.179087022852749,0.0634652522703485,0.0925));
#48231=CARTESIAN_POINT('Ctrl Pts',(-0.172903442224607,0.0629317063719231,
0.191));
#48232=CARTESIAN_POINT('Ctrl Pts',(-0.175945631624522,0.0631941995411996,
0.188051499118489));
#48233=CARTESIAN_POINT('Ctrl Pts',(-0.179087022852749,0.0634652522703486,
0.185));
#48234=CARTESIAN_POINT('Origin',(-0.170607004545534,0.0985,0.04));
#48235=CARTESIAN_POINT('',(-0.165345663167344,0.0935992076448906,0.04));
#48236=CARTESIAN_POINT('',(-0.163732123178242,0.0963939408860592,0.04));
#48237=CARTESIAN_POINT('Origin',(0.,0.,0.04));
#48238=CARTESIAN_POINT('',(-0.159348674296337,0.092,0.04));
#48239=CARTESIAN_POINT('',(-0.185365334794732,0.098937822173509,0.04));
#48240=CARTESIAN_POINT('',(-0.159348674296337,0.092,0.04));
#48241=CARTESIAN_POINT('Origin',(-0.159348674296337,0.092,0.04));
#48242=CARTESIAN_POINT('',(-0.163732123178242,0.0963939408860592,0.185));
#48243=CARTESIAN_POINT('',(-0.163732123178242,0.0963939408860592,0.0925));
#48244=CARTESIAN_POINT('',(-0.159348674296337,0.092,0.191));
#48245=CARTESIAN_POINT('',(-0.159348674296337,0.092,0.04));
#48246=CARTESIAN_POINT('Ctrl Pts',(-0.163732123178242,0.0963939408860592,
0.185));
#48247=CARTESIAN_POINT('Ctrl Pts',(-0.161505237382624,0.0941617249279029,
0.18805149911846));
#48248=CARTESIAN_POINT('Ctrl Pts',(-0.159348674296337,0.092,0.191));
#48249=CARTESIAN_POINT('Origin',(-0.185365334794732,0.098937822173509,0.04));
#48250=CARTESIAN_POINT('',(-0.165345663167344,0.0935992076448906,0.185));
#48251=CARTESIAN_POINT('',(-0.165345663167344,0.0935992076448906,0.0925));
#48252=CARTESIAN_POINT('Ctrl Pts',(-0.159348674296337,0.092,0.191));
#48253=CARTESIAN_POINT('Ctrl Pts',(-0.162299064543065,0.0927867759536439,
0.188051499118434));
#48254=CARTESIAN_POINT('Ctrl Pts',(-0.165345663167344,0.0935992076448907,
0.185));
#48255=CARTESIAN_POINT('Origin',(-0.150910755294439,0.126629159108248,0.04));
#48256=CARTESIAN_POINT('',(-0.146580359175541,0.120889198458627,0.04));
#48257=CARTESIAN_POINT('',(-0.144506032150084,0.123361285143431,0.04));
#48258=CARTESIAN_POINT('Origin',(0.,0.,0.04));
#48259=CARTESIAN_POINT('',(-0.140952177533892,0.118272920182323,0.04));
#48260=CARTESIAN_POINT('',(-0.165368846322791,0.12962308693234,0.04));
#48261=CARTESIAN_POINT('',(-0.140952177533892,0.118272920182323,0.04));
#48262=CARTESIAN_POINT('Origin',(-0.140952177533892,0.118272920182323,0.04));
#48263=CARTESIAN_POINT('',(-0.144506032150084,0.123361285143431,0.185));
#48264=CARTESIAN_POINT('',(-0.144506032150084,0.123361285143431,0.0925));
#48265=CARTESIAN_POINT('',(-0.140952177533892,0.118272920182323,0.191));
#48266=CARTESIAN_POINT('',(-0.140952177533892,0.118272920182323,0.04));
#48267=CARTESIAN_POINT('Ctrl Pts',(-0.144506032150084,0.123361285143431,
0.185));
#48268=CARTESIAN_POINT('Ctrl Pts',(-0.142700597986805,0.120776286901195,
0.188051499118418));
#48269=CARTESIAN_POINT('Ctrl Pts',(-0.140952177533892,0.118272920182323,
0.191));
#48270=CARTESIAN_POINT('Origin',(-0.165368846322791,0.12962308693234,0.04));
#48271=CARTESIAN_POINT('',(-0.146580359175541,0.120889198458627,0.185));
#48272=CARTESIAN_POINT('',(-0.146580359175541,0.120889198458627,0.0925));
#48273=CARTESIAN_POINT('Ctrl Pts',(-0.140952177533892,0.118272920182323,
0.191));
#48274=CARTESIAN_POINT('Ctrl Pts',(-0.143721122512692,0.119560073131103,
0.188051499118441));
#48275=CARTESIAN_POINT('Ctrl Pts',(-0.146580359175541,0.120889198458627,
0.185));
#48276=CARTESIAN_POINT('Origin',(-0.126629159108248,0.150910755294439,0.04));
#48277=CARTESIAN_POINT('',(-0.123361285143431,0.144506032150084,0.04));
#48278=CARTESIAN_POINT('',(-0.120889198458627,0.146580359175541,0.04));
#48279=CARTESIAN_POINT('Origin',(0.,0.,0.04));
#48280=CARTESIAN_POINT('',(-0.118272920182323,0.140952177533892,0.04));
#48281=CARTESIAN_POINT('',(-0.140347709136006,0.15636981978718,0.04));
#48282=CARTESIAN_POINT('',(-0.118272920182323,0.140952177533892,0.04));
#48283=CARTESIAN_POINT('Origin',(-0.118272920182323,0.140952177533892,0.04));
#48284=CARTESIAN_POINT('',(-0.120889198458627,0.146580359175541,0.185));
#48285=CARTESIAN_POINT('',(-0.120889198458627,0.146580359175541,0.0925));
#48286=CARTESIAN_POINT('',(-0.118272920182323,0.140952177533892,0.191));
#48287=CARTESIAN_POINT('',(-0.118272920182323,0.140952177533892,0.04));
#48288=CARTESIAN_POINT('Ctrl Pts',(-0.120889198458627,0.146580359175541,
0.185));
#48289=CARTESIAN_POINT('Ctrl Pts',(-0.1195600731311,0.143721122512687,0.188051499118446));
#48290=CARTESIAN_POINT('Ctrl Pts',(-0.118272920182323,0.140952177533892,
0.191));
#48291=CARTESIAN_POINT('Origin',(-0.140347709136006,0.15636981978718,0.04));
#48292=CARTESIAN_POINT('',(-0.123361285143431,0.144506032150084,0.185));
#48293=CARTESIAN_POINT('',(-0.123361285143431,0.144506032150084,0.0925));
#48294=CARTESIAN_POINT('Ctrl Pts',(-0.118272920182323,0.140952177533892,
0.191));
#48295=CARTESIAN_POINT('Ctrl Pts',(-0.120776286901187,0.142700597986799,
0.188051499118427));
#48296=CARTESIAN_POINT('Ctrl Pts',(-0.123361285143431,0.144506032150084,
0.185));
#48297=CARTESIAN_POINT('Origin',(-0.0985,0.170607004545534,0.04));
#48298=CARTESIAN_POINT('',(-0.0963939408860591,0.163732123178242,0.04));
#48299=CARTESIAN_POINT('',(-0.0935992076448906,0.165345663167344,0.04));
#48300=CARTESIAN_POINT('Origin',(0.,0.,0.04));
#48301=CARTESIAN_POINT('',(-0.092,0.159348674296337,0.04));
#48302=CARTESIAN_POINT('',(-0.111062177826491,0.178365334794732,0.04));
#48303=CARTESIAN_POINT('',(-0.092,0.159348674296337,0.04));
#48304=CARTESIAN_POINT('Origin',(-0.092,0.159348674296337,0.04));
#48305=CARTESIAN_POINT('',(-0.0935992076448906,0.165345663167344,0.185));
#48306=CARTESIAN_POINT('',(-0.0935992076448906,0.165345663167344,0.0925));
#48307=CARTESIAN_POINT('',(-0.092,0.159348674296337,0.191));
#48308=CARTESIAN_POINT('',(-0.092,0.159348674296337,0.04));
#48309=CARTESIAN_POINT('Ctrl Pts',(-0.0935992076448906,0.165345663167344,
0.185));
#48310=CARTESIAN_POINT('Ctrl Pts',(-0.0927867759536353,0.162299064543033,
0.188051499118466));
#48311=CARTESIAN_POINT('Ctrl Pts',(-0.092,0.159348674296337,0.191));
#48312=CARTESIAN_POINT('Origin',(-0.111062177826491,0.178365334794732,0.04));
#48313=CARTESIAN_POINT('',(-0.0963939408860592,0.163732123178242,0.185));
#48314=CARTESIAN_POINT('',(-0.0963939408860592,0.163732123178242,0.0925));
#48315=CARTESIAN_POINT('Ctrl Pts',(-0.092,0.159348674296337,0.191));
#48316=CARTESIAN_POINT('Ctrl Pts',(-0.0941617249279073,0.161505237382628,
0.188051499118454));
#48317=CARTESIAN_POINT('Ctrl Pts',(-0.0963939408860592,0.163732123178242,
0.185));
#48318=CARTESIAN_POINT('Origin',(-0.0673779682351567,0.185119446294824,
0.04));
#48319=CARTESIAN_POINT('',(-0.0664977155125525,0.17798329649608,0.04));
#48320=CARTESIAN_POINT('',(-0.0634652522703485,0.179087022852749,0.04));
#48321=CARTESIAN_POINT('Origin',(0.,0.,0.04));
#48322=CARTESIAN_POINT('',(-0.062931706371923,0.172903442224607,0.04));
#48323=CARTESIAN_POINT('',(-0.0784020784438918,0.194941309361761,0.04));
#48324=CARTESIAN_POINT('',(-0.062931706371923,0.172903442224607,0.04));
#48325=CARTESIAN_POINT('Origin',(-0.062931706371923,0.172903442224607,0.04));
#48326=CARTESIAN_POINT('',(-0.0634652522703485,0.179087022852749,0.185));
#48327=CARTESIAN_POINT('',(-0.0634652522703485,0.179087022852749,0.0925));
#48328=CARTESIAN_POINT('',(-0.062931706371923,0.172903442224607,0.191));
#48329=CARTESIAN_POINT('',(-0.062931706371923,0.172903442224607,0.04));
#48330=CARTESIAN_POINT('Ctrl Pts',(-0.0634652522703485,0.179087022852749,
0.185));
#48331=CARTESIAN_POINT('Ctrl Pts',(-0.0631941995412009,0.175945631624537,
0.188051499118474));
#48332=CARTESIAN_POINT('Ctrl Pts',(-0.062931706371923,0.172903442224607,
0.191));
#48333=CARTESIAN_POINT('Origin',(-0.0784020784438918,0.194941309361761,
0.04));
#48334=CARTESIAN_POINT('',(-0.0664977155125525,0.17798329649608,0.185));
#48335=CARTESIAN_POINT('',(-0.0664977155125525,0.17798329649608,0.0925));
#48336=CARTESIAN_POINT('Ctrl Pts',(-0.062931706371923,0.172903442224607,
0.191));
#48337=CARTESIAN_POINT('Ctrl Pts',(-0.0646861065908464,0.175402621866193,
0.188051499118456));
#48338=CARTESIAN_POINT('Ctrl Pts',(-0.0664977155125525,0.17798329649608,
0.185));
#48339=CARTESIAN_POINT('Origin',(-0.0342086910003853,0.194007127343405,
0.04));
#48340=CARTESIAN_POINT('',(-0.0345809907026646,0.186826537413779,0.04));
#48341=CARTESIAN_POINT('',(-0.0314029373205391,0.18738691397118,0.04));
#48342=CARTESIAN_POINT('Origin',(0.,0.,0.04));
#48343=CARTESIAN_POINT('',(-0.0319512646907152,0.181204626554246,0.04));
#48344=CARTESIAN_POINT('',(-0.0433597715811408,0.205594090888895,0.04));
#48345=CARTESIAN_POINT('',(-0.0319512646907152,0.181204626554246,0.04));
#48346=CARTESIAN_POINT('Origin',(-0.0319512646907152,0.181204626554246,
0.04));
#48347=CARTESIAN_POINT('',(-0.0314029373205391,0.18738691397118,0.185));
#48348=CARTESIAN_POINT('',(-0.0314029373205391,0.18738691397118,0.0925));
#48349=CARTESIAN_POINT('',(-0.0319512646907152,0.181204626554246,0.191));
#48350=CARTESIAN_POINT('',(-0.0319512646907152,0.181204626554246,0.04));
#48351=CARTESIAN_POINT('Ctrl Pts',(-0.0314029373205391,0.18738691397118,
0.185));
#48352=CARTESIAN_POINT('Ctrl Pts',(-0.031681499353516,0.184246179721939,
0.18805149911846));
#48353=CARTESIAN_POINT('Ctrl Pts',(-0.0319512646907152,0.181204626554246,
0.191));
#48354=CARTESIAN_POINT('Origin',(-0.0433597715811408,0.205594090888895,
0.04));
#48355=CARTESIAN_POINT('',(-0.0345809907026646,0.186826537413779,0.185));
#48356=CARTESIAN_POINT('',(-0.0345809907026646,0.186826537413779,0.0925));
#48357=CARTESIAN_POINT('Ctrl Pts',(-0.0319512646907152,0.181204626554246,
0.191));
#48358=CARTESIAN_POINT('Ctrl Pts',(-0.033245033637777,0.183970486442373,
0.188051499118448));
#48359=CARTESIAN_POINT('Ctrl Pts',(-0.0345809907026646,0.186826537413779,
0.185));
#48360=CARTESIAN_POINT('Origin',(1.38777878078145E-17,0.197,0.04));
#48361=CARTESIAN_POINT('',(-0.00161353998910187,0.18999314853095,0.04));
#48362=CARTESIAN_POINT('',(0.00161353998910189,0.18999314853095,0.04));
#48363=CARTESIAN_POINT('Origin',(0.,0.,0.04));
#48364=CARTESIAN_POINT('',(6.93889390390723E-18,0.184,0.04));
#48365=CARTESIAN_POINT('',(-0.00699999999999999,0.21,0.04));
#48366=CARTESIAN_POINT('',(6.93889390390723E-18,0.184,0.04));
#48367=CARTESIAN_POINT('Origin',(6.93889390390723E-18,0.184,0.04));
#48368=CARTESIAN_POINT('',(0.00161353998910188,0.18999314853095,0.185));
#48369=CARTESIAN_POINT('',(0.00161353998910188,0.18999314853095,0.0925));
#48370=CARTESIAN_POINT('',(6.93889390390723E-18,0.184,0.191));
#48371=CARTESIAN_POINT('',(6.93889390390723E-18,0.184,0.04));
#48372=CARTESIAN_POINT('Ctrl Pts',(0.00161353998910188,0.18999314853095,
0.185));
#48373=CARTESIAN_POINT('Ctrl Pts',(0.000793827160417808,0.186948500881552,
0.188051499118448));
#48374=CARTESIAN_POINT('Ctrl Pts',(6.93889390390723E-18,0.184,0.191));
#48375=CARTESIAN_POINT('Origin',(-0.00699999999999999,0.21,0.04));
#48376=CARTESIAN_POINT('',(-0.00161353998910187,0.18999314853095,0.185));
#48377=CARTESIAN_POINT('',(-0.00161353998910187,0.18999314853095,0.0925));
#48378=CARTESIAN_POINT('Ctrl Pts',(6.93889390390723E-18,0.184,0.191));
#48379=CARTESIAN_POINT('Ctrl Pts',(-0.000793827160415599,0.186948500881544,
0.188051499118456));
#48380=CARTESIAN_POINT('Ctrl Pts',(-0.00161353998910187,0.18999314853095,
0.185));
#48381=CARTESIAN_POINT('Origin',(0.0342086910003853,0.194007127343405,0.04));
#48382=CARTESIAN_POINT('',(0.0314029373205391,0.18738691397118,0.04));
#48383=CARTESIAN_POINT('',(0.0345809907026646,0.186826537413779,0.04));
#48384=CARTESIAN_POINT('Origin',(0.,0.,0.04));
#48385=CARTESIAN_POINT('',(0.0319512646907152,0.181204626554246,0.04));
#48386=CARTESIAN_POINT('',(0.02957246303897,0.208025165376232,0.04));
#48387=CARTESIAN_POINT('',(0.0319512646907152,0.181204626554246,0.04));
#48388=CARTESIAN_POINT('Origin',(0.0319512646907152,0.181204626554246,0.04));
#48389=CARTESIAN_POINT('',(0.0345809907026646,0.186826537413779,0.185));
#48390=CARTESIAN_POINT('',(0.0345809907026646,0.186826537413779,0.0925));
#48391=CARTESIAN_POINT('',(0.0319512646907152,0.181204626554246,0.191));
#48392=CARTESIAN_POINT('',(0.0319512646907152,0.181204626554246,0.04));
#48393=CARTESIAN_POINT('Ctrl Pts',(0.0345809907026646,0.186826537413779,
0.185));
#48394=CARTESIAN_POINT('Ctrl Pts',(0.0332450336377822,0.183970486442384,
0.188051499118437));
#48395=CARTESIAN_POINT('Ctrl Pts',(0.0319512646907152,0.181204626554246,
0.191));
#48396=CARTESIAN_POINT('Origin',(0.02957246303897,0.208025165376232,0.04));
#48397=CARTESIAN_POINT('',(0.0314029373205391,0.18738691397118,0.185));
#48398=CARTESIAN_POINT('',(0.0314029373205391,0.18738691397118,0.0925));
#48399=CARTESIAN_POINT('Ctrl Pts',(0.0319512646907152,0.181204626554246,
0.191));
#48400=CARTESIAN_POINT('Ctrl Pts',(0.0316814993535166,0.184246179721932,
0.188051499118467));
#48401=CARTESIAN_POINT('Ctrl Pts',(0.0314029373205392,0.18738691397118,
0.185));
#48402=CARTESIAN_POINT('Origin',(0.0673779682351568,0.185119446294824,0.04));
#48403=CARTESIAN_POINT('',(0.0634652522703486,0.179087022852749,0.04));
#48404=CARTESIAN_POINT('',(0.0664977155125526,0.17798329649608,0.04));
#48405=CARTESIAN_POINT('Origin',(0.,0.,0.04));
#48406=CARTESIAN_POINT('',(0.0629317063719231,0.172903442224607,0.04));
#48407=CARTESIAN_POINT('',(0.0652463817528891,0.199729591368321,0.04));
#48408=CARTESIAN_POINT('',(0.0629317063719231,0.172903442224607,0.04));
#48409=CARTESIAN_POINT('Origin',(0.0629317063719231,0.172903442224607,0.04));
#48410=CARTESIAN_POINT('',(0.0664977155125526,0.17798329649608,0.185));
#48411=CARTESIAN_POINT('',(0.0664977155125526,0.17798329649608,0.0925));
#48412=CARTESIAN_POINT('',(0.0629317063719231,0.172903442224607,0.191));
#48413=CARTESIAN_POINT('',(0.0629317063719231,0.172903442224607,0.04));
#48414=CARTESIAN_POINT('Ctrl Pts',(0.0664977155125526,0.17798329649608,
0.185));
#48415=CARTESIAN_POINT('Ctrl Pts',(0.0646861065908417,0.175402621866187,
0.188051499118464));
#48416=CARTESIAN_POINT('Ctrl Pts',(0.0629317063719231,0.172903442224607,
0.191));
#48417=CARTESIAN_POINT('Origin',(0.0652463817528891,0.199729591368321,0.04));
#48418=CARTESIAN_POINT('',(0.0634652522703485,0.179087022852749,0.185));
#48419=CARTESIAN_POINT('',(0.0634652522703485,0.179087022852749,0.0925));
#48420=CARTESIAN_POINT('Ctrl Pts',(0.0629317063719231,0.172903442224607,
0.191));
#48421=CARTESIAN_POINT('Ctrl Pts',(0.0631941995411996,0.175945631624522,
0.188051499118489));
#48422=CARTESIAN_POINT('Ctrl Pts',(0.0634652522703486,0.179087022852749,
0.185));
#48423=CARTESIAN_POINT('Origin',(0.0985,0.170607004545534,0.04));
#48424=CARTESIAN_POINT('',(0.0935992076448906,0.165345663167344,0.04));
#48425=CARTESIAN_POINT('',(0.0963939408860592,0.163732123178242,0.04));
#48426=CARTESIAN_POINT('Origin',(0.,0.,0.04));
#48427=CARTESIAN_POINT('',(0.092,0.159348674296337,0.04));
#48428=CARTESIAN_POINT('',(0.098937822173509,0.185365334794732,0.04));
#48429=CARTESIAN_POINT('',(0.092,0.159348674296337,0.04));
#48430=CARTESIAN_POINT('Origin',(0.092,0.159348674296337,0.04));
#48431=CARTESIAN_POINT('',(0.0963939408860592,0.163732123178242,0.185));
#48432=CARTESIAN_POINT('',(0.0963939408860592,0.163732123178242,0.0925));
#48433=CARTESIAN_POINT('',(0.092,0.159348674296337,0.191));
#48434=CARTESIAN_POINT('',(0.092,0.159348674296337,0.04));
#48435=CARTESIAN_POINT('Ctrl Pts',(0.0963939408860592,0.163732123178242,
0.185));
#48436=CARTESIAN_POINT('Ctrl Pts',(0.0941617249279218,0.161505237382642,
0.188051499118435));
#48437=CARTESIAN_POINT('Ctrl Pts',(0.092,0.159348674296337,0.191));
#48438=CARTESIAN_POINT('Origin',(0.098937822173509,0.185365334794732,0.04));
#48439=CARTESIAN_POINT('',(0.0935992076448906,0.165345663167344,0.185));
#48440=CARTESIAN_POINT('',(0.0935992076448906,0.165345663167344,0.0925));
#48441=CARTESIAN_POINT('Ctrl Pts',(0.092,0.159348674296337,0.191));
#48442=CARTESIAN_POINT('Ctrl Pts',(0.0927867759536358,0.162299064543034,
0.188051499118464));
#48443=CARTESIAN_POINT('Ctrl Pts',(0.0935992076448907,0.165345663167344,
0.185));
#48444=CARTESIAN_POINT('Origin',(0.126629159108248,0.150910755294439,0.04));
#48445=CARTESIAN_POINT('',(0.120889198458627,0.146580359175541,0.04));
#48446=CARTESIAN_POINT('',(0.123361285143431,0.144506032150084,0.04));
#48447=CARTESIAN_POINT('Origin',(0.,0.,0.04));
#48448=CARTESIAN_POINT('',(0.118272920182323,0.140952177533892,0.04));
#48449=CARTESIAN_POINT('',(0.12962308693234,0.165368846322791,0.04));
#48450=CARTESIAN_POINT('',(0.118272920182323,0.140952177533892,0.04));
#48451=CARTESIAN_POINT('Origin',(0.118272920182323,0.140952177533892,0.04));
#48452=CARTESIAN_POINT('',(0.123361285143431,0.144506032150084,0.185));
#48453=CARTESIAN_POINT('',(0.123361285143431,0.144506032150084,0.0925));
#48454=CARTESIAN_POINT('',(0.118272920182323,0.140952177533892,0.191));
#48455=CARTESIAN_POINT('',(0.118272920182323,0.140952177533892,0.04));
#48456=CARTESIAN_POINT('Ctrl Pts',(0.123361285143431,0.144506032150084,
0.185));
#48457=CARTESIAN_POINT('Ctrl Pts',(0.120776286901163,0.142700597986783,
0.188051499118455));
#48458=CARTESIAN_POINT('Ctrl Pts',(0.118272920182323,0.140952177533892,
0.191));
#48459=CARTESIAN_POINT('Origin',(0.12962308693234,0.165368846322791,0.04));
#48460=CARTESIAN_POINT('',(0.120889198458627,0.146580359175541,0.185));
#48461=CARTESIAN_POINT('',(0.120889198458627,0.146580359175541,0.0925));
#48462=CARTESIAN_POINT('Ctrl Pts',(0.118272920182323,0.140952177533892,
0.191));
#48463=CARTESIAN_POINT('Ctrl Pts',(0.119560073131097,0.14372112251268,0.188051499118454));
#48464=CARTESIAN_POINT('Ctrl Pts',(0.120889198458627,0.146580359175541,
0.185));
#48465=CARTESIAN_POINT('Origin',(0.150910755294439,0.126629159108248,0.04));
#48466=CARTESIAN_POINT('',(0.144506032150084,0.123361285143431,0.04));
#48467=CARTESIAN_POINT('',(0.146580359175541,0.120889198458627,0.04));
#48468=CARTESIAN_POINT('Origin',(0.,0.,0.04));
#48469=CARTESIAN_POINT('',(0.140952177533892,0.118272920182323,0.04));
#48470=CARTESIAN_POINT('',(0.15636981978718,0.140347709136006,0.04));
#48471=CARTESIAN_POINT('',(0.140952177533892,0.118272920182323,0.04));
#48472=CARTESIAN_POINT('Origin',(0.140952177533892,0.118272920182323,0.04));
#48473=CARTESIAN_POINT('',(0.146580359175541,0.120889198458627,0.185));
#48474=CARTESIAN_POINT('',(0.146580359175541,0.120889198458627,0.0925));
#48475=CARTESIAN_POINT('',(0.140952177533892,0.118272920182323,0.191));
#48476=CARTESIAN_POINT('',(0.140952177533892,0.118272920182323,0.04));
#48477=CARTESIAN_POINT('Ctrl Pts',(0.146580359175541,0.120889198458627,
0.185));
#48478=CARTESIAN_POINT('Ctrl Pts',(0.14372112251267,0.119560073131093,0.188051499118464));
#48479=CARTESIAN_POINT('Ctrl Pts',(0.140952177533892,0.118272920182323,
0.191));
#48480=CARTESIAN_POINT('Origin',(0.15636981978718,0.140347709136006,0.04));
#48481=CARTESIAN_POINT('',(0.144506032150084,0.123361285143431,0.185));
#48482=CARTESIAN_POINT('',(0.144506032150084,0.123361285143431,0.0925));
#48483=CARTESIAN_POINT('Ctrl Pts',(0.140952177533892,0.118272920182323,
0.191));
#48484=CARTESIAN_POINT('Ctrl Pts',(0.142700597986788,0.120776286901171,
0.188051499118446));
#48485=CARTESIAN_POINT('Ctrl Pts',(0.144506032150084,0.123361285143431,
0.185));
#48486=CARTESIAN_POINT('Origin',(0.170607004545534,0.0985,0.04));
#48487=CARTESIAN_POINT('',(0.163732123178242,0.0963939408860592,0.04));
#48488=CARTESIAN_POINT('',(0.165345663167344,0.0935992076448906,0.04));
#48489=CARTESIAN_POINT('Origin',(0.,0.,0.04));
#48490=CARTESIAN_POINT('',(0.159348674296337,0.092,0.04));
#48491=CARTESIAN_POINT('',(0.178365334794732,0.111062177826491,0.04));
#48492=CARTESIAN_POINT('',(0.159348674296337,0.092,0.04));
#48493=CARTESIAN_POINT('Origin',(0.159348674296337,0.092,0.04));
#48494=CARTESIAN_POINT('',(0.165345663167344,0.0935992076448906,0.185));
#48495=CARTESIAN_POINT('',(0.165345663167344,0.0935992076448906,0.0925));
#48496=CARTESIAN_POINT('',(0.159348674296337,0.092,0.191));
#48497=CARTESIAN_POINT('',(0.159348674296337,0.092,0.04));
#48498=CARTESIAN_POINT('Ctrl Pts',(0.165345663167344,0.0935992076448906,
0.185));
#48499=CARTESIAN_POINT('Ctrl Pts',(0.162299064543034,0.0927867759536356,
0.188051499118465));
#48500=CARTESIAN_POINT('Ctrl Pts',(0.159348674296337,0.092,0.191));
#48501=CARTESIAN_POINT('Origin',(0.178365334794732,0.111062177826491,0.04));
#48502=CARTESIAN_POINT('',(0.163732123178242,0.0963939408860592,0.185));
#48503=CARTESIAN_POINT('',(0.163732123178242,0.0963939408860592,0.0925));
#48504=CARTESIAN_POINT('Ctrl Pts',(0.159348674296337,0.092,0.191));
#48505=CARTESIAN_POINT('Ctrl Pts',(0.161505237382625,0.0941617249279039,
0.188051499118459));
#48506=CARTESIAN_POINT('Ctrl Pts',(0.163732123178242,0.0963939408860592,
0.185));
#48507=CARTESIAN_POINT('Origin',(0.185119446294824,0.0673779682351567,0.04));
#48508=CARTESIAN_POINT('',(0.17798329649608,0.0664977155125525,0.04));
#48509=CARTESIAN_POINT('',(0.179087022852749,0.0634652522703485,0.04));
#48510=CARTESIAN_POINT('Origin',(0.,0.,0.04));
#48511=CARTESIAN_POINT('',(0.172903442224607,0.062931706371923,0.04));
#48512=CARTESIAN_POINT('',(0.194941309361761,0.0784020784438918,0.04));
#48513=CARTESIAN_POINT('',(0.172903442224607,0.062931706371923,0.04));
#48514=CARTESIAN_POINT('Origin',(0.172903442224607,0.062931706371923,0.04));
#48515=CARTESIAN_POINT('',(0.179087022852749,0.0634652522703485,0.185));
#48516=CARTESIAN_POINT('',(0.179087022852749,0.0634652522703485,0.0925));
#48517=CARTESIAN_POINT('',(0.172903442224607,0.062931706371923,0.191));
#48518=CARTESIAN_POINT('',(0.172903442224607,0.062931706371923,0.04));
#48519=CARTESIAN_POINT('Ctrl Pts',(0.179087022852749,0.0634652522703485,
0.185));
#48520=CARTESIAN_POINT('Ctrl Pts',(0.175945631624537,0.0631941995412009,
0.188051499118474));
#48521=CARTESIAN_POINT('Ctrl Pts',(0.172903442224607,0.062931706371923,
0.191));
#48522=CARTESIAN_POINT('Origin',(0.194941309361761,0.0784020784438918,0.04));
#48523=CARTESIAN_POINT('',(0.17798329649608,0.0664977155125525,0.185));
#48524=CARTESIAN_POINT('',(0.17798329649608,0.0664977155125525,0.0925));
#48525=CARTESIAN_POINT('Ctrl Pts',(0.172903442224607,0.062931706371923,
0.191));
#48526=CARTESIAN_POINT('Ctrl Pts',(0.175402621866193,0.0646861065908464,
0.188051499118456));
#48527=CARTESIAN_POINT('Ctrl Pts',(0.17798329649608,0.0664977155125525,
0.185));
#48528=CARTESIAN_POINT('Origin',(0.194007127343405,0.0342086910003853,0.04));
#48529=CARTESIAN_POINT('',(0.186826537413779,0.0345809907026646,0.04));
#48530=CARTESIAN_POINT('',(0.18738691397118,0.0314029373205391,0.04));
#48531=CARTESIAN_POINT('Origin',(0.,0.,0.04));
#48532=CARTESIAN_POINT('',(0.181204626554246,0.0319512646907152,0.04));
#48533=CARTESIAN_POINT('',(0.205594090888895,0.0433597715811408,0.04));
#48534=CARTESIAN_POINT('',(0.181204626554246,0.0319512646907152,0.04));
#48535=CARTESIAN_POINT('Origin',(0.181204626554246,0.0319512646907152,0.04));
#48536=CARTESIAN_POINT('',(0.18738691397118,0.0314029373205391,0.185));
#48537=CARTESIAN_POINT('',(0.18738691397118,0.0314029373205391,0.0925));
#48538=CARTESIAN_POINT('',(0.181204626554246,0.0319512646907152,0.191));
#48539=CARTESIAN_POINT('',(0.181204626554246,0.0319512646907152,0.04));
#48540=CARTESIAN_POINT('Ctrl Pts',(0.18738691397118,0.0314029373205391,
0.185));
#48541=CARTESIAN_POINT('Ctrl Pts',(0.184246179721932,0.0316814993535165,
0.188051499118466));
#48542=CARTESIAN_POINT('Ctrl Pts',(0.181204626554246,0.0319512646907152,
0.191));
#48543=CARTESIAN_POINT('Origin',(0.205594090888895,0.0433597715811408,0.04));
#48544=CARTESIAN_POINT('',(0.186826537413779,0.0345809907026646,0.185));
#48545=CARTESIAN_POINT('',(0.186826537413779,0.0345809907026646,0.0925));
#48546=CARTESIAN_POINT('Ctrl Pts',(0.181204626554246,0.0319512646907152,
0.191));
#48547=CARTESIAN_POINT('Ctrl Pts',(0.183970486442399,0.0332450336377893,
0.18805149911842));
#48548=CARTESIAN_POINT('Ctrl Pts',(0.186826537413779,0.0345809907026646,
0.185));
#48549=CARTESIAN_POINT('Origin',(0.,0.,0.0925));
#48550=CARTESIAN_POINT('Origin',(0.,0.,0.185));
#48551=CARTESIAN_POINT('Origin',(0.,0.,0.185));
#48552=CARTESIAN_POINT('Origin',(0.,0.,0.185));
#48553=CARTESIAN_POINT('Origin',(0.,0.,0.185));
#48554=CARTESIAN_POINT('Origin',(0.,0.,0.185));
#48555=CARTESIAN_POINT('Origin',(0.,0.,0.185));
#48556=CARTESIAN_POINT('Origin',(0.,0.,0.185));
#48557=CARTESIAN_POINT('Origin',(0.,0.,0.185));
#48558=CARTESIAN_POINT('Origin',(0.,0.,0.185));
#48559=CARTESIAN_POINT('Origin',(0.,0.,0.185));
#48560=CARTESIAN_POINT('Origin',(0.,0.,0.185));
#48561=CARTESIAN_POINT('Origin',(0.,0.,0.185));
#48562=CARTESIAN_POINT('Origin',(0.,0.,0.185));
#48563=CARTESIAN_POINT('Origin',(0.,0.,0.185));
#48564=CARTESIAN_POINT('Origin',(0.,0.,0.185));
#48565=CARTESIAN_POINT('Origin',(0.,0.,0.185));
#48566=CARTESIAN_POINT('Origin',(0.,0.,0.185));
#48567=CARTESIAN_POINT('',(-0.19,-2.32682891837997E-17,0.));
#48568=CARTESIAN_POINT('',(-0.19,-2.32682891837997E-17,0.0925));
#48569=CARTESIAN_POINT('Origin',(0.,0.,0.));
#48570=CARTESIAN_POINT('Origin',(0.,0.,0.185));
#48571=CARTESIAN_POINT('Origin',(0.,0.,0.185));
#48572=CARTESIAN_POINT('Origin',(0.,0.,0.185));
#48573=CARTESIAN_POINT('Origin',(0.,0.,0.185));
#48574=CARTESIAN_POINT('Origin',(0.,0.,0.185));
#48575=CARTESIAN_POINT('Origin',(0.,0.,0.185));
#48576=CARTESIAN_POINT('Origin',(0.,0.,0.185));
#48577=CARTESIAN_POINT('Origin',(0.,0.,0.185));
#48578=CARTESIAN_POINT('Origin',(0.,0.,0.185));
#48579=CARTESIAN_POINT('Origin',(0.,0.,0.185));
#48580=CARTESIAN_POINT('Origin',(0.,0.,0.185));
#48581=CARTESIAN_POINT('Origin',(0.,0.,0.185));
#48582=CARTESIAN_POINT('Origin',(0.,0.,0.185));
#48583=CARTESIAN_POINT('Origin',(0.,0.,0.185));
#48584=CARTESIAN_POINT('Origin',(0.,0.,0.185));
#48585=CARTESIAN_POINT('Origin',(0.,0.,0.185));
#48586=CARTESIAN_POINT('Origin',(0.,0.,0.185));
#48587=CARTESIAN_POINT('',(0.18999314853095,0.00161353998910188,0.185));
#48588=CARTESIAN_POINT('Origin',(0.,0.,0.185));
#48589=CARTESIAN_POINT('',(0.18999314853095,0.00161353998910188,0.04));
#48590=CARTESIAN_POINT('',(0.18999314853095,0.00161353998910188,0.0925));
#48591=CARTESIAN_POINT('',(0.18999314853095,-0.00161353998910189,0.04));
#48592=CARTESIAN_POINT('Origin',(0.,0.,0.04));
#48593=CARTESIAN_POINT('',(0.18999314853095,-0.00161353998910189,0.185));
#48594=CARTESIAN_POINT('',(0.18999314853095,-0.00161353998910189,0.0925));
#48595=CARTESIAN_POINT('Origin',(0.,0.,0.185));
#48596=CARTESIAN_POINT('Origin',(0.184,0.,0.04));
#48597=CARTESIAN_POINT('',(0.184,0.,0.04));
#48598=CARTESIAN_POINT('',(0.184,0.,0.04));
#48599=CARTESIAN_POINT('',(0.184,0.,0.191));
#48600=CARTESIAN_POINT('',(0.184,0.,0.04));
#48601=CARTESIAN_POINT('Ctrl Pts',(0.18999314853095,-0.00161353998910188,
0.185));
#48602=CARTESIAN_POINT('Ctrl Pts',(0.186948500881579,-0.000793827160425129,
0.188051499118421));
#48603=CARTESIAN_POINT('Ctrl Pts',(0.184,0.,0.191));
#48604=CARTESIAN_POINT('Origin',(0.21,0.007,0.04));
#48605=CARTESIAN_POINT('Ctrl Pts',(0.184,0.,0.191));
#48606=CARTESIAN_POINT('Ctrl Pts',(0.1869485008816,0.000793827160430761,
0.1880514991184));
#48607=CARTESIAN_POINT('Ctrl Pts',(0.18999314853095,0.00161353998910188,
0.185));
#48608=CARTESIAN_POINT('',(0.21,0.007,0.04));
#48609=CARTESIAN_POINT('Origin',(0.197,0.,0.04));
#48610=CARTESIAN_POINT('Origin',(0.,0.,0.1925));
#48611=CARTESIAN_POINT('',(-0.175,-2.14313189850787E-17,0.2));
#48612=CARTESIAN_POINT('Origin',(0.,0.,0.2));
#48613=CARTESIAN_POINT('',(-0.1825,-2.23498040844392E-17,0.1925));
#48614=CARTESIAN_POINT('Origin',(0.,0.,0.078849364905389));
#48615=CARTESIAN_POINT('',(0.,0.,0.0566987298107781));
#48616=CARTESIAN_POINT('',(-0.0677181486487011,8.29308139868164E-18,0.1));
#48617=CARTESIAN_POINT('',(-0.0346410161513776,-4.24230095489963E-18,0.078849364905389));
#48618=CARTESIAN_POINT('Origin',(0.,0.,0.1));
#48619=CARTESIAN_POINT('Origin',(0.,0.0866025403784439,0.2));
#48620=CARTESIAN_POINT('',(5.30287619362453E-18,0.0866025403784439,0.2));
#48621=CARTESIAN_POINT('',(0.075,0.0433012701892219,0.2));
#48622=CARTESIAN_POINT('',(0.01875,0.0757772228311384,0.2));
#48623=CARTESIAN_POINT('',(0.,0.0866025403784439,0.1));
#48624=CARTESIAN_POINT('',(5.30287619362453E-18,0.0866025403784439,0.2));
#48625=CARTESIAN_POINT('',(0.075,0.0433012701892219,0.1));
#48626=CARTESIAN_POINT('',(0.075,0.0433012701892219,0.1));
#48627=CARTESIAN_POINT('',(0.075,0.0433012701892219,0.2));
#48628=CARTESIAN_POINT('Origin',(-0.075,0.0433012701892219,0.2));
#48629=CARTESIAN_POINT('',(-0.075,0.0433012701892219,0.2));
#48630=CARTESIAN_POINT('',(-0.05625,0.0541265877365274,0.2));
#48631=CARTESIAN_POINT('',(-0.075,0.0433012701892219,0.1));
#48632=CARTESIAN_POINT('',(-0.075,0.0433012701892219,0.2));
#48633=CARTESIAN_POINT('',(5.30287619362453E-18,0.0866025403784439,0.1));
#48634=CARTESIAN_POINT('Origin',(-0.075,-0.0433012701892219,0.2));
#48635=CARTESIAN_POINT('',(-0.075,-0.0433012701892219,0.2));
#48636=CARTESIAN_POINT('',(-0.075,-0.021650635094611,0.2));
#48637=CARTESIAN_POINT('',(-0.075,-0.0433012701892219,0.1));
#48638=CARTESIAN_POINT('',(-0.075,-0.0433012701892219,0.2));
#48639=CARTESIAN_POINT('',(-0.075,0.0433012701892219,0.1));
#48640=CARTESIAN_POINT('Origin',(-1.38777878078145E-17,-0.0866025403784439,
0.2));
#48641=CARTESIAN_POINT('',(-1.59086285808736E-17,-0.0866025403784439,0.2));
#48642=CARTESIAN_POINT('',(-0.01875,-0.0757772228311384,0.2));
#48643=CARTESIAN_POINT('',(-1.38777878078145E-17,-0.0866025403784439,0.1));
#48644=CARTESIAN_POINT('',(-1.59086285808736E-17,-0.0866025403784439,0.2));
#48645=CARTESIAN_POINT('',(-0.075,-0.0433012701892219,0.1));
#48646=CARTESIAN_POINT('Origin',(0.075,-0.043301270189222,0.2));
#48647=CARTESIAN_POINT('',(0.075,-0.043301270189222,0.2));
#48648=CARTESIAN_POINT('',(0.05625,-0.0541265877365275,0.2));
#48649=CARTESIAN_POINT('',(0.075,-0.043301270189222,0.1));
#48650=CARTESIAN_POINT('',(0.075,-0.043301270189222,0.2));
#48651=CARTESIAN_POINT('',(-1.59086285808736E-17,-0.0866025403784439,0.1));
#48652=CARTESIAN_POINT('Origin',(0.075,0.0433012701892219,0.2));
#48653=CARTESIAN_POINT('',(0.075,0.021650635094611,0.2));
#48654=CARTESIAN_POINT('',(0.075,-0.043301270189222,0.1));
#48655=CARTESIAN_POINT('Origin',(0.,0.,0.1));
#48656=CARTESIAN_POINT('Origin',(0.076,0.,-1.));
#48657=CARTESIAN_POINT('',(-0.076,-9.30731567351988E-18,-1.));
#48658=CARTESIAN_POINT('Origin',(0.,0.,-1.));
#48659=CARTESIAN_POINT('Origin',(0.,0.,-0.988));
#48660=CARTESIAN_POINT('',(-0.088,-1.07768918324967E-17,-0.988));
#48661=CARTESIAN_POINT('Origin',(0.,0.,-0.493));
#48662=CARTESIAN_POINT('Origin',(0.,0.,-0.013325));
#48663=CARTESIAN_POINT('Origin',(0.,0.,-0.005));
#48664=CARTESIAN_POINT('',(-0.11,-1.34711147906209E-17,-3.46944695195361E-18));
#48665=CARTESIAN_POINT('Origin',(0.,0.,0.));
#48666=CARTESIAN_POINT('',(-0.105,-1.28587913910472E-17,-0.005));
#48667=CARTESIAN_POINT('Origin',(0.19,0.,0.));
#48668=CARTESIAN_POINT('Origin',(0.,0.,0.2));
#54976=UNCERTAINTY_MEASURE_WITH_UNIT(LENGTH_MEASURE(0.001),#55003,
'DISTANCE_ACCURACY_VALUE',
'Maximum model space distance between geometric entities at asserted c
onnectivities');
#54980=UNCERTAINTY_MEASURE_WITH_UNIT(LENGTH_MEASURE(0.001),#55003,
'DISTANCE_ACCURACY_VALUE',
'Maximum model space distance between geometric entities at asserted c
onnectivities');
#54998=(
GEOMETRIC_REPRESENTATION_CONTEXT(3)
GLOBAL_UNCERTAINTY_ASSIGNED_CONTEXT((#54976))
GLOBAL_UNIT_ASSIGNED_CONTEXT((#55003,#55005,#55006))
REPRESENTATION_CONTEXT('','3D')
);
#55002=(
GEOMETRIC_REPRESENTATION_CONTEXT(3)
GLOBAL_UNCERTAINTY_ASSIGNED_CONTEXT((#54980))
GLOBAL_UNIT_ASSIGNED_CONTEXT((#55003,#55005,#55006))
REPRESENTATION_CONTEXT('','3D')
);
#55003=(
LENGTH_UNIT()
NAMED_UNIT(*)
SI_UNIT(.CENTI.,.METRE.)
);
#55005=(
NAMED_UNIT(*)
PLANE_ANGLE_UNIT()
SI_UNIT($,.RADIAN.)
);
#55006=(
NAMED_UNIT(*)
SI_UNIT($,.STERADIAN.)
SOLID_ANGLE_UNIT()
);
#55024=SHAPE_DEFINITION_REPRESENTATION(#55045,#55120);
#55045=PRODUCT_DEFINITION_SHAPE('',$,#55142);
#55120=SHAPE_REPRESENTATION('',(#26524),#54998);
#55124=PRODUCT_DEFINITION_CONTEXT('part definition',#55189,'design');
#55142=PRODUCT_DEFINITION('2026-10-18-23-36-55-856',
'16_ISO_4762_M2x10_A2',#55163,#55124);
#55163=PRODUCT_DEFINITION_FORMATION('',$,#55208);
#55189=APPLICATION_CONTEXT(
'Core Data for Automotive Mechanical Design Process');
#55190=PRODUCT_CONTEXT('part definition',#55189,'mechanical');
#55208=PRODUCT('2026-10-18-23-36-55-856','16_ISO_4762_M2x10_A2',$,(#55190));
#55387=COLOUR_RGB('Black',0.12,0.14,0.17);
#55388=FILL_AREA_STYLE_COLOUR('',#55387);
#55389=FILL_AREA_STYLE('',(#55388));
#55390=SURFACE_STYLE_FILL_AREA(#55389);
#55391=SURFACE_SIDE_STYLE('',(#55390));
#55392=SURFACE_STYLE_USAGE(.BOTH.,#55391);
#55393=PRESENTATION_STYLE_ASSIGNMENT((#55392));
ENDSEC;
END-ISO-10303-21;
